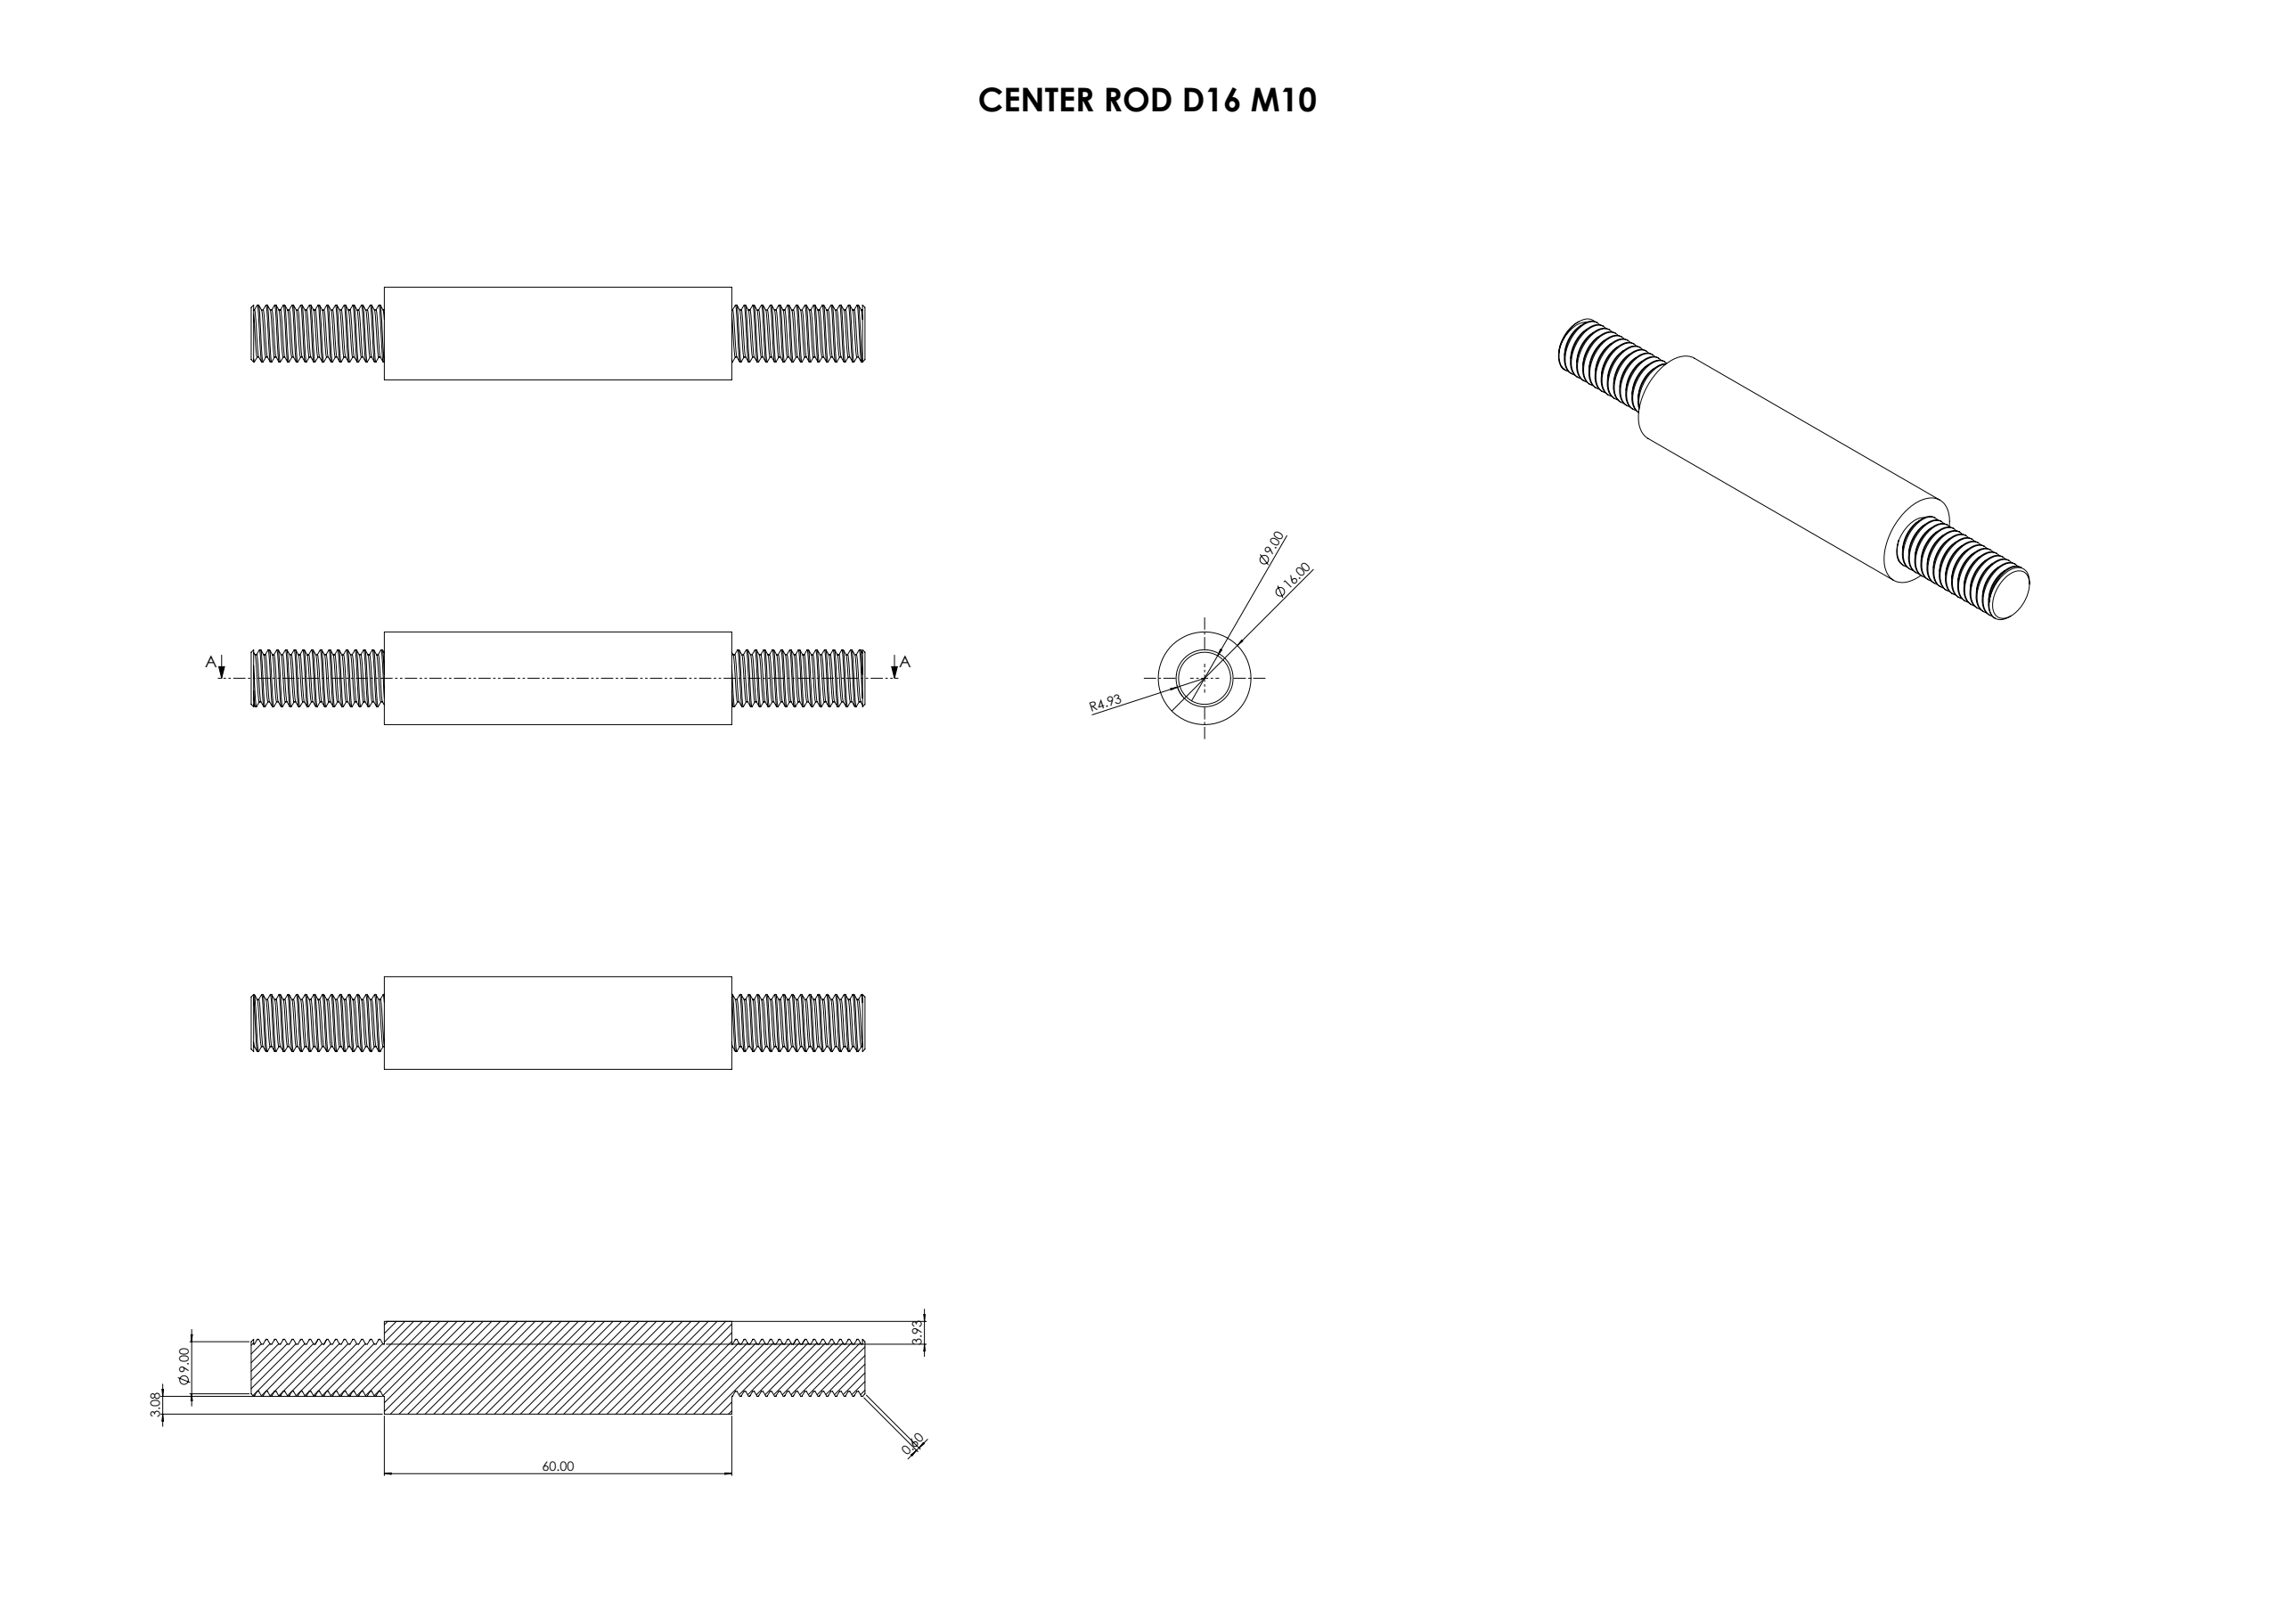
ISO-10303-21;
HEADER;
/* Generated by software containing ST-Developer
 * from STEP Tools, Inc. (www.steptools.com) 
 */

FILE_DESCRIPTION(
/* description */ (''),
/* implementation_level */ '2;1');

FILE_NAME(
/* name */ '08_Center_Rod_D16_M10.step',
/* time_stamp */ '2026-10-26T06:13:19-07:00',
/* author */ (''),
/* organization */ (''),
/* preprocessor_version */ 'ST-DEVELOPER v20.2',
/* originating_system */ 'Autodesk Translation Framework v15.15.0.0',
/* authorisation */ '');

FILE_SCHEMA (('AUTOMOTIVE_DESIGN { 1 0 10303 214 3 1 1 }','TECHNICAL_DATA_PACKAGING'));
ENDSEC;

DATA;
#10=MECHANICAL_DESIGN_GEOMETRIC_PRESENTATION_REPRESENTATION('',(#304),#56639);
#264=SHAPE_REPRESENTATION_RELATIONSHIP('SRR','None',#56752,#284);
#284=ADVANCED_BREP_SHAPE_REPRESENTATION('',(#324),#56626);
#304=STYLED_ITEM('',(#56915),#324);
#324=MANIFOLD_SOLID_BREP('Body1',#16956);
#339=B_SPLINE_SURFACE_WITH_KNOTS('',3,3,((#28895,#28896,#28897,#28898,#28899,
#28900,#28901,#28902,#28903,#28904,#28905,#28906,#28907,#28908,#28909,#28910,
#28911,#28912,#28913,#28914,#28915,#28916,#28917,#28918,#28919,#28920,#28921,
#28922,#28923,#28924,#28925,#28926,#28927,#28928,#28929,#28930,#28931,#28932,
#28933,#28934,#28935,#28936,#28937,#28938,#28939,#28940,#28941,#28942,#28943,
#28944,#28945,#28946,#28947,#28948,#28949,#28950,#28951,#28952,#28953,#28954,
#28955,#28956,#28957,#28958,#28959,#28960,#28961,#28962,#28963,#28964,#28965,
#28966,#28967,#28968,#28969,#28970,#28971,#28972,#28973,#28974,#28975,#28976,
#28977,#28978,#28979,#28980,#28981,#28982,#28983,#28984,#28985,#28986,#28987,
#28988,#28989,#28990,#28991,#28992,#28993,#28994,#28995,#28996,#28997,#28998,
#28999,#29000,#29001,#29002,#29003,#29004,#29005,#29006,#29007,#29008,#29009,
#29010,#29011,#29012,#29013,#29014,#29015,#29016,#29017,#29018,#29019,#29020,
#29021,#29022,#29023,#29024,#29025,#29026,#29027,#29028,#29029,#29030,#29031,
#29032,#29033,#29034,#29035,#29036,#29037,#29038,#29039,#29040,#29041,#29042,
#29043,#29044,#29045,#29046,#29047,#29048,#29049,#29050,#29051,#29052,#29053,
#29054,#29055,#29056,#29057,#29058,#29059,#29060,#29061,#29062,#29063,#29064,
#29065,#29066,#29067,#29068,#29069,#29070,#29071,#29072,#29073,#29074,#29075,
#29076,#29077,#29078,#29079,#29080,#29081,#29082,#29083,#29084,#29085,#29086,
#29087,#29088),(#29089,#29090,#29091,#29092,#29093,#29094,#29095,#29096,
#29097,#29098,#29099,#29100,#29101,#29102,#29103,#29104,#29105,#29106,#29107,
#29108,#29109,#29110,#29111,#29112,#29113,#29114,#29115,#29116,#29117,#29118,
#29119,#29120,#29121,#29122,#29123,#29124,#29125,#29126,#29127,#29128,#29129,
#29130,#29131,#29132,#29133,#29134,#29135,#29136,#29137,#29138,#29139,#29140,
#29141,#29142,#29143,#29144,#29145,#29146,#29147,#29148,#29149,#29150,#29151,
#29152,#29153,#29154,#29155,#29156,#29157,#29158,#29159,#29160,#29161,#29162,
#29163,#29164,#29165,#29166,#29167,#29168,#29169,#29170,#29171,#29172,#29173,
#29174,#29175,#29176,#29177,#29178,#29179,#29180,#29181,#29182,#29183,#29184,
#29185,#29186,#29187,#29188,#29189,#29190,#29191,#29192,#29193,#29194,#29195,
#29196,#29197,#29198,#29199,#29200,#29201,#29202,#29203,#29204,#29205,#29206,
#29207,#29208,#29209,#29210,#29211,#29212,#29213,#29214,#29215,#29216,#29217,
#29218,#29219,#29220,#29221,#29222,#29223,#29224,#29225,#29226,#29227,#29228,
#29229,#29230,#29231,#29232,#29233,#29234,#29235,#29236,#29237,#29238,#29239,
#29240,#29241,#29242,#29243,#29244,#29245,#29246,#29247,#29248,#29249,#29250,
#29251,#29252,#29253,#29254,#29255,#29256,#29257,#29258,#29259,#29260,#29261,
#29262,#29263,#29264,#29265,#29266,#29267,#29268,#29269,#29270,#29271,#29272,
#29273,#29274,#29275,#29276,#29277,#29278,#29279,#29280,#29281,#29282),
(#29283,#29284,#29285,#29286,#29287,#29288,#29289,#29290,#29291,#29292,
#29293,#29294,#29295,#29296,#29297,#29298,#29299,#29300,#29301,#29302,#29303,
#29304,#29305,#29306,#29307,#29308,#29309,#29310,#29311,#29312,#29313,#29314,
#29315,#29316,#29317,#29318,#29319,#29320,#29321,#29322,#29323,#29324,#29325,
#29326,#29327,#29328,#29329,#29330,#29331,#29332,#29333,#29334,#29335,#29336,
#29337,#29338,#29339,#29340,#29341,#29342,#29343,#29344,#29345,#29346,#29347,
#29348,#29349,#29350,#29351,#29352,#29353,#29354,#29355,#29356,#29357,#29358,
#29359,#29360,#29361,#29362,#29363,#29364,#29365,#29366,#29367,#29368,#29369,
#29370,#29371,#29372,#29373,#29374,#29375,#29376,#29377,#29378,#29379,#29380,
#29381,#29382,#29383,#29384,#29385,#29386,#29387,#29388,#29389,#29390,#29391,
#29392,#29393,#29394,#29395,#29396,#29397,#29398,#29399,#29400,#29401,#29402,
#29403,#29404,#29405,#29406,#29407,#29408,#29409,#29410,#29411,#29412,#29413,
#29414,#29415,#29416,#29417,#29418,#29419,#29420,#29421,#29422,#29423,#29424,
#29425,#29426,#29427,#29428,#29429,#29430,#29431,#29432,#29433,#29434,#29435,
#29436,#29437,#29438,#29439,#29440,#29441,#29442,#29443,#29444,#29445,#29446,
#29447,#29448,#29449,#29450,#29451,#29452,#29453,#29454,#29455,#29456,#29457,
#29458,#29459,#29460,#29461,#29462,#29463,#29464,#29465,#29466,#29467,#29468,
#29469,#29470,#29471,#29472,#29473,#29474,#29475,#29476),(#29477,#29478,
#29479,#29480,#29481,#29482,#29483,#29484,#29485,#29486,#29487,#29488,#29489,
#29490,#29491,#29492,#29493,#29494,#29495,#29496,#29497,#29498,#29499,#29500,
#29501,#29502,#29503,#29504,#29505,#29506,#29507,#29508,#29509,#29510,#29511,
#29512,#29513,#29514,#29515,#29516,#29517,#29518,#29519,#29520,#29521,#29522,
#29523,#29524,#29525,#29526,#29527,#29528,#29529,#29530,#29531,#29532,#29533,
#29534,#29535,#29536,#29537,#29538,#29539,#29540,#29541,#29542,#29543,#29544,
#29545,#29546,#29547,#29548,#29549,#29550,#29551,#29552,#29553,#29554,#29555,
#29556,#29557,#29558,#29559,#29560,#29561,#29562,#29563,#29564,#29565,#29566,
#29567,#29568,#29569,#29570,#29571,#29572,#29573,#29574,#29575,#29576,#29577,
#29578,#29579,#29580,#29581,#29582,#29583,#29584,#29585,#29586,#29587,#29588,
#29589,#29590,#29591,#29592,#29593,#29594,#29595,#29596,#29597,#29598,#29599,
#29600,#29601,#29602,#29603,#29604,#29605,#29606,#29607,#29608,#29609,#29610,
#29611,#29612,#29613,#29614,#29615,#29616,#29617,#29618,#29619,#29620,#29621,
#29622,#29623,#29624,#29625,#29626,#29627,#29628,#29629,#29630,#29631,#29632,
#29633,#29634,#29635,#29636,#29637,#29638,#29639,#29640,#29641,#29642,#29643,
#29644,#29645,#29646,#29647,#29648,#29649,#29650,#29651,#29652,#29653,#29654,
#29655,#29656,#29657,#29658,#29659,#29660,#29661,#29662,#29663,#29664,#29665,
#29666,#29667,#29668,#29669,#29670)),.UNSPECIFIED.,.F.,.F.,.F.,(4,4),(4,
1,1,1,1,1,1,1,1,1,1,1,1,1,1,1,1,1,1,1,1,1,1,1,1,1,1,1,1,1,1,1,1,1,1,1,1,
1,1,1,1,1,1,1,1,1,1,1,1,1,1,1,1,1,1,1,1,1,1,1,1,1,1,1,1,1,1,1,1,1,1,1,1,
1,1,1,1,1,1,1,1,1,1,1,1,1,1,1,1,1,1,1,1,1,1,1,1,1,1,1,1,1,1,1,1,1,1,1,1,
1,1,1,1,1,1,1,1,1,1,1,1,1,1,1,1,1,1,1,1,1,1,1,1,1,1,1,1,1,1,1,1,1,1,1,1,
1,1,1,1,1,1,1,1,1,1,1,1,1,1,1,1,1,1,1,1,1,1,1,1,1,1,1,1,1,1,1,1,1,1,1,1,
1,1,1,1,1,1,1,1,1,1,4),(0.,0.0986691610045069),(8.30989595155334,8.80798080180439,
9.30606565205544,9.80415050230649,10.3022353525575,10.8003202028086,11.2984050530596,
11.7964899033107,12.2945747535617,12.7926596038128,13.2907444540638,13.7888293043149,
14.2869141545659,14.784999004817,15.283083855068,15.7811687053191,16.2792535555701,
16.7773384058212,17.2754232560722,17.7735081063233,18.2715929565743,18.7696778068254,
19.2677626570764,19.7658475073275,20.2639323575785,20.7620172078296,21.2601020580806,
21.7581869083317,22.2562717585827,22.7543566088338,23.2524414590848,23.7505263093359,
24.2486111595869,24.746696009838,25.244780860089,25.7428657103401,26.2409505605911,
26.7390354108422,27.2371202610932,27.7352051113443,28.2332899615953,28.7313748118464,
29.2294596620974,29.7275445123485,30.2256293625995,30.7237142128506,31.2217990631016,
31.7198839133527,32.2179687636037,32.7160536138548,33.2141384641058,33.7122233143569,
34.2103081646079,34.708393014859,35.20647786511,35.7045627153611,36.2026475656121,
36.7007324158632,37.1988172661142,37.6969021163653,38.1949869666163,38.6930718168674,
39.1911566671184,39.6892415173695,40.1873263676205,40.6854112178715,41.1834960681226,
41.6815809183737,42.1796657686247,42.6777506188757,43.1758354691268,43.6739203193778,
44.1720051696289,44.67009001988,45.168174870131,45.666259720382,46.1643445706331,
46.6624294208841,47.1605142711352,47.6585991213862,48.1566839716373,48.6547688218883,
49.1528536721394,49.6509385223904,50.1490233726415,50.6471082228925,51.1451930731436,
51.6432779233946,52.1413627736457,52.6394476238967,53.1375324741478,53.6356173243988,
54.1337021746499,54.6317870249009,55.129871875152,56.1260415756541,57.1222112761562,
58.1183809766583,58.6164658269093,59.1145506771604,59.6126355274114,60.1107203776625,
60.6088052279135,61.1068900781646,61.6049749284156,62.1030597786667,62.6011446289177,
63.0992294791688,63.5973143294198,64.0953991796709,64.5934840299219,65.091568880173,
65.589653730424,66.0877385806751,66.5858234309261,67.0839082811772,67.5819931314282,
68.0800779816793,68.5781628319303,69.0762476821814,69.5743325324324,70.0724173826835,
70.5705022329345,71.0685870831856,71.5666719334366,72.0647567836877,72.5628416339387,
73.0609264841898,73.5590113344408,74.0570961846919,74.5551810349429,75.053265885194,
75.551350735445,76.0494355856961,76.5475204359471,77.0456052861982,77.5436901364492,
78.0417749867003,78.5398598369513,79.0379446872024,79.5360295374534,80.0341143877044,
80.5321992379555,81.0302840882066,81.5283689384576,82.0264537887087,82.5245386389597,
83.0226234892107,83.5207083394618,84.0187931897129,84.5168780399639,85.0149628902149,
85.513047740466,86.011132590717,86.5092174409681,87.0073022912191,87.5053871414702,
88.0034719917212,88.5015568419723,88.9996416922233,89.4977265424744,89.9958113927254,
90.4938962429765,90.9919810932275,91.4900659434786,91.9881507937296,92.4862356439807,
92.9843204942317,93.4824053444828,93.9804901947338,94.4785750449849,94.9766598952359,
95.474744745487,95.972829595738,96.4709144459891,96.9689992962401,97.4670841464912,
97.9651689967422,98.4632538469933,98.9613386972443,99.4594235474954,99.9575083977464,
100.455593247997,100.953678098249,101.4517629485,101.949847798751,102.447932649002,
102.946017499253,103.444102349504,103.942187199755,104.440272050006,104.938356900257),
 .UNSPECIFIED.);
#340=B_SPLINE_SURFACE_WITH_KNOTS('',3,3,((#29850,#29851,#29852,#29853,#29854,
#29855,#29856,#29857,#29858,#29859,#29860,#29861,#29862,#29863,#29864,#29865,
#29866,#29867,#29868,#29869,#29870,#29871,#29872,#29873,#29874,#29875,#29876,
#29877,#29878,#29879,#29880,#29881,#29882,#29883,#29884,#29885,#29886,#29887,
#29888,#29889,#29890,#29891,#29892,#29893,#29894,#29895,#29896,#29897,#29898,
#29899,#29900,#29901,#29902,#29903,#29904,#29905,#29906,#29907,#29908,#29909,
#29910,#29911,#29912,#29913,#29914,#29915,#29916,#29917,#29918,#29919,#29920,
#29921,#29922,#29923,#29924,#29925,#29926,#29927,#29928,#29929,#29930,#29931,
#29932,#29933,#29934,#29935,#29936,#29937,#29938,#29939,#29940,#29941,#29942,
#29943,#29944,#29945,#29946,#29947,#29948,#29949,#29950,#29951,#29952,#29953,
#29954,#29955,#29956,#29957,#29958,#29959,#29960,#29961,#29962,#29963,#29964,
#29965,#29966,#29967,#29968,#29969,#29970,#29971,#29972,#29973,#29974,#29975,
#29976,#29977,#29978,#29979,#29980,#29981,#29982,#29983,#29984,#29985,#29986,
#29987,#29988,#29989,#29990,#29991,#29992,#29993,#29994,#29995,#29996,#29997,
#29998,#29999,#30000,#30001,#30002,#30003,#30004,#30005,#30006,#30007,#30008,
#30009,#30010,#30011,#30012,#30013,#30014,#30015,#30016,#30017,#30018,#30019,
#30020,#30021,#30022,#30023,#30024,#30025,#30026,#30027,#30028,#30029,#30030,
#30031,#30032,#30033,#30034,#30035,#30036,#30037,#30038,#30039,#30040,#30041,
#30042,#30043),(#30044,#30045,#30046,#30047,#30048,#30049,#30050,#30051,
#30052,#30053,#30054,#30055,#30056,#30057,#30058,#30059,#30060,#30061,#30062,
#30063,#30064,#30065,#30066,#30067,#30068,#30069,#30070,#30071,#30072,#30073,
#30074,#30075,#30076,#30077,#30078,#30079,#30080,#30081,#30082,#30083,#30084,
#30085,#30086,#30087,#30088,#30089,#30090,#30091,#30092,#30093,#30094,#30095,
#30096,#30097,#30098,#30099,#30100,#30101,#30102,#30103,#30104,#30105,#30106,
#30107,#30108,#30109,#30110,#30111,#30112,#30113,#30114,#30115,#30116,#30117,
#30118,#30119,#30120,#30121,#30122,#30123,#30124,#30125,#30126,#30127,#30128,
#30129,#30130,#30131,#30132,#30133,#30134,#30135,#30136,#30137,#30138,#30139,
#30140,#30141,#30142,#30143,#30144,#30145,#30146,#30147,#30148,#30149,#30150,
#30151,#30152,#30153,#30154,#30155,#30156,#30157,#30158,#30159,#30160,#30161,
#30162,#30163,#30164,#30165,#30166,#30167,#30168,#30169,#30170,#30171,#30172,
#30173,#30174,#30175,#30176,#30177,#30178,#30179,#30180,#30181,#30182,#30183,
#30184,#30185,#30186,#30187,#30188,#30189,#30190,#30191,#30192,#30193,#30194,
#30195,#30196,#30197,#30198,#30199,#30200,#30201,#30202,#30203,#30204,#30205,
#30206,#30207,#30208,#30209,#30210,#30211,#30212,#30213,#30214,#30215,#30216,
#30217,#30218,#30219,#30220,#30221,#30222,#30223,#30224,#30225,#30226,#30227,
#30228,#30229,#30230,#30231,#30232,#30233,#30234,#30235,#30236,#30237),
(#30238,#30239,#30240,#30241,#30242,#30243,#30244,#30245,#30246,#30247,
#30248,#30249,#30250,#30251,#30252,#30253,#30254,#30255,#30256,#30257,#30258,
#30259,#30260,#30261,#30262,#30263,#30264,#30265,#30266,#30267,#30268,#30269,
#30270,#30271,#30272,#30273,#30274,#30275,#30276,#30277,#30278,#30279,#30280,
#30281,#30282,#30283,#30284,#30285,#30286,#30287,#30288,#30289,#30290,#30291,
#30292,#30293,#30294,#30295,#30296,#30297,#30298,#30299,#30300,#30301,#30302,
#30303,#30304,#30305,#30306,#30307,#30308,#30309,#30310,#30311,#30312,#30313,
#30314,#30315,#30316,#30317,#30318,#30319,#30320,#30321,#30322,#30323,#30324,
#30325,#30326,#30327,#30328,#30329,#30330,#30331,#30332,#30333,#30334,#30335,
#30336,#30337,#30338,#30339,#30340,#30341,#30342,#30343,#30344,#30345,#30346,
#30347,#30348,#30349,#30350,#30351,#30352,#30353,#30354,#30355,#30356,#30357,
#30358,#30359,#30360,#30361,#30362,#30363,#30364,#30365,#30366,#30367,#30368,
#30369,#30370,#30371,#30372,#30373,#30374,#30375,#30376,#30377,#30378,#30379,
#30380,#30381,#30382,#30383,#30384,#30385,#30386,#30387,#30388,#30389,#30390,
#30391,#30392,#30393,#30394,#30395,#30396,#30397,#30398,#30399,#30400,#30401,
#30402,#30403,#30404,#30405,#30406,#30407,#30408,#30409,#30410,#30411,#30412,
#30413,#30414,#30415,#30416,#30417,#30418,#30419,#30420,#30421,#30422,#30423,
#30424,#30425,#30426,#30427,#30428,#30429,#30430,#30431),(#30432,#30433,
#30434,#30435,#30436,#30437,#30438,#30439,#30440,#30441,#30442,#30443,#30444,
#30445,#30446,#30447,#30448,#30449,#30450,#30451,#30452,#30453,#30454,#30455,
#30456,#30457,#30458,#30459,#30460,#30461,#30462,#30463,#30464,#30465,#30466,
#30467,#30468,#30469,#30470,#30471,#30472,#30473,#30474,#30475,#30476,#30477,
#30478,#30479,#30480,#30481,#30482,#30483,#30484,#30485,#30486,#30487,#30488,
#30489,#30490,#30491,#30492,#30493,#30494,#30495,#30496,#30497,#30498,#30499,
#30500,#30501,#30502,#30503,#30504,#30505,#30506,#30507,#30508,#30509,#30510,
#30511,#30512,#30513,#30514,#30515,#30516,#30517,#30518,#30519,#30520,#30521,
#30522,#30523,#30524,#30525,#30526,#30527,#30528,#30529,#30530,#30531,#30532,
#30533,#30534,#30535,#30536,#30537,#30538,#30539,#30540,#30541,#30542,#30543,
#30544,#30545,#30546,#30547,#30548,#30549,#30550,#30551,#30552,#30553,#30554,
#30555,#30556,#30557,#30558,#30559,#30560,#30561,#30562,#30563,#30564,#30565,
#30566,#30567,#30568,#30569,#30570,#30571,#30572,#30573,#30574,#30575,#30576,
#30577,#30578,#30579,#30580,#30581,#30582,#30583,#30584,#30585,#30586,#30587,
#30588,#30589,#30590,#30591,#30592,#30593,#30594,#30595,#30596,#30597,#30598,
#30599,#30600,#30601,#30602,#30603,#30604,#30605,#30606,#30607,#30608,#30609,
#30610,#30611,#30612,#30613,#30614,#30615,#30616,#30617,#30618,#30619,#30620,
#30621,#30622,#30623,#30624,#30625)),.UNSPECIFIED.,.F.,.F.,.F.,(4,4),(4,
1,1,1,1,1,1,1,1,1,1,1,1,1,1,1,1,1,1,1,1,1,1,1,1,1,1,1,1,1,1,1,1,1,1,1,1,
1,1,1,1,1,1,1,1,1,1,1,1,1,1,1,1,1,1,1,1,1,1,1,1,1,1,1,1,1,1,1,1,1,1,1,1,
1,1,1,1,1,1,1,1,1,1,1,1,1,1,1,1,1,1,1,1,1,1,1,1,1,1,1,1,1,1,1,1,1,1,1,1,
1,1,1,1,1,1,1,1,1,1,1,1,1,1,1,1,1,1,1,1,1,1,1,1,1,1,1,1,1,1,1,1,1,1,1,1,
1,1,1,1,1,1,1,1,1,1,1,1,1,1,1,1,1,1,1,1,1,1,1,1,1,1,1,1,1,1,1,1,1,1,1,1,
1,1,1,1,1,1,1,1,1,1,4),(0.,0.0986691610045069),(11.6147305479242,12.1128153981753,
12.6109002484263,13.1089850986774,13.6070699489284,14.1051547991795,14.6032396494305,
15.1013244996816,15.5994093499326,16.0974942001837,16.5955790504347,17.0936639006858,
17.5917487509368,18.0898336011878,18.5879184514389,19.0860033016899,19.584088151941,
20.082173002192,20.5802578524431,21.0783427026941,21.5764275529452,22.0745124031962,
22.5725972534473,23.0706821036983,23.5687669539494,24.0668518042004,24.5649366544515,
25.0630215047025,25.5611063549536,26.0591912052046,26.5572760554557,27.0553609057067,
27.5534457559578,28.0515306062088,28.5496154564599,29.0477003067109,29.545785156962,
30.043870007213,30.5419548574641,31.0400397077151,31.5381245579662,32.0362094082172,
32.5342942584683,33.0323791087193,33.5304639589704,34.0285488092214,34.5266336594725,
35.0247185097235,35.5228033599746,36.0208882102256,36.5189730604767,37.0170579107277,
37.5151427609788,38.0132276112298,38.5113124614809,39.0093973117319,39.507482161983,
40.005567012234,40.5036518624851,41.0017367127361,41.4998215629872,41.9979064132382,
42.4959912634893,42.9940761137403,43.4921609639914,43.9902458142424,44.4883306644935,
44.9864155147445,45.4845003649956,45.9825852152466,46.4806700654977,46.9787549157487,
47.4768397659998,47.9749246162508,48.4730094665019,48.9710943167529,49.469179167004,
49.967264017255,50.4653488675061,50.9634337177571,51.4615185680082,51.9596034182592,
52.4576882685103,52.9557731187613,53.4538579690124,53.9519428192634,54.4500276695145,
54.9481125197655,55.4461973700166,55.9442822202676,56.4423670705187,56.9404519207697,
57.4385367710208,57.9366216212718,58.4347064715229,59.430876172025,60.427045872527,
61.4232155730292,61.9213004232802,62.4193852735312,62.9174701237823,63.4155549740333,
63.9136398242844,64.4117246745354,64.9098095247865,65.4078943750375,65.9059792252886,
66.4040640755397,66.9021489257907,67.4002337760417,67.8983186262928,68.3964034765438,
68.8944883267949,69.3925731770459,69.890658027297,70.388742877548,70.8868277277991,
71.3849125780501,71.8829974283012,72.3810822785522,72.8791671288033,73.3772519790543,
73.8753368293054,74.3734216795564,74.8715065298075,75.3695913800585,75.8676762303096,
76.3657610805606,76.8638459308117,77.3619307810627,77.8600156313138,78.3581004815648,
78.8561853318159,79.3542701820669,79.852355032318,80.350439882569,80.8485247328201,
81.3466095830711,81.8446944333222,82.3427792835732,82.8408641338243,83.3389489840753,
83.8370338343264,84.3351186845774,84.8332035348285,85.3312883850795,85.8293732353306,
86.3274580855816,86.8255429358327,87.3236277860837,87.8217126363348,88.3197974865858,
88.8178823368369,89.3159671870879,89.814052037339,90.31213688759,90.8102217378411,
91.3083065880921,91.8063914383432,92.3044762885942,92.8025611388453,93.3006459890963,
93.7987308393474,94.2968156895984,94.7949005398495,95.2929853901005,95.7910702403516,
96.2891550906026,96.7872399408537,97.2853247911047,97.7834096413558,98.2814944916068,
98.7795793418579,99.2776641921089,99.77574904236,100.273833892611,100.771918742862,
101.270003593113,101.768088443364,102.266173293615,102.764258143866,103.262342994117,
103.760427844368,104.258512694619,104.75659754487,105.254682395122,105.752767245373,
106.250852095624,106.748936945875,107.247021796126,107.745106646377,108.243191496628),
 .UNSPECIFIED.);
#341=B_SPLINE_SURFACE_WITH_KNOTS('',3,3,((#30768,#30769,#30770,#30771,#30772,
#30773,#30774,#30775,#30776,#30777,#30778,#30779,#30780,#30781,#30782,#30783,
#30784,#30785,#30786,#30787,#30788,#30789,#30790,#30791,#30792,#30793,#30794,
#30795,#30796,#30797,#30798,#30799,#30800,#30801,#30802,#30803,#30804,#30805,
#30806,#30807,#30808,#30809,#30810,#30811,#30812,#30813,#30814,#30815,#30816,
#30817,#30818,#30819,#30820,#30821,#30822,#30823,#30824,#30825,#30826,#30827,
#30828,#30829,#30830,#30831,#30832,#30833,#30834,#30835,#30836,#30837,#30838,
#30839,#30840,#30841,#30842,#30843,#30844,#30845,#30846,#30847,#30848,#30849,
#30850,#30851,#30852,#30853,#30854,#30855,#30856,#30857,#30858,#30859,#30860,
#30861,#30862,#30863,#30864,#30865,#30866,#30867,#30868,#30869,#30870,#30871,
#30872,#30873,#30874,#30875,#30876,#30877,#30878,#30879,#30880,#30881,#30882,
#30883,#30884,#30885,#30886,#30887,#30888,#30889,#30890,#30891,#30892,#30893,
#30894,#30895,#30896,#30897,#30898,#30899,#30900,#30901,#30902,#30903,#30904,
#30905,#30906,#30907,#30908,#30909,#30910,#30911,#30912,#30913,#30914,#30915,
#30916,#30917,#30918,#30919,#30920,#30921,#30922,#30923,#30924,#30925,#30926,
#30927,#30928,#30929,#30930,#30931,#30932,#30933,#30934,#30935,#30936,#30937,
#30938,#30939,#30940,#30941,#30942,#30943,#30944,#30945,#30946,#30947,#30948,
#30949,#30950,#30951,#30952,#30953,#30954,#30955,#30956,#30957,#30958,#30959,
#30960,#30961),(#30962,#30963,#30964,#30965,#30966,#30967,#30968,#30969,
#30970,#30971,#30972,#30973,#30974,#30975,#30976,#30977,#30978,#30979,#30980,
#30981,#30982,#30983,#30984,#30985,#30986,#30987,#30988,#30989,#30990,#30991,
#30992,#30993,#30994,#30995,#30996,#30997,#30998,#30999,#31000,#31001,#31002,
#31003,#31004,#31005,#31006,#31007,#31008,#31009,#31010,#31011,#31012,#31013,
#31014,#31015,#31016,#31017,#31018,#31019,#31020,#31021,#31022,#31023,#31024,
#31025,#31026,#31027,#31028,#31029,#31030,#31031,#31032,#31033,#31034,#31035,
#31036,#31037,#31038,#31039,#31040,#31041,#31042,#31043,#31044,#31045,#31046,
#31047,#31048,#31049,#31050,#31051,#31052,#31053,#31054,#31055,#31056,#31057,
#31058,#31059,#31060,#31061,#31062,#31063,#31064,#31065,#31066,#31067,#31068,
#31069,#31070,#31071,#31072,#31073,#31074,#31075,#31076,#31077,#31078,#31079,
#31080,#31081,#31082,#31083,#31084,#31085,#31086,#31087,#31088,#31089,#31090,
#31091,#31092,#31093,#31094,#31095,#31096,#31097,#31098,#31099,#31100,#31101,
#31102,#31103,#31104,#31105,#31106,#31107,#31108,#31109,#31110,#31111,#31112,
#31113,#31114,#31115,#31116,#31117,#31118,#31119,#31120,#31121,#31122,#31123,
#31124,#31125,#31126,#31127,#31128,#31129,#31130,#31131,#31132,#31133,#31134,
#31135,#31136,#31137,#31138,#31139,#31140,#31141,#31142,#31143,#31144,#31145,
#31146,#31147,#31148,#31149,#31150,#31151,#31152,#31153,#31154,#31155),
(#31156,#31157,#31158,#31159,#31160,#31161,#31162,#31163,#31164,#31165,
#31166,#31167,#31168,#31169,#31170,#31171,#31172,#31173,#31174,#31175,#31176,
#31177,#31178,#31179,#31180,#31181,#31182,#31183,#31184,#31185,#31186,#31187,
#31188,#31189,#31190,#31191,#31192,#31193,#31194,#31195,#31196,#31197,#31198,
#31199,#31200,#31201,#31202,#31203,#31204,#31205,#31206,#31207,#31208,#31209,
#31210,#31211,#31212,#31213,#31214,#31215,#31216,#31217,#31218,#31219,#31220,
#31221,#31222,#31223,#31224,#31225,#31226,#31227,#31228,#31229,#31230,#31231,
#31232,#31233,#31234,#31235,#31236,#31237,#31238,#31239,#31240,#31241,#31242,
#31243,#31244,#31245,#31246,#31247,#31248,#31249,#31250,#31251,#31252,#31253,
#31254,#31255,#31256,#31257,#31258,#31259,#31260,#31261,#31262,#31263,#31264,
#31265,#31266,#31267,#31268,#31269,#31270,#31271,#31272,#31273,#31274,#31275,
#31276,#31277,#31278,#31279,#31280,#31281,#31282,#31283,#31284,#31285,#31286,
#31287,#31288,#31289,#31290,#31291,#31292,#31293,#31294,#31295,#31296,#31297,
#31298,#31299,#31300,#31301,#31302,#31303,#31304,#31305,#31306,#31307,#31308,
#31309,#31310,#31311,#31312,#31313,#31314,#31315,#31316,#31317,#31318,#31319,
#31320,#31321,#31322,#31323,#31324,#31325,#31326,#31327,#31328,#31329,#31330,
#31331,#31332,#31333,#31334,#31335,#31336,#31337,#31338,#31339,#31340,#31341,
#31342,#31343,#31344,#31345,#31346,#31347,#31348,#31349),(#31350,#31351,
#31352,#31353,#31354,#31355,#31356,#31357,#31358,#31359,#31360,#31361,#31362,
#31363,#31364,#31365,#31366,#31367,#31368,#31369,#31370,#31371,#31372,#31373,
#31374,#31375,#31376,#31377,#31378,#31379,#31380,#31381,#31382,#31383,#31384,
#31385,#31386,#31387,#31388,#31389,#31390,#31391,#31392,#31393,#31394,#31395,
#31396,#31397,#31398,#31399,#31400,#31401,#31402,#31403,#31404,#31405,#31406,
#31407,#31408,#31409,#31410,#31411,#31412,#31413,#31414,#31415,#31416,#31417,
#31418,#31419,#31420,#31421,#31422,#31423,#31424,#31425,#31426,#31427,#31428,
#31429,#31430,#31431,#31432,#31433,#31434,#31435,#31436,#31437,#31438,#31439,
#31440,#31441,#31442,#31443,#31444,#31445,#31446,#31447,#31448,#31449,#31450,
#31451,#31452,#31453,#31454,#31455,#31456,#31457,#31458,#31459,#31460,#31461,
#31462,#31463,#31464,#31465,#31466,#31467,#31468,#31469,#31470,#31471,#31472,
#31473,#31474,#31475,#31476,#31477,#31478,#31479,#31480,#31481,#31482,#31483,
#31484,#31485,#31486,#31487,#31488,#31489,#31490,#31491,#31492,#31493,#31494,
#31495,#31496,#31497,#31498,#31499,#31500,#31501,#31502,#31503,#31504,#31505,
#31506,#31507,#31508,#31509,#31510,#31511,#31512,#31513,#31514,#31515,#31516,
#31517,#31518,#31519,#31520,#31521,#31522,#31523,#31524,#31525,#31526,#31527,
#31528,#31529,#31530,#31531,#31532,#31533,#31534,#31535,#31536,#31537,#31538,
#31539,#31540,#31541,#31542,#31543)),.UNSPECIFIED.,.F.,.F.,.F.,(4,4),(4,
1,1,1,1,1,1,1,1,1,1,1,1,1,1,1,1,1,1,1,1,1,1,1,1,1,1,1,1,1,1,1,1,1,1,1,1,
1,1,1,1,1,1,1,1,1,1,1,1,1,1,1,1,1,1,1,1,1,1,1,1,1,1,1,1,1,1,1,1,1,1,1,1,
1,1,1,1,1,1,1,1,1,1,1,1,1,1,1,1,1,1,1,1,1,1,1,1,1,1,1,1,1,1,1,1,1,1,1,1,
1,1,1,1,1,1,1,1,1,1,1,1,1,1,1,1,1,1,1,1,1,1,1,1,1,1,1,1,1,1,1,1,1,1,1,1,
1,1,1,1,1,1,1,1,1,1,1,1,1,1,1,1,1,1,1,1,1,1,1,1,1,1,1,1,1,1,1,1,1,1,1,1,
1,1,1,1,1,1,1,1,1,1,4),(0.,0.0986691610045069),(8.30989595155336,8.80798080180441,
9.30606565205546,9.80415050230651,10.3022353525576,10.8003202028086,11.2984050530597,
11.7964899033107,12.2945747535618,12.7926596038128,13.2907444540639,13.7888293043149,
14.286914154566,14.784999004817,15.2830838550681,15.7811687053191,16.2792535555702,
16.7773384058212,17.2754232560723,17.7735081063233,18.2715929565744,18.7696778068254,
19.2677626570764,19.7658475073275,20.2639323575785,20.7620172078296,21.2601020580806,
21.7581869083317,22.2562717585827,22.7543566088338,23.2524414590848,23.7505263093359,
24.2486111595869,24.746696009838,25.244780860089,25.7428657103401,26.2409505605911,
26.7390354108422,27.2371202610932,27.7352051113443,28.2332899615953,28.7313748118464,
29.2294596620974,29.7275445123485,30.2256293625995,30.7237142128506,31.2217990631016,
31.7198839133527,32.2179687636037,32.7160536138548,33.2141384641058,33.7122233143569,
34.2103081646079,34.708393014859,35.20647786511,35.7045627153611,36.2026475656121,
36.7007324158632,37.1988172661142,37.6969021163653,38.1949869666163,38.6930718168674,
39.1911566671184,39.6892415173695,40.1873263676205,40.6854112178716,41.1834960681226,
41.6815809183737,42.1796657686247,42.6777506188758,43.1758354691268,43.6739203193779,
44.1720051696289,44.67009001988,45.168174870131,45.6662597203821,46.1643445706331,
46.6624294208842,47.1605142711352,47.6585991213863,48.1566839716373,48.6547688218884,
49.1528536721394,49.6509385223905,50.1490233726415,50.6471082228926,51.1451930731436,
51.6432779233947,52.1413627736457,52.6394476238968,53.1375324741478,53.6356173243989,
54.1337021746499,54.631787024901,55.129871875152,56.1260415756541,57.1222112761562,
58.1183809766583,58.6164658269093,59.1145506771604,59.6126355274115,60.1107203776625,
60.6088052279135,61.1068900781646,61.6049749284156,62.1030597786667,62.6011446289178,
63.0992294791688,63.5973143294198,64.0953991796709,64.5934840299219,65.091568880173,
65.589653730424,66.0877385806751,66.5858234309261,67.0839082811772,67.5819931314282,
68.0800779816793,68.5781628319303,69.0762476821814,69.5743325324324,70.0724173826835,
70.5705022329345,71.0685870831856,71.5666719334366,72.0647567836877,72.5628416339387,
73.0609264841898,73.5590113344408,74.0570961846919,74.5551810349429,75.053265885194,
75.551350735445,76.0494355856961,76.5475204359471,77.0456052861982,77.5436901364492,
78.0417749867003,78.5398598369513,79.0379446872024,79.5360295374534,80.0341143877045,
80.5321992379555,81.0302840882066,81.5283689384576,82.0264537887087,82.5245386389597,
83.0226234892108,83.5207083394618,84.0187931897129,84.5168780399639,85.014962890215,
85.513047740466,86.0111325907171,86.5092174409681,87.0073022912192,87.5053871414702,
88.0034719917213,88.5015568419723,88.9996416922233,89.4977265424744,89.9958113927255,
90.4938962429765,90.9919810932276,91.4900659434786,91.9881507937297,92.4862356439807,
92.9843204942318,93.4824053444828,93.9804901947338,94.4785750449849,94.976659895236,
95.474744745487,95.972829595738,96.4709144459891,96.9689992962401,97.4670841464912,
97.9651689967422,98.4632538469933,98.9613386972443,99.4594235474954,99.9575083977464,
100.455593247997,100.953678098249,101.4517629485,101.949847798751,102.447932649002,
102.946017499253,103.444102349504,103.942187199755,104.440272050006,104.938356900257),
 .UNSPECIFIED.);
#342=B_SPLINE_SURFACE_WITH_KNOTS('',3,3,((#31946,#31947,#31948,#31949,#31950,
#31951,#31952,#31953,#31954,#31955,#31956,#31957,#31958,#31959,#31960,#31961,
#31962,#31963,#31964,#31965,#31966,#31967,#31968,#31969,#31970,#31971,#31972,
#31973,#31974,#31975,#31976,#31977,#31978,#31979,#31980,#31981,#31982,#31983,
#31984,#31985,#31986,#31987,#31988,#31989,#31990,#31991,#31992,#31993,#31994,
#31995,#31996,#31997,#31998,#31999,#32000,#32001,#32002,#32003,#32004,#32005,
#32006,#32007,#32008,#32009,#32010,#32011,#32012,#32013,#32014,#32015,#32016,
#32017,#32018,#32019,#32020,#32021,#32022,#32023,#32024,#32025,#32026,#32027,
#32028,#32029,#32030,#32031,#32032,#32033,#32034,#32035,#32036,#32037,#32038,
#32039,#32040,#32041,#32042,#32043,#32044,#32045,#32046,#32047,#32048,#32049,
#32050,#32051,#32052,#32053,#32054,#32055,#32056,#32057,#32058,#32059,#32060,
#32061,#32062,#32063,#32064,#32065,#32066,#32067,#32068,#32069,#32070,#32071,
#32072,#32073,#32074,#32075,#32076,#32077,#32078,#32079,#32080,#32081,#32082,
#32083,#32084,#32085,#32086,#32087,#32088,#32089,#32090,#32091,#32092,#32093,
#32094,#32095,#32096,#32097,#32098,#32099,#32100,#32101,#32102,#32103,#32104,
#32105,#32106,#32107,#32108,#32109,#32110,#32111,#32112,#32113,#32114,#32115,
#32116,#32117,#32118,#32119,#32120,#32121,#32122,#32123,#32124,#32125,#32126,
#32127,#32128,#32129,#32130,#32131,#32132,#32133,#32134,#32135,#32136,#32137,
#32138,#32139),(#32140,#32141,#32142,#32143,#32144,#32145,#32146,#32147,
#32148,#32149,#32150,#32151,#32152,#32153,#32154,#32155,#32156,#32157,#32158,
#32159,#32160,#32161,#32162,#32163,#32164,#32165,#32166,#32167,#32168,#32169,
#32170,#32171,#32172,#32173,#32174,#32175,#32176,#32177,#32178,#32179,#32180,
#32181,#32182,#32183,#32184,#32185,#32186,#32187,#32188,#32189,#32190,#32191,
#32192,#32193,#32194,#32195,#32196,#32197,#32198,#32199,#32200,#32201,#32202,
#32203,#32204,#32205,#32206,#32207,#32208,#32209,#32210,#32211,#32212,#32213,
#32214,#32215,#32216,#32217,#32218,#32219,#32220,#32221,#32222,#32223,#32224,
#32225,#32226,#32227,#32228,#32229,#32230,#32231,#32232,#32233,#32234,#32235,
#32236,#32237,#32238,#32239,#32240,#32241,#32242,#32243,#32244,#32245,#32246,
#32247,#32248,#32249,#32250,#32251,#32252,#32253,#32254,#32255,#32256,#32257,
#32258,#32259,#32260,#32261,#32262,#32263,#32264,#32265,#32266,#32267,#32268,
#32269,#32270,#32271,#32272,#32273,#32274,#32275,#32276,#32277,#32278,#32279,
#32280,#32281,#32282,#32283,#32284,#32285,#32286,#32287,#32288,#32289,#32290,
#32291,#32292,#32293,#32294,#32295,#32296,#32297,#32298,#32299,#32300,#32301,
#32302,#32303,#32304,#32305,#32306,#32307,#32308,#32309,#32310,#32311,#32312,
#32313,#32314,#32315,#32316,#32317,#32318,#32319,#32320,#32321,#32322,#32323,
#32324,#32325,#32326,#32327,#32328,#32329,#32330,#32331,#32332,#32333),
(#32334,#32335,#32336,#32337,#32338,#32339,#32340,#32341,#32342,#32343,
#32344,#32345,#32346,#32347,#32348,#32349,#32350,#32351,#32352,#32353,#32354,
#32355,#32356,#32357,#32358,#32359,#32360,#32361,#32362,#32363,#32364,#32365,
#32366,#32367,#32368,#32369,#32370,#32371,#32372,#32373,#32374,#32375,#32376,
#32377,#32378,#32379,#32380,#32381,#32382,#32383,#32384,#32385,#32386,#32387,
#32388,#32389,#32390,#32391,#32392,#32393,#32394,#32395,#32396,#32397,#32398,
#32399,#32400,#32401,#32402,#32403,#32404,#32405,#32406,#32407,#32408,#32409,
#32410,#32411,#32412,#32413,#32414,#32415,#32416,#32417,#32418,#32419,#32420,
#32421,#32422,#32423,#32424,#32425,#32426,#32427,#32428,#32429,#32430,#32431,
#32432,#32433,#32434,#32435,#32436,#32437,#32438,#32439,#32440,#32441,#32442,
#32443,#32444,#32445,#32446,#32447,#32448,#32449,#32450,#32451,#32452,#32453,
#32454,#32455,#32456,#32457,#32458,#32459,#32460,#32461,#32462,#32463,#32464,
#32465,#32466,#32467,#32468,#32469,#32470,#32471,#32472,#32473,#32474,#32475,
#32476,#32477,#32478,#32479,#32480,#32481,#32482,#32483,#32484,#32485,#32486,
#32487,#32488,#32489,#32490,#32491,#32492,#32493,#32494,#32495,#32496,#32497,
#32498,#32499,#32500,#32501,#32502,#32503,#32504,#32505,#32506,#32507,#32508,
#32509,#32510,#32511,#32512,#32513,#32514,#32515,#32516,#32517,#32518,#32519,
#32520,#32521,#32522,#32523,#32524,#32525,#32526,#32527),(#32528,#32529,
#32530,#32531,#32532,#32533,#32534,#32535,#32536,#32537,#32538,#32539,#32540,
#32541,#32542,#32543,#32544,#32545,#32546,#32547,#32548,#32549,#32550,#32551,
#32552,#32553,#32554,#32555,#32556,#32557,#32558,#32559,#32560,#32561,#32562,
#32563,#32564,#32565,#32566,#32567,#32568,#32569,#32570,#32571,#32572,#32573,
#32574,#32575,#32576,#32577,#32578,#32579,#32580,#32581,#32582,#32583,#32584,
#32585,#32586,#32587,#32588,#32589,#32590,#32591,#32592,#32593,#32594,#32595,
#32596,#32597,#32598,#32599,#32600,#32601,#32602,#32603,#32604,#32605,#32606,
#32607,#32608,#32609,#32610,#32611,#32612,#32613,#32614,#32615,#32616,#32617,
#32618,#32619,#32620,#32621,#32622,#32623,#32624,#32625,#32626,#32627,#32628,
#32629,#32630,#32631,#32632,#32633,#32634,#32635,#32636,#32637,#32638,#32639,
#32640,#32641,#32642,#32643,#32644,#32645,#32646,#32647,#32648,#32649,#32650,
#32651,#32652,#32653,#32654,#32655,#32656,#32657,#32658,#32659,#32660,#32661,
#32662,#32663,#32664,#32665,#32666,#32667,#32668,#32669,#32670,#32671,#32672,
#32673,#32674,#32675,#32676,#32677,#32678,#32679,#32680,#32681,#32682,#32683,
#32684,#32685,#32686,#32687,#32688,#32689,#32690,#32691,#32692,#32693,#32694,
#32695,#32696,#32697,#32698,#32699,#32700,#32701,#32702,#32703,#32704,#32705,
#32706,#32707,#32708,#32709,#32710,#32711,#32712,#32713,#32714,#32715,#32716,
#32717,#32718,#32719,#32720,#32721)),.UNSPECIFIED.,.F.,.F.,.F.,(4,4),(4,
1,1,1,1,1,1,1,1,1,1,1,1,1,1,1,1,1,1,1,1,1,1,1,1,1,1,1,1,1,1,1,1,1,1,1,1,
1,1,1,1,1,1,1,1,1,1,1,1,1,1,1,1,1,1,1,1,1,1,1,1,1,1,1,1,1,1,1,1,1,1,1,1,
1,1,1,1,1,1,1,1,1,1,1,1,1,1,1,1,1,1,1,1,1,1,1,1,1,1,1,1,1,1,1,1,1,1,1,1,
1,1,1,1,1,1,1,1,1,1,1,1,1,1,1,1,1,1,1,1,1,1,1,1,1,1,1,1,1,1,1,1,1,1,1,1,
1,1,1,1,1,1,1,1,1,1,1,1,1,1,1,1,1,1,1,1,1,1,1,1,1,1,1,1,1,1,1,1,1,1,1,1,
1,1,1,1,1,1,1,1,1,1,4),(0.,0.0986691610045069),(11.6147305479242,12.1128153981753,
12.6109002484263,13.1089850986774,13.6070699489284,14.1051547991795,14.6032396494305,
15.1013244996816,15.5994093499326,16.0974942001837,16.5955790504347,17.0936639006858,
17.5917487509368,18.0898336011879,18.5879184514389,19.08600330169,19.584088151941,
20.0821730021921,20.5802578524431,21.0783427026942,21.5764275529452,22.0745124031963,
22.5725972534473,23.0706821036984,23.5687669539494,24.0668518042005,24.5649366544515,
25.0630215047026,25.5611063549536,26.0591912052047,26.5572760554557,27.0553609057068,
27.5534457559578,28.0515306062089,28.5496154564599,29.047700306711,29.545785156962,
30.0438700072131,30.5419548574641,31.0400397077152,31.5381245579662,32.0362094082173,
32.5342942584683,33.0323791087194,33.5304639589704,34.0285488092214,34.5266336594725,
35.0247185097235,35.5228033599746,36.0208882102256,36.5189730604767,37.0170579107277,
37.5151427609788,38.0132276112299,38.5113124614809,39.0093973117319,39.507482161983,
40.005567012234,40.5036518624851,41.0017367127361,41.4998215629872,41.9979064132382,
42.4959912634893,42.9940761137403,43.4921609639914,43.9902458142424,44.4883306644935,
44.9864155147445,45.4845003649956,45.9825852152466,46.4806700654977,46.9787549157487,
47.4768397659998,47.9749246162508,48.4730094665019,48.9710943167529,49.469179167004,
49.967264017255,50.4653488675061,50.9634337177571,51.4615185680082,51.9596034182592,
52.4576882685103,52.9557731187613,53.4538579690124,53.9519428192634,54.4500276695145,
54.9481125197655,55.4461973700166,55.9442822202676,56.4423670705187,56.9404519207697,
57.4385367710208,57.9366216212718,58.4347064715229,59.430876172025,60.4270458725271,
61.4232155730292,61.9213004232802,62.4193852735313,62.9174701237823,63.4155549740334,
63.9136398242844,64.4117246745355,64.9098095247865,65.4078943750376,65.9059792252886,
66.4040640755397,66.9021489257907,67.4002337760418,67.8983186262928,68.3964034765439,
68.8944883267949,69.392573177046,69.890658027297,70.3887428775481,70.8868277277991,
71.3849125780502,71.8829974283012,72.3810822785523,72.8791671288033,73.3772519790544,
73.8753368293054,74.3734216795565,74.8715065298075,75.3695913800586,75.8676762303096,
76.3657610805606,76.8638459308117,77.3619307810628,77.8600156313138,78.3581004815648,
78.8561853318159,79.3542701820669,79.852355032318,80.350439882569,80.8485247328201,
81.3466095830711,81.8446944333222,82.3427792835733,82.8408641338243,83.3389489840753,
83.8370338343264,84.3351186845774,84.8332035348285,85.3312883850795,85.8293732353306,
86.3274580855816,86.8255429358327,87.3236277860837,87.8217126363348,88.3197974865858,
88.8178823368369,89.3159671870879,89.814052037339,90.31213688759,90.8102217378411,
91.3083065880921,91.8063914383432,92.3044762885942,92.8025611388453,93.3006459890963,
93.7987308393474,94.2968156895984,94.7949005398495,95.2929853901005,95.7910702403516,
96.2891550906026,96.7872399408537,97.2853247911047,97.7834096413558,98.2814944916068,
98.7795793418579,99.2776641921089,99.77574904236,100.273833892611,100.771918742862,
101.270003593113,101.768088443364,102.266173293615,102.764258143866,103.262342994117,
103.760427844368,104.258512694619,104.75659754487,105.254682395122,105.752767245373,
106.250852095624,106.748936945875,107.247021796126,107.745106646377,108.243191496628),
 .UNSPECIFIED.);
#510=FACE_BOUND('',#3171,.T.);
#511=FACE_BOUND('',#3174,.T.);
#595=CONICAL_SURFACE('',#17763,4.75,0.78539816339745);
#596=CONICAL_SURFACE('',#17771,4.75,0.78539816339745);
#926=CIRCLE('',#17686,4.925);
#927=CIRCLE('',#17702,4.0705);
#928=CIRCLE('',#17718,4.925);
#929=CIRCLE('',#17734,4.0705);
#930=CIRCLE('',#17750,4.925);
#931=CIRCLE('',#17751,4.925);
#932=CIRCLE('',#17753,4.0705);
#933=CIRCLE('',#17755,4.925);
#934=CIRCLE('',#17757,4.925);
#935=CIRCLE('',#17758,4.925);
#936=CIRCLE('',#17759,4.0705);
#937=CIRCLE('',#17762,4.5);
#938=CIRCLE('',#17765,4.925);
#939=CIRCLE('',#17767,8.);
#940=CIRCLE('',#17769,8.);
#941=CIRCLE('',#17772,4.5);
#1321=CYLINDRICAL_SURFACE('',#17685,4.925);
#1322=CYLINDRICAL_SURFACE('',#17687,4.925);
#1323=CYLINDRICAL_SURFACE('',#17688,4.925);
#1324=CYLINDRICAL_SURFACE('',#17689,4.925);
#1325=CYLINDRICAL_SURFACE('',#17690,4.925);
#1326=CYLINDRICAL_SURFACE('',#17691,4.925);
#1327=CYLINDRICAL_SURFACE('',#17692,4.925);
#1328=CYLINDRICAL_SURFACE('',#17693,4.925);
#1329=CYLINDRICAL_SURFACE('',#17694,4.925);
#1330=CYLINDRICAL_SURFACE('',#17695,4.925);
#1331=CYLINDRICAL_SURFACE('',#17696,4.925);
#1332=CYLINDRICAL_SURFACE('',#17697,4.925);
#1333=CYLINDRICAL_SURFACE('',#17698,4.925);
#1334=CYLINDRICAL_SURFACE('',#17699,4.925);
#1335=CYLINDRICAL_SURFACE('',#17700,4.925);
#1336=CYLINDRICAL_SURFACE('',#17701,4.0705);
#1337=CYLINDRICAL_SURFACE('',#17703,4.0705);
#1338=CYLINDRICAL_SURFACE('',#17704,4.0705);
#1339=CYLINDRICAL_SURFACE('',#17705,4.0705);
#1340=CYLINDRICAL_SURFACE('',#17706,4.0705);
#1341=CYLINDRICAL_SURFACE('',#17707,4.0705);
#1342=CYLINDRICAL_SURFACE('',#17708,4.0705);
#1343=CYLINDRICAL_SURFACE('',#17709,4.0705);
#1344=CYLINDRICAL_SURFACE('',#17710,4.0705);
#1345=CYLINDRICAL_SURFACE('',#17711,4.0705);
#1346=CYLINDRICAL_SURFACE('',#17712,4.0705);
#1347=CYLINDRICAL_SURFACE('',#17713,4.0705);
#1348=CYLINDRICAL_SURFACE('',#17714,4.0705);
#1349=CYLINDRICAL_SURFACE('',#17715,4.0705);
#1350=CYLINDRICAL_SURFACE('',#17716,4.0705);
#1351=CYLINDRICAL_SURFACE('',#17717,4.925);
#1352=CYLINDRICAL_SURFACE('',#17719,4.925);
#1353=CYLINDRICAL_SURFACE('',#17720,4.925);
#1354=CYLINDRICAL_SURFACE('',#17721,4.925);
#1355=CYLINDRICAL_SURFACE('',#17722,4.925);
#1356=CYLINDRICAL_SURFACE('',#17723,4.925);
#1357=CYLINDRICAL_SURFACE('',#17724,4.925);
#1358=CYLINDRICAL_SURFACE('',#17725,4.925);
#1359=CYLINDRICAL_SURFACE('',#17726,4.925);
#1360=CYLINDRICAL_SURFACE('',#17727,4.925);
#1361=CYLINDRICAL_SURFACE('',#17728,4.925);
#1362=CYLINDRICAL_SURFACE('',#17729,4.925);
#1363=CYLINDRICAL_SURFACE('',#17730,4.925);
#1364=CYLINDRICAL_SURFACE('',#17731,4.925);
#1365=CYLINDRICAL_SURFACE('',#17732,4.925);
#1366=CYLINDRICAL_SURFACE('',#17733,4.0705);
#1367=CYLINDRICAL_SURFACE('',#17735,4.0705);
#1368=CYLINDRICAL_SURFACE('',#17736,4.0705);
#1369=CYLINDRICAL_SURFACE('',#17737,4.0705);
#1370=CYLINDRICAL_SURFACE('',#17738,4.0705);
#1371=CYLINDRICAL_SURFACE('',#17739,4.0705);
#1372=CYLINDRICAL_SURFACE('',#17740,4.0705);
#1373=CYLINDRICAL_SURFACE('',#17741,4.0705);
#1374=CYLINDRICAL_SURFACE('',#17742,4.0705);
#1375=CYLINDRICAL_SURFACE('',#17743,4.0705);
#1376=CYLINDRICAL_SURFACE('',#17744,4.0705);
#1377=CYLINDRICAL_SURFACE('',#17745,4.0705);
#1378=CYLINDRICAL_SURFACE('',#17746,4.0705);
#1379=CYLINDRICAL_SURFACE('',#17747,4.0705);
#1380=CYLINDRICAL_SURFACE('',#17748,4.0705);
#1381=CYLINDRICAL_SURFACE('',#17752,4.0705);
#1382=CYLINDRICAL_SURFACE('',#17754,4.925);
#1383=CYLINDRICAL_SURFACE('',#17760,4.0705);
#1384=CYLINDRICAL_SURFACE('',#17764,4.925);
#1385=CYLINDRICAL_SURFACE('',#17768,8.);
#2029=FACE_OUTER_BOUND('',#3098,.T.);
#2030=FACE_OUTER_BOUND('',#3099,.T.);
#2031=FACE_OUTER_BOUND('',#3100,.T.);
#2032=FACE_OUTER_BOUND('',#3101,.T.);
#2033=FACE_OUTER_BOUND('',#3102,.T.);
#2034=FACE_OUTER_BOUND('',#3103,.T.);
#2035=FACE_OUTER_BOUND('',#3104,.T.);
#2036=FACE_OUTER_BOUND('',#3105,.T.);
#2037=FACE_OUTER_BOUND('',#3106,.T.);
#2038=FACE_OUTER_BOUND('',#3107,.T.);
#2039=FACE_OUTER_BOUND('',#3108,.T.);
#2040=FACE_OUTER_BOUND('',#3109,.T.);
#2041=FACE_OUTER_BOUND('',#3110,.T.);
#2042=FACE_OUTER_BOUND('',#3111,.T.);
#2043=FACE_OUTER_BOUND('',#3112,.T.);
#2044=FACE_OUTER_BOUND('',#3113,.T.);
#2045=FACE_OUTER_BOUND('',#3114,.T.);
#2046=FACE_OUTER_BOUND('',#3115,.T.);
#2047=FACE_OUTER_BOUND('',#3116,.T.);
#2048=FACE_OUTER_BOUND('',#3117,.T.);
#2049=FACE_OUTER_BOUND('',#3118,.T.);
#2050=FACE_OUTER_BOUND('',#3119,.T.);
#2051=FACE_OUTER_BOUND('',#3120,.T.);
#2052=FACE_OUTER_BOUND('',#3121,.T.);
#2053=FACE_OUTER_BOUND('',#3122,.T.);
#2054=FACE_OUTER_BOUND('',#3123,.T.);
#2055=FACE_OUTER_BOUND('',#3124,.T.);
#2056=FACE_OUTER_BOUND('',#3125,.T.);
#2057=FACE_OUTER_BOUND('',#3126,.T.);
#2058=FACE_OUTER_BOUND('',#3127,.T.);
#2059=FACE_OUTER_BOUND('',#3128,.T.);
#2060=FACE_OUTER_BOUND('',#3129,.T.);
#2061=FACE_OUTER_BOUND('',#3130,.T.);
#2062=FACE_OUTER_BOUND('',#3131,.T.);
#2063=FACE_OUTER_BOUND('',#3132,.T.);
#2064=FACE_OUTER_BOUND('',#3133,.T.);
#2065=FACE_OUTER_BOUND('',#3134,.T.);
#2066=FACE_OUTER_BOUND('',#3135,.T.);
#2067=FACE_OUTER_BOUND('',#3136,.T.);
#2068=FACE_OUTER_BOUND('',#3137,.T.);
#2069=FACE_OUTER_BOUND('',#3138,.T.);
#2070=FACE_OUTER_BOUND('',#3139,.T.);
#2071=FACE_OUTER_BOUND('',#3140,.T.);
#2072=FACE_OUTER_BOUND('',#3141,.T.);
#2073=FACE_OUTER_BOUND('',#3142,.T.);
#2074=FACE_OUTER_BOUND('',#3143,.T.);
#2075=FACE_OUTER_BOUND('',#3144,.T.);
#2076=FACE_OUTER_BOUND('',#3145,.T.);
#2077=FACE_OUTER_BOUND('',#3146,.T.);
#2078=FACE_OUTER_BOUND('',#3147,.T.);
#2079=FACE_OUTER_BOUND('',#3148,.T.);
#2080=FACE_OUTER_BOUND('',#3149,.T.);
#2081=FACE_OUTER_BOUND('',#3150,.T.);
#2082=FACE_OUTER_BOUND('',#3151,.T.);
#2083=FACE_OUTER_BOUND('',#3152,.T.);
#2084=FACE_OUTER_BOUND('',#3153,.T.);
#2085=FACE_OUTER_BOUND('',#3154,.T.);
#2086=FACE_OUTER_BOUND('',#3155,.T.);
#2087=FACE_OUTER_BOUND('',#3156,.T.);
#2088=FACE_OUTER_BOUND('',#3157,.T.);
#2089=FACE_OUTER_BOUND('',#3158,.T.);
#2090=FACE_OUTER_BOUND('',#3159,.T.);
#2091=FACE_OUTER_BOUND('',#3160,.T.);
#2092=FACE_OUTER_BOUND('',#3161,.T.);
#2093=FACE_OUTER_BOUND('',#3162,.T.);
#2094=FACE_OUTER_BOUND('',#3163,.T.);
#2095=FACE_OUTER_BOUND('',#3164,.T.);
#2096=FACE_OUTER_BOUND('',#3165,.T.);
#2097=FACE_OUTER_BOUND('',#3166,.T.);
#2098=FACE_OUTER_BOUND('',#3167,.T.);
#2099=FACE_OUTER_BOUND('',#3168,.T.);
#2100=FACE_OUTER_BOUND('',#3169,.T.);
#2101=FACE_OUTER_BOUND('',#3170,.T.);
#2102=FACE_OUTER_BOUND('',#3172,.T.);
#2103=FACE_OUTER_BOUND('',#3173,.T.);
#2104=FACE_OUTER_BOUND('',#3175,.T.);
#2105=FACE_OUTER_BOUND('',#3176,.T.);
#3098=EDGE_LOOP('',(#11848,#11849,#11850,#11851));
#3099=EDGE_LOOP('',(#11852,#11853,#11854,#11855));
#3100=EDGE_LOOP('',(#11856,#11857,#11858,#11859));
#3101=EDGE_LOOP('',(#11860,#11861,#11862,#11863));
#3102=EDGE_LOOP('',(#11864,#11865,#11866,#11867));
#3103=EDGE_LOOP('',(#11868,#11869,#11870,#11871));
#3104=EDGE_LOOP('',(#11872,#11873,#11874,#11875));
#3105=EDGE_LOOP('',(#11876,#11877,#11878,#11879));
#3106=EDGE_LOOP('',(#11880,#11881,#11882,#11883));
#3107=EDGE_LOOP('',(#11884,#11885,#11886,#11887));
#3108=EDGE_LOOP('',(#11888,#11889,#11890,#11891));
#3109=EDGE_LOOP('',(#11892,#11893,#11894,#11895));
#3110=EDGE_LOOP('',(#11896,#11897,#11898,#11899));
#3111=EDGE_LOOP('',(#11900,#11901,#11902,#11903));
#3112=EDGE_LOOP('',(#11904,#11905,#11906,#11907));
#3113=EDGE_LOOP('',(#11908,#11909,#11910,#11911));
#3114=EDGE_LOOP('',(#11912,#11913,#11914,#11915));
#3115=EDGE_LOOP('',(#11916,#11917,#11918,#11919));
#3116=EDGE_LOOP('',(#11920,#11921,#11922,#11923));
#3117=EDGE_LOOP('',(#11924,#11925,#11926,#11927));
#3118=EDGE_LOOP('',(#11928,#11929,#11930,#11931));
#3119=EDGE_LOOP('',(#11932,#11933,#11934,#11935));
#3120=EDGE_LOOP('',(#11936,#11937,#11938,#11939));
#3121=EDGE_LOOP('',(#11940,#11941,#11942,#11943));
#3122=EDGE_LOOP('',(#11944,#11945,#11946,#11947));
#3123=EDGE_LOOP('',(#11948,#11949,#11950,#11951));
#3124=EDGE_LOOP('',(#11952,#11953,#11954,#11955));
#3125=EDGE_LOOP('',(#11956,#11957,#11958,#11959));
#3126=EDGE_LOOP('',(#11960,#11961,#11962,#11963));
#3127=EDGE_LOOP('',(#11964,#11965,#11966,#11967));
#3128=EDGE_LOOP('',(#11968,#11969,#11970,#11971));
#3129=EDGE_LOOP('',(#11972,#11973,#11974,#11975));
#3130=EDGE_LOOP('',(#11976,#11977,#11978,#11979));
#3131=EDGE_LOOP('',(#11980,#11981,#11982,#11983));
#3132=EDGE_LOOP('',(#11984,#11985,#11986,#11987));
#3133=EDGE_LOOP('',(#11988,#11989,#11990,#11991));
#3134=EDGE_LOOP('',(#11992,#11993,#11994,#11995));
#3135=EDGE_LOOP('',(#11996,#11997,#11998,#11999));
#3136=EDGE_LOOP('',(#12000,#12001,#12002,#12003));
#3137=EDGE_LOOP('',(#12004,#12005,#12006,#12007));
#3138=EDGE_LOOP('',(#12008,#12009,#12010,#12011));
#3139=EDGE_LOOP('',(#12012,#12013,#12014,#12015));
#3140=EDGE_LOOP('',(#12016,#12017,#12018,#12019));
#3141=EDGE_LOOP('',(#12020,#12021,#12022,#12023));
#3142=EDGE_LOOP('',(#12024,#12025,#12026,#12027));
#3143=EDGE_LOOP('',(#12028,#12029,#12030,#12031));
#3144=EDGE_LOOP('',(#12032,#12033,#12034,#12035));
#3145=EDGE_LOOP('',(#12036,#12037,#12038,#12039));
#3146=EDGE_LOOP('',(#12040,#12041,#12042,#12043));
#3147=EDGE_LOOP('',(#12044,#12045,#12046,#12047));
#3148=EDGE_LOOP('',(#12048,#12049,#12050,#12051));
#3149=EDGE_LOOP('',(#12052,#12053,#12054,#12055));
#3150=EDGE_LOOP('',(#12056,#12057,#12058,#12059));
#3151=EDGE_LOOP('',(#12060,#12061,#12062,#12063));
#3152=EDGE_LOOP('',(#12064,#12065,#12066,#12067));
#3153=EDGE_LOOP('',(#12068,#12069,#12070,#12071));
#3154=EDGE_LOOP('',(#12072,#12073,#12074,#12075));
#3155=EDGE_LOOP('',(#12076,#12077,#12078,#12079));
#3156=EDGE_LOOP('',(#12080,#12081,#12082,#12083));
#3157=EDGE_LOOP('',(#12084,#12085,#12086,#12087));
#3158=EDGE_LOOP('',(#12088,#12089,#12090,#12091,#12092));
#3159=EDGE_LOOP('',(#12093,#12094,#12095,#12096,#12097,#12098,#12099,#12100,
#12101,#12102,#12103,#12104,#12105,#12106,#12107,#12108,#12109,#12110,#12111,
#12112,#12113,#12114,#12115,#12116,#12117,#12118,#12119,#12120,#12121,#12122,
#12123,#12124,#12125,#12126));
#3160=EDGE_LOOP('',(#12127,#12128,#12129,#12130));
#3161=EDGE_LOOP('',(#12131,#12132,#12133,#12134,#12135,#12136,#12137,#12138,
#12139,#12140,#12141,#12142,#12143,#12144,#12145,#12146,#12147,#12148,#12149,
#12150,#12151,#12152,#12153,#12154,#12155,#12156,#12157,#12158,#12159,#12160,
#12161,#12162,#12163,#12164));
#3162=EDGE_LOOP('',(#12165,#12166,#12167,#12168));
#3163=EDGE_LOOP('',(#12169,#12170,#12171,#12172,#12173,#12174,#12175,#12176,
#12177,#12178,#12179,#12180,#12181,#12182,#12183,#12184,#12185,#12186,#12187,
#12188,#12189,#12190,#12191,#12192,#12193,#12194,#12195,#12196,#12197,#12198,
#12199,#12200,#12201,#12202));
#3164=EDGE_LOOP('',(#12203,#12204,#12205,#12206,#12207));
#3165=EDGE_LOOP('',(#12208,#12209,#12210,#12211));
#3166=EDGE_LOOP('',(#12212,#12213,#12214,#12215,#12216,#12217,#12218,#12219,
#12220,#12221,#12222,#12223,#12224,#12225,#12226,#12227,#12228,#12229,#12230,
#12231,#12232,#12233,#12234,#12235,#12236,#12237,#12238,#12239,#12240,#12241,
#12242,#12243,#12244,#12245));
#3167=EDGE_LOOP('',(#12246));
#3168=EDGE_LOOP('',(#12247,#12248,#12249,#12250,#12251,#12252));
#3169=EDGE_LOOP('',(#12253,#12254,#12255,#12256));
#3170=EDGE_LOOP('',(#12257));
#3171=EDGE_LOOP('',(#12258,#12259,#12260,#12261));
#3172=EDGE_LOOP('',(#12262,#12263,#12264,#12265));
#3173=EDGE_LOOP('',(#12266));
#3174=EDGE_LOOP('',(#12267,#12268,#12269,#12270));
#3175=EDGE_LOOP('',(#12271,#12272,#12273,#12274,#12275,#12276));
#3176=EDGE_LOOP('',(#12277));
#4103=LINE('',#25125,#5057);
#4104=LINE('',#25158,#5058);
#4105=LINE('',#25242,#5059);
#4106=LINE('',#25332,#5060);
#4107=LINE('',#25422,#5061);
#4108=LINE('',#25506,#5062);
#4109=LINE('',#25596,#5063);
#4110=LINE('',#25680,#5064);
#4111=LINE('',#25767,#5065);
#4112=LINE('',#25842,#5066);
#4113=LINE('',#25926,#5067);
#4114=LINE('',#26016,#5068);
#4115=LINE('',#26100,#5069);
#4116=LINE('',#26187,#5070);
#4117=LINE('',#26277,#5071);
#4118=LINE('',#26361,#5072);
#4119=LINE('',#26383,#5073);
#4120=LINE('',#26420,#5074);
#4121=LINE('',#26457,#5075);
#4122=LINE('',#26495,#5076);
#4123=LINE('',#26532,#5077);
#4124=LINE('',#26569,#5078);
#4125=LINE('',#26606,#5079);
#4126=LINE('',#26641,#5080);
#4127=LINE('',#26675,#5081);
#4128=LINE('',#26712,#5082);
#4129=LINE('',#26749,#5083);
#4130=LINE('',#26786,#5084);
#4131=LINE('',#26823,#5085);
#4132=LINE('',#26861,#5086);
#4133=LINE('',#26898,#5087);
#4134=LINE('',#26931,#5088);
#4135=LINE('',#27015,#5089);
#4136=LINE('',#27105,#5090);
#4137=LINE('',#27195,#5091);
#4138=LINE('',#27279,#5092);
#4139=LINE('',#27369,#5093);
#4140=LINE('',#27453,#5094);
#4141=LINE('',#27540,#5095);
#4142=LINE('',#27615,#5096);
#4143=LINE('',#27699,#5097);
#4144=LINE('',#27789,#5098);
#4145=LINE('',#27873,#5099);
#4146=LINE('',#27960,#5100);
#4147=LINE('',#28050,#5101);
#4148=LINE('',#28134,#5102);
#4149=LINE('',#28156,#5103);
#4150=LINE('',#28193,#5104);
#4151=LINE('',#28230,#5105);
#4152=LINE('',#28268,#5106);
#4153=LINE('',#28305,#5107);
#4154=LINE('',#28342,#5108);
#4155=LINE('',#28379,#5109);
#4156=LINE('',#28414,#5110);
#4157=LINE('',#28448,#5111);
#4158=LINE('',#28485,#5112);
#4159=LINE('',#28522,#5113);
#4160=LINE('',#28559,#5114);
#4161=LINE('',#28596,#5115);
#4162=LINE('',#28634,#5116);
#4163=LINE('',#32870,#5117);
#4164=LINE('',#32879,#5118);
#4165=LINE('',#32884,#5119);
#5057=VECTOR('',#19983,5.);
#5058=VECTOR('',#19988,5.);
#5059=VECTOR('',#19991,5.);
#5060=VECTOR('',#19994,5.);
#5061=VECTOR('',#19997,5.);
#5062=VECTOR('',#20000,5.);
#5063=VECTOR('',#20003,5.);
#5064=VECTOR('',#20006,5.);
#5065=VECTOR('',#20009,5.);
#5066=VECTOR('',#20012,5.);
#5067=VECTOR('',#20015,5.);
#5068=VECTOR('',#20018,5.);
#5069=VECTOR('',#20021,5.);
#5070=VECTOR('',#20024,5.);
#5071=VECTOR('',#20027,5.);
#5072=VECTOR('',#20030,4.0705);
#5073=VECTOR('',#20035,4.0705);
#5074=VECTOR('',#20038,4.0705);
#5075=VECTOR('',#20041,4.0705);
#5076=VECTOR('',#20044,4.0705);
#5077=VECTOR('',#20047,4.0705);
#5078=VECTOR('',#20050,4.0705);
#5079=VECTOR('',#20053,4.0705);
#5080=VECTOR('',#20056,4.0705);
#5081=VECTOR('',#20059,4.0705);
#5082=VECTOR('',#20062,4.0705);
#5083=VECTOR('',#20065,4.0705);
#5084=VECTOR('',#20068,4.0705);
#5085=VECTOR('',#20071,4.0705);
#5086=VECTOR('',#20074,4.0705);
#5087=VECTOR('',#20077,5.);
#5088=VECTOR('',#20082,5.);
#5089=VECTOR('',#20085,5.);
#5090=VECTOR('',#20088,5.);
#5091=VECTOR('',#20091,5.);
#5092=VECTOR('',#20094,5.);
#5093=VECTOR('',#20097,5.);
#5094=VECTOR('',#20100,5.);
#5095=VECTOR('',#20103,5.);
#5096=VECTOR('',#20106,5.);
#5097=VECTOR('',#20109,5.);
#5098=VECTOR('',#20112,5.);
#5099=VECTOR('',#20115,5.);
#5100=VECTOR('',#20118,5.);
#5101=VECTOR('',#20121,5.);
#5102=VECTOR('',#20124,4.0705);
#5103=VECTOR('',#20129,4.0705);
#5104=VECTOR('',#20132,4.0705);
#5105=VECTOR('',#20135,4.0705);
#5106=VECTOR('',#20138,4.0705);
#5107=VECTOR('',#20141,4.0705);
#5108=VECTOR('',#20144,4.0705);
#5109=VECTOR('',#20147,4.0705);
#5110=VECTOR('',#20150,4.0705);
#5111=VECTOR('',#20153,4.0705);
#5112=VECTOR('',#20156,4.0705);
#5113=VECTOR('',#20159,4.0705);
#5114=VECTOR('',#20162,4.0705);
#5115=VECTOR('',#20165,4.0705);
#5116=VECTOR('',#20168,4.0705);
#5117=VECTOR('',#20199,4.75);
#5118=VECTOR('',#20212,8.);
#5119=VECTOR('',#20219,4.75);
#5881=B_SPLINE_CURVE_WITH_KNOTS('',3,(#25127,#25128,#25129,#25130,#25131,
#25132,#25133,#25134,#25135,#25136,#25137,#25138,#25139,#25140,#25141,#25142),
 .UNSPECIFIED.,.F.,.F.,(4,3,3,3,3,4),(-4.09323272002468,-3.98467880200839,
-3.48659395175734,-2.9885091015063,-2.49042425125525,-2.06652207565085),
 .UNSPECIFIED.);
#5882=B_SPLINE_CURVE_WITH_KNOTS('',3,(#25145,#25146,#25147,#25148,#25149,
#25150,#25151,#25152,#25153,#25154),.UNSPECIFIED.,.F.,.F.,(4,3,3,4),(0.,
0.498084850251037,0.996169700502089,1.11488200921589),.UNSPECIFIED.);
#5883=B_SPLINE_CURVE_WITH_KNOTS('',3,(#25159,#25160,#25161,#25162,#25163,
#25164,#25165,#25166,#25167,#25168,#25169,#25170,#25171,#25172,#25173,#25174,
#25175,#25176,#25177,#25178,#25179,#25180,#25181,#25182,#25183,#25184,#25185,
#25186,#25187,#25188,#25189,#25190,#25191,#25192,#25193,#25194,#25195,#25196,
#25197,#25198),.UNSPECIFIED.,.F.,.F.,(4,3,3,3,3,3,3,3,3,3,3,3,3,4),(-10.3764180272042,
-9.96169700502099,-9.46361215476994,-8.96552730451889,-8.46744245426784,
-7.96935760401679,-7.47127275376574,-6.97318790351469,-6.47510305326364,
-5.9770182030126,-5.47893335276154,-4.9808485025105,-4.48276365225944,-4.09323272002468),
 .UNSPECIFIED.);
#5884=B_SPLINE_CURVE_WITH_KNOTS('',3,(#25199,#25200,#25201,#25202,#25203,
#25204,#25205,#25206,#25207,#25208,#25209,#25210,#25211,#25212,#25213,#25214,
#25215,#25216,#25217,#25218,#25219,#25220,#25221,#25222,#25223,#25224,#25225,
#25226,#25227,#25228,#25229,#25230,#25231,#25232,#25233,#25234,#25235,#25236,
#25237,#25238),.UNSPECIFIED.,.F.,.F.,(4,3,3,3,3,3,3,3,3,3,3,3,3,4),(1.11488200921589,
1.49425455075314,1.99233940100419,2.49042425125524,2.98850910150629,3.48659395175734,
3.98467880200839,4.48276365225944,4.98084850251049,5.47893335276154,5.97701820301259,
6.47510305326364,6.97318790351469,7.39806731639545),.UNSPECIFIED.);
#5885=B_SPLINE_CURVE_WITH_KNOTS('',3,(#25243,#25244,#25245,#25246,#25247,
#25248,#25249,#25250,#25251,#25252,#25253,#25254,#25255,#25256,#25257,#25258,
#25259,#25260,#25261,#25262,#25263,#25264,#25265,#25266,#25267,#25268,#25269,
#25270,#25271,#25272,#25273,#25274,#25275,#25276,#25277,#25278,#25279,#25280,
#25281,#25282,#25283,#25284,#25285),.UNSPECIFIED.,.F.,.F.,(4,3,3,3,3,3,
3,3,3,3,3,3,3,3,4),(-16.6596033343838,-16.4368000582846,-15.9387152080336,
-15.4406303577825,-14.9425455075315,-14.4444606572804,-13.9463758070294,
-13.4482909567783,-12.9502061065273,-12.4521212562762,-11.9540364060252,
-11.4559515557741,-10.9578667055231,-10.459781855272,-10.3764180272042),
 .UNSPECIFIED.);
#5886=B_SPLINE_CURVE_WITH_KNOTS('',3,(#25286,#25287,#25288,#25289,#25290,
#25291,#25292,#25293,#25294,#25295,#25296,#25297,#25298,#25299,#25300,#25301,
#25302,#25303,#25304,#25305,#25306,#25307,#25308,#25309,#25310,#25311,#25312,
#25313,#25314,#25315,#25316,#25317,#25318,#25319,#25320,#25321,#25322,#25323,
#25324,#25325,#25326,#25327,#25328),.UNSPECIFIED.,.F.,.F.,(4,3,3,3,3,3,
3,3,3,3,3,3,3,3,4),(7.39806731639545,7.47127275376574,7.96935760401679,
8.46744245426784,8.96552730451889,9.46361215476994,9.96169700502099,10.459781855272,
10.9578667055231,11.4559515557741,11.9540364060252,12.4521212562762,12.9502061065273,
13.4482909567783,13.681252623575),.UNSPECIFIED.);
#5887=B_SPLINE_CURVE_WITH_KNOTS('',3,(#25333,#25334,#25335,#25336,#25337,
#25338,#25339,#25340,#25341,#25342,#25343,#25344,#25345,#25346,#25347,#25348,
#25349,#25350,#25351,#25352,#25353,#25354,#25355,#25356,#25357,#25358,#25359,
#25360,#25361,#25362,#25363,#25364,#25365,#25366,#25367,#25368,#25369,#25370,
#25371,#25372,#25373,#25374,#25375),.UNSPECIFIED.,.F.,.F.,(4,3,3,3,3,3,
3,3,3,3,3,3,3,3,4),(-22.9427886415634,-22.9119031115483,-22.4138182612972,
-21.9157334110462,-21.4176485607951,-20.9195637105441,-20.421478860293,
-19.923394010042,-19.4253091597909,-18.9272243095399,-18.4291394592888,
-17.9310546090378,-17.4329697587867,-16.9348849085357,-16.6596033343838),
 .UNSPECIFIED.);
#5888=B_SPLINE_CURVE_WITH_KNOTS('',3,(#25376,#25377,#25378,#25379,#25380,
#25381,#25382,#25383,#25384,#25385,#25386,#25387,#25388,#25389,#25390,#25391,
#25392,#25393,#25394,#25395,#25396,#25397,#25398,#25399,#25400,#25401,#25402,
#25403,#25404,#25405,#25406,#25407,#25408,#25409,#25410,#25411,#25412,#25413,
#25414,#25415,#25416,#25417,#25418),.UNSPECIFIED.,.F.,.F.,(4,3,3,3,3,3,
3,3,3,3,3,3,3,3,4),(13.681252623575,13.9463758070294,14.4444606572804,14.9425455075315,
15.4406303577825,15.9387152080336,16.4368000582846,16.9348849085357,17.4329697587867,
17.9310546090378,18.4291394592888,18.9272243095399,19.4253091597909,19.923394010042,
19.9644379307546),.UNSPECIFIED.);
#5889=B_SPLINE_CURVE_WITH_KNOTS('',3,(#25423,#25424,#25425,#25426,#25427,
#25428,#25429,#25430,#25431,#25432,#25433,#25434,#25435,#25436,#25437,#25438,
#25439,#25440,#25441,#25442,#25443,#25444,#25445,#25446,#25447,#25448,#25449,
#25450,#25451,#25452,#25453,#25454,#25455,#25456,#25457,#25458,#25459,#25460,
#25461,#25462),.UNSPECIFIED.,.F.,.F.,(4,3,3,3,3,3,3,3,3,3,3,3,3,4),(-29.225973948743,
-28.8889213145609,-28.3908364643098,-27.8927516140588,-27.3946667638077,
-26.8965819135567,-26.3984970633056,-25.9004122130546,-25.4023273628035,
-24.9042425125525,-24.4061576623014,-23.9080728120504,-23.4099879617993,
-22.9427886415634),.UNSPECIFIED.);
#5890=B_SPLINE_CURVE_WITH_KNOTS('',3,(#25463,#25464,#25465,#25466,#25467,
#25468,#25469,#25470,#25471,#25472,#25473,#25474,#25475,#25476,#25477,#25478,
#25479,#25480,#25481,#25482,#25483,#25484,#25485,#25486,#25487,#25488,#25489,
#25490,#25491,#25492,#25493,#25494,#25495,#25496,#25497,#25498,#25499,#25500,
#25501,#25502),.UNSPECIFIED.,.F.,.F.,(4,3,3,3,3,3,3,3,3,3,3,3,3,4),(19.9644379307546,
20.421478860293,20.9195637105441,21.4176485607951,21.9157334110462,22.4138182612972,
22.9119031115483,23.4099879617993,23.9080728120504,24.4061576623014,24.9042425125525,
25.4023273628035,25.9004122130546,26.2476232379342),.UNSPECIFIED.);
#5891=B_SPLINE_CURVE_WITH_KNOTS('',3,(#25507,#25508,#25509,#25510,#25511,
#25512,#25513,#25514,#25515,#25516,#25517,#25518,#25519,#25520,#25521,#25522,
#25523,#25524,#25525,#25526,#25527,#25528,#25529,#25530,#25531,#25532,#25533,
#25534,#25535,#25536,#25537,#25538,#25539,#25540,#25541,#25542,#25543,#25544,
#25545,#25546,#25547,#25548,#25549),.UNSPECIFIED.,.F.,.F.,(4,3,3,3,3,3,
3,3,3,3,3,3,3,3,4),(-35.5091592559226,-35.3640243678245,-34.8659395175735,
-34.3678546673224,-33.8697698170714,-33.3716849668203,-32.8736001165693,
-32.3755152663182,-31.8774304160672,-31.3793455658161,-30.8812607155651,
-30.383175865314,-29.885091015063,-29.3870061648119,-29.225973948743),
 .UNSPECIFIED.);
#5892=B_SPLINE_CURVE_WITH_KNOTS('',3,(#25550,#25551,#25552,#25553,#25554,
#25555,#25556,#25557,#25558,#25559,#25560,#25561,#25562,#25563,#25564,#25565,
#25566,#25567,#25568,#25569,#25570,#25571,#25572,#25573,#25574,#25575,#25576,
#25577,#25578,#25579,#25580,#25581,#25582,#25583,#25584,#25585,#25586,#25587,
#25588,#25589,#25590,#25591,#25592),.UNSPECIFIED.,.F.,.F.,(4,3,3,3,3,3,
3,3,3,3,3,3,3,3,4),(26.2476232379342,26.3984970633056,26.8965819135567,
27.3946667638077,27.8927516140588,28.3908364643098,28.8889213145609,29.3870061648119,
29.885091015063,30.383175865314,30.8812607155651,31.3793455658161,31.8774304160672,
32.3755152663182,32.5308085451138),.UNSPECIFIED.);
#5893=B_SPLINE_CURVE_WITH_KNOTS('',3,(#25597,#25598,#25599,#25600,#25601,
#25602,#25603,#25604,#25605,#25606,#25607,#25608,#25609,#25610,#25611,#25612,
#25613,#25614,#25615,#25616,#25617,#25618,#25619,#25620,#25621,#25622,#25623,
#25624,#25625,#25626,#25627,#25628,#25629,#25630,#25631,#25632,#25633,#25634,
#25635,#25636),.UNSPECIFIED.,.F.,.F.,(4,3,3,3,3,3,3,3,3,3,3,3,3,4),(-41.7923445631022,
-41.3410425708371,-40.842957720586,-40.344872870335,-39.846788020084,-39.3487031698329,
-38.8506183195819,-38.3525334693308,-37.8544486190798,-37.3563637688287,
-36.8582789185777,-36.3601940683266,-35.8621092180756,-35.5091592559226),
 .UNSPECIFIED.);
#5894=B_SPLINE_CURVE_WITH_KNOTS('',3,(#25637,#25638,#25639,#25640,#25641,
#25642,#25643,#25644,#25645,#25646,#25647,#25648,#25649,#25650,#25651,#25652,
#25653,#25654,#25655,#25656,#25657,#25658,#25659,#25660,#25661,#25662,#25663,
#25664,#25665,#25666,#25667,#25668,#25669,#25670,#25671,#25672,#25673,#25674,
#25675,#25676),.UNSPECIFIED.,.F.,.F.,(4,3,3,3,3,3,3,3,3,3,3,3,3,4),(32.5308085451138,
32.8736001165693,33.3716849668203,33.8697698170714,34.3678546673224,34.8659395175735,
35.3640243678245,35.8621092180756,36.3601940683266,36.8582789185776,37.3563637688287,
37.8544486190798,38.3525334693308,38.8139938522934),.UNSPECIFIED.);
#5895=B_SPLINE_CURVE_WITH_KNOTS('',3,(#25681,#25682,#25683,#25684,#25685,
#25686,#25687,#25688,#25689,#25690,#25691,#25692,#25693,#25694,#25695,#25696,
#25697,#25698,#25699,#25700,#25701,#25702,#25703,#25704,#25705,#25706,#25707,
#25708,#25709,#25710,#25711,#25712,#25713,#25714,#25715,#25716,#25717,#25718,
#25719,#25720),.UNSPECIFIED.,.F.,.F.,(4,3,3,3,3,3,3,3,3,3,3,3,3,4),(-48.0755298702818,
-47.8161456241007,-46.8199759235986,-46.3218910733476,-45.8238062230966,
-45.3257213728455,-44.8276365225944,-44.3295516723434,-43.8314668220923,
-43.3333819718413,-42.8352971215903,-42.3372122713392,-41.8391274210882,
-41.7923445631022),.UNSPECIFIED.);
#5896=B_SPLINE_CURVE_WITH_KNOTS('',3,(#25721,#25722,#25723,#25724,#25725,
#25726,#25727,#25728,#25729,#25730,#25731,#25732,#25733,#25734,#25735,#25736,
#25737,#25738,#25739,#25740,#25741,#25742,#25743,#25744,#25745,#25746,#25747,
#25748,#25749,#25750,#25751,#25752,#25753,#25754,#25755,#25756,#25757,#25758,
#25759,#25760,#25761,#25762,#25763),.UNSPECIFIED.,.F.,.F.,(4,3,3,3,3,3,
3,3,3,3,3,3,3,3,4),(38.8139938522934,38.8506183195818,39.3487031698329,
39.846788020084,40.344872870335,40.842957720586,41.3410425708371,41.8391274210882,
42.3372122713392,42.8352971215903,43.3333819718413,43.8314668220924,44.3295516723434,
44.8276365225945,45.097179159473),.UNSPECIFIED.);
#5897=B_SPLINE_CURVE_WITH_KNOTS('',3,(#25768,#25769,#25770,#25771,#25772,
#25773,#25774,#25775,#25776,#25777,#25778,#25779,#25780,#25781,#25782,#25783,
#25784,#25785,#25786,#25787,#25788,#25789,#25790,#25791,#25792,#25793,#25794,
#25795,#25796,#25797,#25798,#25799,#25800,#25801,#25802,#25803,#25804),
 .UNSPECIFIED.,.F.,.F.,(4,3,3,3,3,3,3,3,3,3,3,3,4),(-54.3587151774614,-54.2912486773644,
-53.7931638271134,-53.2950789768623,-52.7969941266112,-52.2989092763602,
-51.8008244261091,-51.3027395758581,-50.8046547256071,-50.306569875356,
-49.8084850251049,-48.8123153246028,-48.0755298702818),.UNSPECIFIED.);
#5898=B_SPLINE_CURVE_WITH_KNOTS('',3,(#25805,#25806,#25807,#25808,#25809,
#25810,#25811,#25812,#25813,#25814,#25815,#25816,#25817,#25818,#25819,#25820,
#25821,#25822,#25823,#25824,#25825,#25826,#25827,#25828,#25829,#25830,#25831,
#25832,#25833,#25834,#25835,#25836,#25837,#25838),.UNSPECIFIED.,.F.,.F.,
(4,3,3,3,3,3,3,3,3,3,3,4),(45.097179159473,45.3257213728455,45.8238062230965,
46.3218910733476,46.8199759235986,47.8161456241007,48.8123153246028,49.8084850251049,
50.306569875356,50.8046547256071,51.3027395758581,51.3803644666526),
 .UNSPECIFIED.);
#5899=B_SPLINE_CURVE_WITH_KNOTS('',3,(#25843,#25844,#25845,#25846,#25847,
#25848,#25849,#25850,#25851,#25852,#25853,#25854,#25855,#25856,#25857,#25858,
#25859,#25860,#25861,#25862,#25863,#25864,#25865,#25866,#25867,#25868,#25869,
#25870,#25871,#25872,#25873,#25874,#25875,#25876,#25877,#25878,#25879,#25880,
#25881,#25882),.UNSPECIFIED.,.F.,.F.,(4,3,3,3,3,3,3,3,3,3,3,3,3,4),(-60.641900484641,
-60.268266880377,-59.7701820301259,-59.2720971798749,-58.7740123296238,
-58.2759274793728,-57.7778426291217,-57.2797577788707,-56.7816729286196,
-56.2835880783686,-55.7855032281175,-55.2874183778665,-54.7893335276154,
-54.3587151774614),.UNSPECIFIED.);
#5900=B_SPLINE_CURVE_WITH_KNOTS('',3,(#25883,#25884,#25885,#25886,#25887,
#25888,#25889,#25890,#25891,#25892,#25893,#25894,#25895,#25896,#25897,#25898,
#25899,#25900,#25901,#25902,#25903,#25904,#25905,#25906,#25907,#25908,#25909,
#25910,#25911,#25912,#25913,#25914,#25915,#25916,#25917,#25918,#25919,#25920,
#25921,#25922),.UNSPECIFIED.,.F.,.F.,(4,3,3,3,3,3,3,3,3,3,3,3,3,4),(51.3803644666526,
51.8008244261091,52.2989092763602,52.7969941266112,53.2950789768623,53.7931638271133,
54.2912486773644,54.7893335276154,55.2874183778665,55.7855032281175,56.2835880783686,
56.7816729286196,57.2797577788707,57.6635497738322),.UNSPECIFIED.);
#5901=B_SPLINE_CURVE_WITH_KNOTS('',3,(#25927,#25928,#25929,#25930,#25931,
#25932,#25933,#25934,#25935,#25936,#25937,#25938,#25939,#25940,#25941,#25942,
#25943,#25944,#25945,#25946,#25947,#25948,#25949,#25950,#25951,#25952,#25953,
#25954,#25955,#25956,#25957,#25958,#25959,#25960,#25961,#25962,#25963,#25964,
#25965,#25966,#25967,#25968,#25969),.UNSPECIFIED.,.F.,.F.,(4,3,3,3,3,3,
3,3,3,3,3,3,3,3,4),(-66.9250857918206,-66.7433699336406,-66.2452850833896,
-65.7472002331385,-65.2491153828875,-64.7510305326364,-64.2529456823854,
-63.7548608321343,-63.2567759818833,-62.7586911316322,-62.2606062813812,
-61.7625214311301,-61.2644365808791,-60.766351730628,-60.641900484641),
 .UNSPECIFIED.);
#5902=B_SPLINE_CURVE_WITH_KNOTS('',3,(#25970,#25971,#25972,#25973,#25974,
#25975,#25976,#25977,#25978,#25979,#25980,#25981,#25982,#25983,#25984,#25985,
#25986,#25987,#25988,#25989,#25990,#25991,#25992,#25993,#25994,#25995,#25996,
#25997,#25998,#25999,#26000,#26001,#26002,#26003,#26004,#26005,#26006,#26007,
#26008,#26009,#26010,#26011,#26012),.UNSPECIFIED.,.F.,.F.,(4,3,3,3,3,3,
3,3,3,3,3,3,3,3,4),(57.6635497738322,57.7778426291217,58.2759274793728,
58.7740123296238,59.2720971798749,59.7701820301259,60.268266880377,60.766351730628,
61.2644365808791,61.7625214311301,62.2606062813812,62.7586911316322,63.2567759818833,
63.7548608321343,63.9467350810118),.UNSPECIFIED.);
#5903=B_SPLINE_CURVE_WITH_KNOTS('',3,(#26017,#26018,#26019,#26020,#26021,
#26022,#26023,#26024,#26025,#26026,#26027,#26028,#26029,#26030,#26031,#26032,
#26033,#26034,#26035,#26036,#26037,#26038,#26039,#26040,#26041,#26042,#26043,
#26044,#26045,#26046,#26047,#26048,#26049,#26050,#26051,#26052,#26053,#26054,
#26055,#26056),.UNSPECIFIED.,.F.,.F.,(4,3,3,3,3,3,3,3,3,3,3,3,3,4),(-73.2082710990001,
-72.7203881366532,-72.2223032864022,-71.7242184361511,-71.2261335859001,
-70.728048735649,-70.229963885398,-69.7318790351469,-69.2337941848959,-68.7357093346448,
-68.2376244843938,-67.7395396341427,-67.2414547838917,-66.9250857918206),
 .UNSPECIFIED.);
#5904=B_SPLINE_CURVE_WITH_KNOTS('',3,(#26057,#26058,#26059,#26060,#26061,
#26062,#26063,#26064,#26065,#26066,#26067,#26068,#26069,#26070,#26071,#26072,
#26073,#26074,#26075,#26076,#26077,#26078,#26079,#26080,#26081,#26082,#26083,
#26084,#26085,#26086,#26087,#26088,#26089,#26090,#26091,#26092,#26093,#26094,
#26095,#26096),.UNSPECIFIED.,.F.,.F.,(4,3,3,3,3,3,3,3,3,3,3,3,3,4),(63.9467350810118,
64.2529456823854,64.7510305326364,65.2491153828875,65.7472002331385,66.2452850833896,
66.7433699336406,67.2414547838917,67.7395396341427,68.2376244843938,68.7357093346448,
69.2337941848959,69.7318790351469,70.2299203881914),.UNSPECIFIED.);
#5905=B_SPLINE_CURVE_WITH_KNOTS('',3,(#26101,#26102,#26103,#26104,#26105,
#26106,#26107,#26108,#26109,#26110,#26111,#26112,#26113,#26114,#26115,#26116,
#26117,#26118,#26119,#26120,#26121,#26122,#26123,#26124,#26125,#26126,#26127,
#26128,#26129,#26130,#26131,#26132,#26133,#26134,#26135,#26136,#26137,#26138,
#26139,#26140,#26141,#26142,#26143),.UNSPECIFIED.,.F.,.F.,(4,3,3,3,3,3,
3,3,3,3,3,3,3,3,4),(-79.4914564061798,-79.1954911899169,-78.6974063396658,
-78.1993214894147,-77.7012366391637,-77.2031517889127,-76.7050669386616,
-76.2069820884106,-75.7088972381595,-75.2108123879085,-74.7127275376574,
-74.2146426874064,-73.7165578371553,-73.2184729869043,-73.2082710990001),
 .UNSPECIFIED.);
#5906=B_SPLINE_CURVE_WITH_KNOTS('',3,(#26144,#26145,#26146,#26147,#26148,
#26149,#26150,#26151,#26152,#26153,#26154,#26155,#26156,#26157,#26158,#26159,
#26160,#26161,#26162,#26163,#26164,#26165,#26166,#26167,#26168,#26169,#26170,
#26171,#26172,#26173,#26174,#26175,#26176,#26177,#26178,#26179,#26180,#26181,
#26182,#26183),.UNSPECIFIED.,.F.,.F.,(4,3,3,3,3,3,3,3,3,3,3,3,3,4),(70.2299203881914,
70.728048735649,71.2261335859,71.7242184361511,72.2223032864022,72.7203881366532,
73.2184729869043,73.7165578371553,74.2146426874063,74.7127275376574,75.2108123879084,
75.7088972381595,76.2069820884106,76.513105695371),.UNSPECIFIED.);
#5907=B_SPLINE_CURVE_WITH_KNOTS('',3,(#26188,#26189,#26190,#26191,#26192,
#26193,#26194,#26195,#26196,#26197,#26198,#26199,#26200,#26201,#26202,#26203,
#26204,#26205,#26206,#26207,#26208,#26209,#26210,#26211,#26212,#26213,#26214,
#26215,#26216,#26217,#26218,#26219,#26220,#26221,#26222,#26223,#26224,#26225,
#26226,#26227,#26228,#26229,#26230),.UNSPECIFIED.,.F.,.F.,(4,3,3,3,3,3,
3,3,3,3,3,3,3,3,4),(-85.7746417133593,-85.6705942431805,-85.1725093929295,
-84.6744245426784,-84.1763396924274,-83.6782548421763,-83.1801699919253,
-82.6820851416742,-82.1840002914231,-81.6859154411721,-81.1878305909211,
-80.68974574067,-80.191660890419,-79.6935760401679,-79.4914564061798),
 .UNSPECIFIED.);
#5908=B_SPLINE_CURVE_WITH_KNOTS('',3,(#26231,#26232,#26233,#26234,#26235,
#26236,#26237,#26238,#26239,#26240,#26241,#26242,#26243,#26244,#26245,#26246,
#26247,#26248,#26249,#26250,#26251,#26252,#26253,#26254,#26255,#26256,#26257,
#26258,#26259,#26260,#26261,#26262,#26263,#26264,#26265,#26266,#26267,#26268,
#26269,#26270,#26271,#26272,#26273),.UNSPECIFIED.,.F.,.F.,(4,3,3,3,3,3,
3,3,3,3,3,3,3,3,4),(76.513105695371,76.7050669386616,77.2031517889126,77.7012366391637,
78.1993214894148,78.6974063396658,79.1954911899169,79.6935760401679,80.1916608904189,
80.68974574067,81.187830590921,81.6859154411721,82.1840002914232,82.6820851416742,
82.7962910025505),.UNSPECIFIED.);
#5909=B_SPLINE_CURVE_WITH_KNOTS('',3,(#26278,#26279,#26280,#26281,#26282,
#26283,#26284,#26285,#26286,#26287,#26288,#26289,#26290,#26291,#26292,#26293,
#26294,#26295,#26296,#26297,#26298,#26299,#26300,#26301,#26302,#26303,#26304,
#26305,#26306,#26307,#26308,#26309,#26310,#26311,#26312,#26313,#26314,#26315,
#26316,#26317),.UNSPECIFIED.,.F.,.F.,(4,3,3,3,3,3,3,3,3,3,3,3,3,4),(-92.0578270205389,
-91.6476124461931,-91.1495275959421,-90.651442745691,-90.15335789544,-89.6552730451889,
-89.1571881949379,-88.6591033446868,-88.1610184944358,-87.6629336441847,
-87.1648487939337,-86.6667639436826,-86.1686790934316,-85.7746417133593),
 .UNSPECIFIED.);
#5910=B_SPLINE_CURVE_WITH_KNOTS('',3,(#26318,#26319,#26320,#26321,#26322,
#26323,#26324,#26325,#26326,#26327,#26328,#26329,#26330,#26331,#26332,#26333,
#26334,#26335,#26336,#26337,#26338,#26339,#26340,#26341,#26342,#26343,#26344,
#26345,#26346,#26347,#26348,#26349,#26350,#26351,#26352,#26353,#26354,#26355,
#26356,#26357),.UNSPECIFIED.,.F.,.F.,(4,3,3,3,3,3,3,3,3,3,3,3,3,4),(82.7962910025505,
83.1801699919253,83.6782548421763,84.1763396924274,84.6744245426784,85.1725093929295,
85.6705942431805,86.1686790934315,86.6667639436826,87.1648487939336,87.6629336441847,
88.1610184944358,88.6591033446868,89.0794763097301),.UNSPECIFIED.);
#5911=B_SPLINE_CURVE_WITH_KNOTS('',3,(#26363,#26364,#26365,#26366,#26367,
#26368,#26369,#26370,#26371),.UNSPECIFIED.,.F.,.F.,(4,1,1,1,1,1,4),(103.672557568463,
103.760427844368,104.258512694619,104.75659754487,105.254682395122,105.752767245373,
106.176669420977),.UNSPECIFIED.);
#5912=B_SPLINE_CURVE_WITH_KNOTS('',3,(#26374,#26375,#26376,#26377,#26378,
#26379),.UNSPECIFIED.,.F.,.F.,(4,1,1,4),(103.672557568463,103.942187199755,
104.440272050006,104.938356900257),.UNSPECIFIED.);
#5913=B_SPLINE_CURVE_WITH_KNOTS('',3,(#26384,#26385,#26386,#26387,#26388,
#26389,#26390,#26391,#26392,#26393,#26394,#26395,#26396,#26397,#26398,#26399),
 .UNSPECIFIED.,.F.,.F.,(4,1,1,1,1,1,1,1,1,1,1,1,1,4),(97.3893722612836,
97.7834096413558,98.2814944916068,98.7795793418579,99.2776641921089,99.77574904236,
100.273833892611,100.771918742862,101.270003593113,101.768088443364,102.266173293615,
102.764258143866,103.262342994117,103.672557568463),.UNSPECIFIED.);
#5914=B_SPLINE_CURVE_WITH_KNOTS('',3,(#26400,#26401,#26402,#26403,#26404,
#26405,#26406,#26407,#26408,#26409,#26410,#26411,#26412,#26413,#26414,#26415,
#26416),.UNSPECIFIED.,.F.,.F.,(4,1,1,1,1,1,1,1,1,1,1,1,1,1,4),(97.3893722612836,
97.4670841464912,97.9651689967422,98.4632538469933,98.9613386972443,99.4594235474954,
99.9575083977464,100.455593247997,100.953678098249,101.4517629485,101.949847798751,
102.447932649002,102.946017499253,103.444102349504,103.672557568463),
 .UNSPECIFIED.);
#5915=B_SPLINE_CURVE_WITH_KNOTS('',3,(#26421,#26422,#26423,#26424,#26425,
#26426,#26427,#26428,#26429,#26430,#26431,#26432,#26433,#26434,#26435,#26436,
#26437),.UNSPECIFIED.,.F.,.F.,(4,1,1,1,1,1,1,1,1,1,1,1,1,1,4),(91.106186954104,
91.3083065880921,91.8063914383432,92.3044762885942,92.8025611388453,93.3006459890963,
93.7987308393474,94.2968156895984,94.7949005398495,95.2929853901005,95.7910702403516,
96.2891550906026,96.7872399408537,97.2853247911047,97.3893722612836),
 .UNSPECIFIED.);
#5916=B_SPLINE_CURVE_WITH_KNOTS('',3,(#26438,#26439,#26440,#26441,#26442,
#26443,#26444,#26445,#26446,#26447,#26448,#26449,#26450,#26451,#26452,#26453),
 .UNSPECIFIED.,.F.,.F.,(4,1,1,1,1,1,1,1,1,1,1,1,1,4),(91.106186954104,91.4900659434786,
91.9881507937297,92.4862356439807,92.9843204942318,93.4824053444828,93.9804901947338,
94.4785750449849,94.976659895236,95.474744745487,95.972829595738,96.4709144459891,
96.9689992962401,97.3893722612836),.UNSPECIFIED.);
#5917=B_SPLINE_CURVE_WITH_KNOTS('',3,(#26458,#26459,#26460,#26461,#26462,
#26463,#26464,#26465,#26466,#26467,#26468,#26469,#26470,#26471,#26472,#26473,
#26474),.UNSPECIFIED.,.F.,.F.,(4,1,1,1,1,1,1,1,1,1,1,1,1,1,4),(84.8230016469244,
84.8332035348285,85.3312883850795,85.8293732353306,86.3274580855816,86.8255429358327,
87.3236277860837,87.8217126363348,88.3197974865858,88.8178823368369,89.3159671870879,
89.814052037339,90.31213688759,90.8102217378411,91.106186954104),
 .UNSPECIFIED.);
#5918=B_SPLINE_CURVE_WITH_KNOTS('',3,(#26475,#26476,#26477,#26478,#26479,
#26480,#26481,#26482,#26483,#26484,#26485,#26486,#26487,#26488,#26489,#26490,
#26491),.UNSPECIFIED.,.F.,.F.,(4,1,1,1,1,1,1,1,1,1,1,1,1,1,4),(84.8230016469244,
85.014962890215,85.513047740466,86.0111325907171,86.5092174409681,87.0073022912192,
87.5053871414702,88.0034719917213,88.5015568419723,88.9996416922233,89.4977265424744,
89.9958113927255,90.4938962429765,90.9919810932276,91.106186954104),
 .UNSPECIFIED.);
#5919=B_SPLINE_CURVE_WITH_KNOTS('',3,(#26496,#26497,#26498,#26499,#26500,
#26501,#26502,#26503,#26504,#26505,#26506,#26507,#26508,#26509,#26510,#26511),
 .UNSPECIFIED.,.F.,.F.,(4,1,1,1,1,1,1,1,1,1,1,1,1,4),(78.5398163397448,
78.8561853318159,79.3542701820669,79.852355032318,80.350439882569,80.8485247328201,
81.3466095830711,81.8446944333222,82.3427792835733,82.8408641338243,83.3389489840753,
83.8370338343264,84.3351186845774,84.8230016469244),.UNSPECIFIED.);
#5920=B_SPLINE_CURVE_WITH_KNOTS('',3,(#26512,#26513,#26514,#26515,#26516,
#26517,#26518,#26519,#26520,#26521,#26522,#26523,#26524,#26525,#26526,#26527,
#26528),.UNSPECIFIED.,.F.,.F.,(4,1,1,1,1,1,1,1,1,1,1,1,1,1,4),(78.5398163397448,
78.5398598369513,79.0379446872024,79.5360295374534,80.0341143877045,80.5321992379555,
81.0302840882066,81.5283689384576,82.0264537887087,82.5245386389597,83.0226234892108,
83.5207083394618,84.0187931897129,84.5168780399639,84.8230016469244),
 .UNSPECIFIED.);
#5921=B_SPLINE_CURVE_WITH_KNOTS('',3,(#26533,#26534,#26535,#26536,#26537,
#26538,#26539,#26540,#26541,#26542,#26543,#26544,#26545,#26546,#26547,#26548,
#26549),.UNSPECIFIED.,.F.,.F.,(4,1,1,1,1,1,1,1,1,1,1,1,1,1,4),(72.2566310325652,
72.3810822785523,72.8791671288033,73.3772519790544,73.8753368293054,74.3734216795565,
74.8715065298075,75.3695913800586,75.8676762303096,76.3657610805606,76.8638459308117,
77.3619307810628,77.8600156313138,78.3581004815648,78.5398163397448),
 .UNSPECIFIED.);
#5922=B_SPLINE_CURVE_WITH_KNOTS('',3,(#26550,#26551,#26552,#26553,#26554,
#26555,#26556,#26557,#26558,#26559,#26560,#26561,#26562,#26563,#26564,#26565),
 .UNSPECIFIED.,.F.,.F.,(4,1,1,1,1,1,1,1,1,1,1,1,1,4),(72.2566310325652,
72.5628416339387,73.0609264841898,73.5590113344408,74.0570961846919,74.5551810349429,
75.053265885194,75.551350735445,76.0494355856961,76.5475204359471,77.0456052861982,
77.5436901364492,78.0417749867003,78.5398163397448),.UNSPECIFIED.);
#5923=B_SPLINE_CURVE_WITH_KNOTS('',3,(#26570,#26571,#26572,#26573,#26574,
#26575,#26576,#26577,#26578,#26579,#26580,#26581,#26582,#26583,#26584,#26585),
 .UNSPECIFIED.,.F.,.F.,(4,1,1,1,1,1,1,1,1,1,1,1,1,4),(65.9734457253856,
66.4040640755397,66.9021489257907,67.4002337760418,67.8983186262928,68.3964034765439,
68.8944883267949,69.392573177046,69.890658027297,70.3887428775481,70.8868277277991,
71.3849125780502,71.8829974283012,72.2566310325652),.UNSPECIFIED.);
#5924=B_SPLINE_CURVE_WITH_KNOTS('',3,(#26586,#26587,#26588,#26589,#26590,
#26591,#26592,#26593,#26594,#26595,#26596,#26597,#26598,#26599,#26600,#26601,
#26602),.UNSPECIFIED.,.F.,.F.,(4,1,1,1,1,1,1,1,1,1,1,1,1,1,4),(65.9734457253856,
66.0877385806751,66.5858234309261,67.0839082811772,67.5819931314282,68.0800779816793,
68.5781628319303,69.0762476821814,69.5743325324324,70.0724173826835,70.5705022329345,
71.0685870831856,71.5666719334366,72.0647567836877,72.2566310325652),
 .UNSPECIFIED.);
#5925=B_SPLINE_CURVE_WITH_KNOTS('',3,(#26607,#26608,#26609,#26610,#26611,
#26612,#26613,#26614,#26615,#26616,#26617,#26618,#26619,#26620,#26621),
 .UNSPECIFIED.,.F.,.F.,(4,1,1,1,1,1,1,1,1,1,1,1,4),(59.6902604182061,60.4270458725271,
61.4232155730292,61.9213004232802,62.4193852735313,62.9174701237823,63.4155549740334,
63.9136398242844,64.4117246745355,64.9098095247865,65.4078943750376,65.9059792252886,
65.9734457253856),.UNSPECIFIED.);
#5926=B_SPLINE_CURVE_WITH_KNOTS('',3,(#26622,#26623,#26624,#26625,#26626,
#26627,#26628,#26629,#26630,#26631,#26632,#26633,#26634,#26635,#26636,#26637),
 .UNSPECIFIED.,.F.,.F.,(4,1,1,1,1,1,1,1,1,1,1,1,1,4),(59.690260418206,60.1107203776625,
60.6088052279135,61.1068900781646,61.6049749284156,62.1030597786667,62.6011446289178,
63.0992294791688,63.5973143294198,64.0953991796709,64.5934840299219,65.091568880173,
65.589653730424,65.9734457253856),.UNSPECIFIED.);
#5927=B_SPLINE_CURVE_WITH_KNOTS('',3,(#26642,#26643,#26644,#26645,#26646,
#26647,#26648,#26649,#26650,#26651,#26652,#26653,#26654,#26655,#26656,#26657),
 .UNSPECIFIED.,.F.,.F.,(4,1,1,1,1,1,1,1,1,1,1,1,1,4),(53.4070751110264,
53.4538579690124,53.9519428192634,54.4500276695145,54.9481125197655,55.4461973700166,
55.9442822202676,56.4423670705187,56.9404519207697,57.4385367710208,57.9366216212718,
58.4347064715229,59.430876172025,59.6902604182061),.UNSPECIFIED.);
#5928=B_SPLINE_CURVE_WITH_KNOTS('',3,(#26658,#26659,#26660,#26661,#26662,
#26663,#26664,#26665,#26666,#26667,#26668,#26669,#26670,#26671),
 .UNSPECIFIED.,.F.,.F.,(4,1,1,1,1,1,1,1,1,1,1,4),(53.4070751110264,53.6356173243989,
54.1337021746499,54.631787024901,55.129871875152,56.1260415756541,57.1222112761562,
58.1183809766583,58.6164658269093,59.1145506771604,59.6126355274115,59.690260418206),
 .UNSPECIFIED.);
#5929=B_SPLINE_CURVE_WITH_KNOTS('',3,(#26676,#26677,#26678,#26679,#26680,
#26681,#26682,#26683,#26684,#26685,#26686,#26687,#26688,#26689,#26690,#26691),
 .UNSPECIFIED.,.F.,.F.,(4,1,1,1,1,1,1,1,1,1,1,1,1,4),(47.1238898038469,
47.4768397659998,47.9749246162508,48.4730094665019,48.9710943167529,49.469179167004,
49.967264017255,50.4653488675061,50.9634337177571,51.4615185680082,51.9596034182592,
52.4576882685103,52.9557731187613,53.4070751110264),.UNSPECIFIED.);
#5930=B_SPLINE_CURVE_WITH_KNOTS('',3,(#26692,#26693,#26694,#26695,#26696,
#26697,#26698,#26699,#26700,#26701,#26702,#26703,#26704,#26705,#26706,#26707,
#26708),.UNSPECIFIED.,.F.,.F.,(4,1,1,1,1,1,1,1,1,1,1,1,1,1,4),(47.1238898038469,
47.1605142711352,47.6585991213863,48.1566839716373,48.6547688218884,49.1528536721394,
49.6509385223905,50.1490233726415,50.6471082228926,51.1451930731436,51.6432779233947,
52.1413627736457,52.6394476238968,53.1375324741478,53.4070751110264),
 .UNSPECIFIED.);
#5931=B_SPLINE_CURVE_WITH_KNOTS('',3,(#26713,#26714,#26715,#26716,#26717,
#26718,#26719,#26720,#26721,#26722,#26723,#26724,#26725,#26726,#26727,#26728,
#26729),.UNSPECIFIED.,.F.,.F.,(4,1,1,1,1,1,1,1,1,1,1,1,1,1,4),(40.8407044966673,
41.0017367127361,41.4998215629872,41.9979064132382,42.4959912634893,42.9940761137403,
43.4921609639914,43.9902458142424,44.4883306644935,44.9864155147445,45.4845003649956,
45.9825852152466,46.4806700654977,46.9787549157487,47.1238898038469),
 .UNSPECIFIED.);
#5932=B_SPLINE_CURVE_WITH_KNOTS('',3,(#26730,#26731,#26732,#26733,#26734,
#26735,#26736,#26737,#26738,#26739,#26740,#26741,#26742,#26743,#26744,#26745),
 .UNSPECIFIED.,.F.,.F.,(4,1,1,1,1,1,1,1,1,1,1,1,1,4),(40.8407044966673,
41.1834960681226,41.6815809183737,42.1796657686247,42.6777506188758,43.1758354691268,
43.6739203193779,44.1720051696289,44.67009001988,45.168174870131,45.6662597203821,
46.1643445706331,46.6624294208842,47.1238898038469),.UNSPECIFIED.);
#5933=B_SPLINE_CURVE_WITH_KNOTS('',3,(#26750,#26751,#26752,#26753,#26754,
#26755,#26756,#26757,#26758,#26759,#26760,#26761,#26762,#26763,#26764,#26765),
 .UNSPECIFIED.,.F.,.F.,(4,1,1,1,1,1,1,1,1,1,1,1,1,4),(34.5575191894876,
35.0247185097235,35.5228033599746,36.0208882102256,36.5189730604767,37.0170579107277,
37.5151427609788,38.0132276112299,38.5113124614809,39.0093973117319,39.507482161983,
40.005567012234,40.5036518624851,40.8407044966673),.UNSPECIFIED.);
#5934=B_SPLINE_CURVE_WITH_KNOTS('',3,(#26766,#26767,#26768,#26769,#26770,
#26771,#26772,#26773,#26774,#26775,#26776,#26777,#26778,#26779,#26780,#26781,
#26782),.UNSPECIFIED.,.F.,.F.,(4,1,1,1,1,1,1,1,1,1,1,1,1,1,4),(34.5575191894876,
34.708393014859,35.20647786511,35.7045627153611,36.2026475656121,36.7007324158632,
37.1988172661142,37.6969021163653,38.1949869666163,38.6930718168674,39.1911566671184,
39.6892415173695,40.1873263676205,40.6854112178716,40.8407044966673),
 .UNSPECIFIED.);
#5935=B_SPLINE_CURVE_WITH_KNOTS('',3,(#26787,#26788,#26789,#26790,#26791,
#26792,#26793,#26794,#26795,#26796,#26797,#26798,#26799,#26800,#26801,#26802,
#26803),.UNSPECIFIED.,.F.,.F.,(4,1,1,1,1,1,1,1,1,1,1,1,1,1,4),(28.2743338823081,
28.5496154564599,29.047700306711,29.545785156962,30.0438700072131,30.5419548574641,
31.0400397077152,31.5381245579662,32.0362094082173,32.5342942584683,33.0323791087194,
33.5304639589704,34.0285488092214,34.5266336594725,34.5575191894876),
 .UNSPECIFIED.);
#5936=B_SPLINE_CURVE_WITH_KNOTS('',3,(#26804,#26805,#26806,#26807,#26808,
#26809,#26810,#26811,#26812,#26813,#26814,#26815,#26816,#26817,#26818,#26819),
 .UNSPECIFIED.,.F.,.F.,(4,1,1,1,1,1,1,1,1,1,1,1,1,4),(28.274333882308,28.7313748118464,
29.2294596620974,29.7275445123485,30.2256293625995,30.7237142128506,31.2217990631016,
31.7198839133527,32.2179687636037,32.7160536138548,33.2141384641058,33.7122233143569,
34.2103081646079,34.5575191894876),.UNSPECIFIED.);
#5937=B_SPLINE_CURVE_WITH_KNOTS('',3,(#26824,#26825,#26826,#26827,#26828,
#26829,#26830,#26831,#26832,#26833,#26834,#26835,#26836,#26837,#26838,#26839,
#26840),.UNSPECIFIED.,.F.,.F.,(4,1,1,1,1,1,1,1,1,1,1,1,1,1,4),(21.9911485751285,
22.0745124031963,22.5725972534473,23.0706821036984,23.5687669539494,24.0668518042005,
24.5649366544515,25.0630215047026,25.5611063549536,26.0591912052047,26.5572760554557,
27.0553609057068,27.5534457559578,28.0515306062089,28.2743338823081),
 .UNSPECIFIED.);
#5938=B_SPLINE_CURVE_WITH_KNOTS('',3,(#26841,#26842,#26843,#26844,#26845,
#26846,#26847,#26848,#26849,#26850,#26851,#26852,#26853,#26854,#26855,#26856,
#26857),.UNSPECIFIED.,.F.,.F.,(4,1,1,1,1,1,1,1,1,1,1,1,1,1,4),(21.9911485751285,
22.2562717585827,22.7543566088338,23.2524414590848,23.7505263093359,24.2486111595869,
24.746696009838,25.244780860089,25.7428657103401,26.2409505605911,26.7390354108422,
27.2371202610932,27.7352051113443,28.2332899615953,28.274333882308),
 .UNSPECIFIED.);
#5939=B_SPLINE_CURVE_WITH_KNOTS('',3,(#26862,#26863,#26864,#26865,#26866,
#26867,#26868,#26869,#26870,#26871,#26872,#26873,#26874,#26875,#26876,#26877),
 .UNSPECIFIED.,.F.,.F.,(4,1,1,1,1,1,1,1,1,1,1,1,1,4),(15.7079632679489,
16.0974942001837,16.5955790504347,17.0936639006858,17.5917487509368,18.0898336011879,
18.5879184514389,19.08600330169,19.584088151941,20.0821730021921,20.5802578524431,
21.0783427026942,21.5764275529452,21.9911485751285),.UNSPECIFIED.);
#5940=B_SPLINE_CURVE_WITH_KNOTS('',3,(#26878,#26879,#26880,#26881,#26882,
#26883,#26884,#26885,#26886,#26887,#26888,#26889,#26890,#26891,#26892,#26893,
#26894),.UNSPECIFIED.,.F.,.F.,(4,1,1,1,1,1,1,1,1,1,1,1,1,1,4),(15.7079632679489,
15.7811687053191,16.2792535555702,16.7773384058212,17.2754232560723,17.7735081063233,
18.2715929565744,18.7696778068254,19.2677626570764,19.7658475073275,20.2639323575785,
20.7620172078296,21.2601020580806,21.7581869083317,21.9911485751285),
 .UNSPECIFIED.);
#5941=B_SPLINE_CURVE_WITH_KNOTS('',3,(#26900,#26901,#26902,#26903,#26904,
#26905,#26906,#26907,#26908,#26909,#26910,#26911,#26912,#26913,#26914,#26915),
 .UNSPECIFIED.,.F.,.F.,(4,3,3,3,3,4),(-4.09323272002468,-3.9846788020084,
-3.48659395175735,-2.9885091015063,-2.49042425125525,-2.06652207565086),
 .UNSPECIFIED.);
#5942=B_SPLINE_CURVE_WITH_KNOTS('',3,(#26918,#26919,#26920,#26921,#26922,
#26923,#26924,#26925,#26926,#26927),.UNSPECIFIED.,.F.,.F.,(4,3,3,4),(0.,
0.498084850251037,0.996169700502091,1.11488200921589),.UNSPECIFIED.);
#5943=B_SPLINE_CURVE_WITH_KNOTS('',3,(#26932,#26933,#26934,#26935,#26936,
#26937,#26938,#26939,#26940,#26941,#26942,#26943,#26944,#26945,#26946,#26947,
#26948,#26949,#26950,#26951,#26952,#26953,#26954,#26955,#26956,#26957,#26958,
#26959,#26960,#26961,#26962,#26963,#26964,#26965,#26966,#26967,#26968,#26969,
#26970,#26971),.UNSPECIFIED.,.F.,.F.,(4,3,3,3,3,3,3,3,3,3,3,3,3,4),(-10.3764180272043,
-9.96169700502099,-9.46361215476994,-8.96552730451889,-8.46744245426784,
-7.96935760401679,-7.47127275376574,-6.97318790351469,-6.47510305326364,
-5.97701820301259,-5.47893335276154,-4.98084850251049,-4.48276365225945,
-4.09323272002468),.UNSPECIFIED.);
#5944=B_SPLINE_CURVE_WITH_KNOTS('',3,(#26972,#26973,#26974,#26975,#26976,
#26977,#26978,#26979,#26980,#26981,#26982,#26983,#26984,#26985,#26986,#26987,
#26988,#26989,#26990,#26991,#26992,#26993,#26994,#26995,#26996,#26997,#26998,
#26999,#27000,#27001,#27002,#27003,#27004,#27005,#27006,#27007,#27008,#27009,
#27010,#27011),.UNSPECIFIED.,.F.,.F.,(4,3,3,3,3,3,3,3,3,3,3,3,3,4),(1.11488200921589,
1.49425455075314,1.99233940100419,2.49042425125524,2.98850910150629,3.48659395175734,
3.98467880200839,4.48276365225944,4.98084850251049,5.47893335276154,5.97701820301259,
6.47510305326364,6.97318790351469,7.39806731639547),.UNSPECIFIED.);
#5945=B_SPLINE_CURVE_WITH_KNOTS('',3,(#27016,#27017,#27018,#27019,#27020,
#27021,#27022,#27023,#27024,#27025,#27026,#27027,#27028,#27029,#27030,#27031,
#27032,#27033,#27034,#27035,#27036,#27037,#27038,#27039,#27040,#27041,#27042,
#27043,#27044,#27045,#27046,#27047,#27048,#27049,#27050,#27051,#27052,#27053,
#27054,#27055,#27056,#27057,#27058),.UNSPECIFIED.,.F.,.F.,(4,3,3,3,3,3,
3,3,3,3,3,3,3,3,4),(-16.6596033343839,-16.4368000582846,-15.9387152080336,
-15.4406303577825,-14.9425455075315,-14.4444606572804,-13.9463758070294,
-13.4482909567783,-12.9502061065273,-12.4521212562762,-11.9540364060252,
-11.4559515557741,-10.9578667055231,-10.459781855272,-10.3764180272043),
 .UNSPECIFIED.);
#5946=B_SPLINE_CURVE_WITH_KNOTS('',3,(#27059,#27060,#27061,#27062,#27063,
#27064,#27065,#27066,#27067,#27068,#27069,#27070,#27071,#27072,#27073,#27074,
#27075,#27076,#27077,#27078,#27079,#27080,#27081,#27082,#27083,#27084,#27085,
#27086,#27087,#27088,#27089,#27090,#27091,#27092,#27093,#27094,#27095,#27096,
#27097,#27098,#27099,#27100,#27101),.UNSPECIFIED.,.F.,.F.,(4,3,3,3,3,3,
3,3,3,3,3,3,3,3,4),(7.39806731639547,7.47127275376574,7.96935760401679,
8.46744245426784,8.96552730451889,9.46361215476994,9.96169700502099,10.459781855272,
10.9578667055231,11.4559515557741,11.9540364060252,12.4521212562762,12.9502061065273,
13.4482909567783,13.681252623575),.UNSPECIFIED.);
#5947=B_SPLINE_CURVE_WITH_KNOTS('',3,(#27106,#27107,#27108,#27109,#27110,
#27111,#27112,#27113,#27114,#27115,#27116,#27117,#27118,#27119,#27120,#27121,
#27122,#27123,#27124,#27125,#27126,#27127,#27128,#27129,#27130,#27131,#27132,
#27133,#27134,#27135,#27136,#27137,#27138,#27139,#27140,#27141,#27142,#27143,
#27144,#27145,#27146,#27147,#27148),.UNSPECIFIED.,.F.,.F.,(4,3,3,3,3,3,
3,3,3,3,3,3,3,3,4),(-22.9427886415634,-22.9119031115483,-22.4138182612972,
-21.9157334110462,-21.4176485607951,-20.9195637105441,-20.421478860293,
-19.923394010042,-19.4253091597909,-18.9272243095399,-18.4291394592888,
-17.9310546090378,-17.4329697587867,-16.9348849085357,-16.6596033343839),
 .UNSPECIFIED.);
#5948=B_SPLINE_CURVE_WITH_KNOTS('',3,(#27149,#27150,#27151,#27152,#27153,
#27154,#27155,#27156,#27157,#27158,#27159,#27160,#27161,#27162,#27163,#27164,
#27165,#27166,#27167,#27168,#27169,#27170,#27171,#27172,#27173,#27174,#27175,
#27176,#27177,#27178,#27179,#27180,#27181,#27182,#27183,#27184,#27185,#27186,
#27187,#27188,#27189,#27190,#27191),.UNSPECIFIED.,.F.,.F.,(4,3,3,3,3,3,
3,3,3,3,3,3,3,3,4),(13.681252623575,13.9463758070294,14.4444606572804,14.9425455075315,
15.4406303577825,15.9387152080336,16.4368000582846,16.9348849085357,17.4329697587867,
17.9310546090378,18.4291394592888,18.9272243095399,19.4253091597909,19.923394010042,
19.9644379307546),.UNSPECIFIED.);
#5949=B_SPLINE_CURVE_WITH_KNOTS('',3,(#27196,#27197,#27198,#27199,#27200,
#27201,#27202,#27203,#27204,#27205,#27206,#27207,#27208,#27209,#27210,#27211,
#27212,#27213,#27214,#27215,#27216,#27217,#27218,#27219,#27220,#27221,#27222,
#27223,#27224,#27225,#27226,#27227,#27228,#27229,#27230,#27231,#27232,#27233,
#27234,#27235),.UNSPECIFIED.,.F.,.F.,(4,3,3,3,3,3,3,3,3,3,3,3,3,4),(-29.225973948743,
-28.8889213145609,-28.3908364643098,-27.8927516140588,-27.3946667638077,
-26.8965819135567,-26.3984970633056,-25.9004122130546,-25.4023273628035,
-24.9042425125525,-24.4061576623014,-23.9080728120504,-23.4099879617993,
-22.9427886415634),.UNSPECIFIED.);
#5950=B_SPLINE_CURVE_WITH_KNOTS('',3,(#27236,#27237,#27238,#27239,#27240,
#27241,#27242,#27243,#27244,#27245,#27246,#27247,#27248,#27249,#27250,#27251,
#27252,#27253,#27254,#27255,#27256,#27257,#27258,#27259,#27260,#27261,#27262,
#27263,#27264,#27265,#27266,#27267,#27268,#27269,#27270,#27271,#27272,#27273,
#27274,#27275),.UNSPECIFIED.,.F.,.F.,(4,3,3,3,3,3,3,3,3,3,3,3,3,4),(19.9644379307546,
20.421478860293,20.9195637105441,21.4176485607951,21.9157334110462,22.4138182612972,
22.9119031115483,23.4099879617993,23.9080728120504,24.4061576623014,24.9042425125525,
25.4023273628035,25.9004122130546,26.2476232379342),.UNSPECIFIED.);
#5951=B_SPLINE_CURVE_WITH_KNOTS('',3,(#27280,#27281,#27282,#27283,#27284,
#27285,#27286,#27287,#27288,#27289,#27290,#27291,#27292,#27293,#27294,#27295,
#27296,#27297,#27298,#27299,#27300,#27301,#27302,#27303,#27304,#27305,#27306,
#27307,#27308,#27309,#27310,#27311,#27312,#27313,#27314,#27315,#27316,#27317,
#27318,#27319,#27320,#27321,#27322),.UNSPECIFIED.,.F.,.F.,(4,3,3,3,3,3,
3,3,3,3,3,3,3,3,4),(-35.5091592559226,-35.3640243678245,-34.8659395175735,
-34.3678546673224,-33.8697698170714,-33.3716849668203,-32.8736001165693,
-32.3755152663182,-31.8774304160672,-31.3793455658161,-30.8812607155651,
-30.383175865314,-29.885091015063,-29.3870061648119,-29.225973948743),
 .UNSPECIFIED.);
#5952=B_SPLINE_CURVE_WITH_KNOTS('',3,(#27323,#27324,#27325,#27326,#27327,
#27328,#27329,#27330,#27331,#27332,#27333,#27334,#27335,#27336,#27337,#27338,
#27339,#27340,#27341,#27342,#27343,#27344,#27345,#27346,#27347,#27348,#27349,
#27350,#27351,#27352,#27353,#27354,#27355,#27356,#27357,#27358,#27359,#27360,
#27361,#27362,#27363,#27364,#27365),.UNSPECIFIED.,.F.,.F.,(4,3,3,3,3,3,
3,3,3,3,3,3,3,3,4),(26.2476232379342,26.3984970633056,26.8965819135567,
27.3946667638077,27.8927516140588,28.3908364643098,28.8889213145609,29.3870061648119,
29.885091015063,30.383175865314,30.8812607155651,31.3793455658161,31.8774304160672,
32.3755152663182,32.5308085451138),.UNSPECIFIED.);
#5953=B_SPLINE_CURVE_WITH_KNOTS('',3,(#27370,#27371,#27372,#27373,#27374,
#27375,#27376,#27377,#27378,#27379,#27380,#27381,#27382,#27383,#27384,#27385,
#27386,#27387,#27388,#27389,#27390,#27391,#27392,#27393,#27394,#27395,#27396,
#27397,#27398,#27399,#27400,#27401,#27402,#27403,#27404,#27405,#27406,#27407,
#27408,#27409),.UNSPECIFIED.,.F.,.F.,(4,3,3,3,3,3,3,3,3,3,3,3,3,4),(-41.7923445631022,
-41.3410425708371,-40.842957720586,-40.344872870335,-39.846788020084,-39.3487031698329,
-38.8506183195819,-38.3525334693308,-37.8544486190798,-37.3563637688287,
-36.8582789185777,-36.3601940683266,-35.8621092180756,-35.5091592559226),
 .UNSPECIFIED.);
#5954=B_SPLINE_CURVE_WITH_KNOTS('',3,(#27410,#27411,#27412,#27413,#27414,
#27415,#27416,#27417,#27418,#27419,#27420,#27421,#27422,#27423,#27424,#27425,
#27426,#27427,#27428,#27429,#27430,#27431,#27432,#27433,#27434,#27435,#27436,
#27437,#27438,#27439,#27440,#27441,#27442,#27443,#27444,#27445,#27446,#27447,
#27448,#27449),.UNSPECIFIED.,.F.,.F.,(4,3,3,3,3,3,3,3,3,3,3,3,3,4),(32.5308085451138,
32.8736001165693,33.3716849668203,33.8697698170714,34.3678546673224,34.8659395175735,
35.3640243678245,35.8621092180756,36.3601940683266,36.8582789185777,37.3563637688287,
37.8544486190798,38.3525334693308,38.8139938522934),.UNSPECIFIED.);
#5955=B_SPLINE_CURVE_WITH_KNOTS('',3,(#27454,#27455,#27456,#27457,#27458,
#27459,#27460,#27461,#27462,#27463,#27464,#27465,#27466,#27467,#27468,#27469,
#27470,#27471,#27472,#27473,#27474,#27475,#27476,#27477,#27478,#27479,#27480,
#27481,#27482,#27483,#27484,#27485,#27486,#27487,#27488,#27489,#27490,#27491,
#27492,#27493),.UNSPECIFIED.,.F.,.F.,(4,3,3,3,3,3,3,3,3,3,3,3,3,4),(-48.0755298702818,
-47.8161456241007,-46.8199759235987,-46.3218910733476,-45.8238062230965,
-45.3257213728455,-44.8276365225945,-44.3295516723434,-43.8314668220924,
-43.3333819718413,-42.8352971215903,-42.3372122713392,-41.8391274210882,
-41.7923445631022),.UNSPECIFIED.);
#5956=B_SPLINE_CURVE_WITH_KNOTS('',3,(#27494,#27495,#27496,#27497,#27498,
#27499,#27500,#27501,#27502,#27503,#27504,#27505,#27506,#27507,#27508,#27509,
#27510,#27511,#27512,#27513,#27514,#27515,#27516,#27517,#27518,#27519,#27520,
#27521,#27522,#27523,#27524,#27525,#27526,#27527,#27528,#27529,#27530,#27531,
#27532,#27533,#27534,#27535,#27536),.UNSPECIFIED.,.F.,.F.,(4,3,3,3,3,3,
3,3,3,3,3,3,3,3,4),(38.8139938522934,38.8506183195819,39.3487031698329,
39.846788020084,40.344872870335,40.842957720586,41.3410425708371,41.8391274210882,
42.3372122713392,42.8352971215903,43.3333819718413,43.8314668220923,44.3295516723434,
44.8276365225945,45.097179159473),.UNSPECIFIED.);
#5957=B_SPLINE_CURVE_WITH_KNOTS('',3,(#27541,#27542,#27543,#27544,#27545,
#27546,#27547,#27548,#27549,#27550,#27551,#27552,#27553,#27554,#27555,#27556,
#27557,#27558,#27559,#27560,#27561,#27562,#27563,#27564,#27565,#27566,#27567,
#27568,#27569,#27570,#27571,#27572,#27573,#27574,#27575,#27576,#27577),
 .UNSPECIFIED.,.F.,.F.,(4,3,3,3,3,3,3,3,3,3,3,3,4),(-54.3587151774614,-54.2912486773644,
-53.7931638271133,-53.2950789768623,-52.7969941266112,-52.2989092763602,
-51.8008244261091,-51.3027395758581,-50.804654725607,-50.306569875356,-49.808485025105,
-48.8123153246028,-48.0755298702818),.UNSPECIFIED.);
#5958=B_SPLINE_CURVE_WITH_KNOTS('',3,(#27578,#27579,#27580,#27581,#27582,
#27583,#27584,#27585,#27586,#27587,#27588,#27589,#27590,#27591,#27592,#27593,
#27594,#27595,#27596,#27597,#27598,#27599,#27600,#27601,#27602,#27603,#27604,
#27605,#27606,#27607,#27608,#27609,#27610,#27611),.UNSPECIFIED.,.F.,.F.,
(4,3,3,3,3,3,3,3,3,3,3,4),(45.097179159473,45.3257213728455,45.8238062230965,
46.3218910733476,46.8199759235987,47.8161456241007,48.8123153246028,49.808485025105,
50.306569875356,50.8046547256071,51.3027395758581,51.3803644666526),
 .UNSPECIFIED.);
#5959=B_SPLINE_CURVE_WITH_KNOTS('',3,(#27616,#27617,#27618,#27619,#27620,
#27621,#27622,#27623,#27624,#27625,#27626,#27627,#27628,#27629,#27630,#27631,
#27632,#27633,#27634,#27635,#27636,#27637,#27638,#27639,#27640,#27641,#27642,
#27643,#27644,#27645,#27646,#27647,#27648,#27649,#27650,#27651,#27652,#27653,
#27654,#27655),.UNSPECIFIED.,.F.,.F.,(4,3,3,3,3,3,3,3,3,3,3,3,3,4),(-60.641900484641,
-60.268266880377,-59.7701820301259,-59.2720971798749,-58.7740123296238,
-58.2759274793728,-57.7778426291217,-57.2797577788707,-56.7816729286196,
-56.2835880783686,-55.7855032281175,-55.2874183778665,-54.7893335276154,
-54.3587151774614),.UNSPECIFIED.);
#5960=B_SPLINE_CURVE_WITH_KNOTS('',3,(#27656,#27657,#27658,#27659,#27660,
#27661,#27662,#27663,#27664,#27665,#27666,#27667,#27668,#27669,#27670,#27671,
#27672,#27673,#27674,#27675,#27676,#27677,#27678,#27679,#27680,#27681,#27682,
#27683,#27684,#27685,#27686,#27687,#27688,#27689,#27690,#27691,#27692,#27693,
#27694,#27695),.UNSPECIFIED.,.F.,.F.,(4,3,3,3,3,3,3,3,3,3,3,3,3,4),(51.3803644666526,
51.8008244261092,52.2989092763602,52.7969941266112,53.2950789768623,53.7931638271133,
54.2912486773644,54.7893335276154,55.2874183778665,55.7855032281175,56.2835880783686,
56.7816729286196,57.2797577788707,57.6635497738322),.UNSPECIFIED.);
#5961=B_SPLINE_CURVE_WITH_KNOTS('',3,(#27700,#27701,#27702,#27703,#27704,
#27705,#27706,#27707,#27708,#27709,#27710,#27711,#27712,#27713,#27714,#27715,
#27716,#27717,#27718,#27719,#27720,#27721,#27722,#27723,#27724,#27725,#27726,
#27727,#27728,#27729,#27730,#27731,#27732,#27733,#27734,#27735,#27736,#27737,
#27738,#27739,#27740,#27741,#27742),.UNSPECIFIED.,.F.,.F.,(4,3,3,3,3,3,
3,3,3,3,3,3,3,3,4),(-66.9250857918206,-66.7433699336406,-66.2452850833896,
-65.7472002331385,-65.2491153828875,-64.7510305326364,-64.2529456823854,
-63.7548608321343,-63.2567759818833,-62.7586911316322,-62.2606062813812,
-61.7625214311301,-61.2644365808791,-60.766351730628,-60.641900484641),
 .UNSPECIFIED.);
#5962=B_SPLINE_CURVE_WITH_KNOTS('',3,(#27743,#27744,#27745,#27746,#27747,
#27748,#27749,#27750,#27751,#27752,#27753,#27754,#27755,#27756,#27757,#27758,
#27759,#27760,#27761,#27762,#27763,#27764,#27765,#27766,#27767,#27768,#27769,
#27770,#27771,#27772,#27773,#27774,#27775,#27776,#27777,#27778,#27779,#27780,
#27781,#27782,#27783,#27784,#27785),.UNSPECIFIED.,.F.,.F.,(4,3,3,3,3,3,
3,3,3,3,3,3,3,3,4),(57.6635497738322,57.7778426291217,58.2759274793728,
58.7740123296238,59.2720971798749,59.7701820301259,60.268266880377,60.766351730628,
61.2644365808791,61.7625214311301,62.2606062813812,62.7586911316322,63.2567759818833,
63.7548608321343,63.9467350810118),.UNSPECIFIED.);
#5963=B_SPLINE_CURVE_WITH_KNOTS('',3,(#27790,#27791,#27792,#27793,#27794,
#27795,#27796,#27797,#27798,#27799,#27800,#27801,#27802,#27803,#27804,#27805,
#27806,#27807,#27808,#27809,#27810,#27811,#27812,#27813,#27814,#27815,#27816,
#27817,#27818,#27819,#27820,#27821,#27822,#27823,#27824,#27825,#27826,#27827,
#27828,#27829),.UNSPECIFIED.,.F.,.F.,(4,3,3,3,3,3,3,3,3,3,3,3,3,4),(-73.2082710990002,
-72.7203881366532,-72.2223032864022,-71.7242184361511,-71.2261335859001,
-70.728048735649,-70.229963885398,-69.7318790351469,-69.2337941848959,-68.7357093346448,
-68.2376244843938,-67.7395396341427,-67.2414547838917,-66.9250857918206),
 .UNSPECIFIED.);
#5964=B_SPLINE_CURVE_WITH_KNOTS('',3,(#27830,#27831,#27832,#27833,#27834,
#27835,#27836,#27837,#27838,#27839,#27840,#27841,#27842,#27843,#27844,#27845,
#27846,#27847,#27848,#27849,#27850,#27851,#27852,#27853,#27854,#27855,#27856,
#27857,#27858,#27859,#27860,#27861,#27862,#27863,#27864,#27865,#27866,#27867,
#27868,#27869),.UNSPECIFIED.,.F.,.F.,(4,3,3,3,3,3,3,3,3,3,3,3,3,4),(63.9467350810118,
64.2529456823854,64.7510305326364,65.2491153828875,65.7472002331385,66.2452850833896,
66.7433699336406,67.2414547838917,67.7395396341427,68.2376244843938,68.7357093346448,
69.2337941848959,69.7318790351469,70.2299203881914),.UNSPECIFIED.);
#5965=B_SPLINE_CURVE_WITH_KNOTS('',3,(#27874,#27875,#27876,#27877,#27878,
#27879,#27880,#27881,#27882,#27883,#27884,#27885,#27886,#27887,#27888,#27889,
#27890,#27891,#27892,#27893,#27894,#27895,#27896,#27897,#27898,#27899,#27900,
#27901,#27902,#27903,#27904,#27905,#27906,#27907,#27908,#27909,#27910,#27911,
#27912,#27913,#27914,#27915,#27916),.UNSPECIFIED.,.F.,.F.,(4,3,3,3,3,3,
3,3,3,3,3,3,3,3,4),(-79.4914564061798,-79.1954911899169,-78.6974063396658,
-78.1993214894148,-77.7012366391637,-77.2031517889127,-76.7050669386616,
-76.2069820884106,-75.7088972381595,-75.2108123879085,-74.7127275376574,
-74.2146426874064,-73.7165578371553,-73.2184729869043,-73.2082710990002),
 .UNSPECIFIED.);
#5966=B_SPLINE_CURVE_WITH_KNOTS('',3,(#27917,#27918,#27919,#27920,#27921,
#27922,#27923,#27924,#27925,#27926,#27927,#27928,#27929,#27930,#27931,#27932,
#27933,#27934,#27935,#27936,#27937,#27938,#27939,#27940,#27941,#27942,#27943,
#27944,#27945,#27946,#27947,#27948,#27949,#27950,#27951,#27952,#27953,#27954,
#27955,#27956),.UNSPECIFIED.,.F.,.F.,(4,3,3,3,3,3,3,3,3,3,3,3,3,4),(70.2299203881914,
70.728048735649,71.2261335859001,71.7242184361511,72.2223032864022,72.7203881366532,
73.2184729869043,73.7165578371553,74.2146426874064,74.7127275376574,75.2108123879085,
75.7088972381595,76.2069820884106,76.513105695371),.UNSPECIFIED.);
#5967=B_SPLINE_CURVE_WITH_KNOTS('',3,(#27961,#27962,#27963,#27964,#27965,
#27966,#27967,#27968,#27969,#27970,#27971,#27972,#27973,#27974,#27975,#27976,
#27977,#27978,#27979,#27980,#27981,#27982,#27983,#27984,#27985,#27986,#27987,
#27988,#27989,#27990,#27991,#27992,#27993,#27994,#27995,#27996,#27997,#27998,
#27999,#28000,#28001,#28002,#28003),.UNSPECIFIED.,.F.,.F.,(4,3,3,3,3,3,
3,3,3,3,3,3,3,3,4),(-85.7746417133593,-85.6705942431805,-85.1725093929295,
-84.6744245426784,-84.1763396924274,-83.6782548421763,-83.1801699919253,
-82.6820851416742,-82.1840002914232,-81.6859154411721,-81.1878305909211,
-80.68974574067,-80.191660890419,-79.6935760401679,-79.4914564061798),
 .UNSPECIFIED.);
#5968=B_SPLINE_CURVE_WITH_KNOTS('',3,(#28004,#28005,#28006,#28007,#28008,
#28009,#28010,#28011,#28012,#28013,#28014,#28015,#28016,#28017,#28018,#28019,
#28020,#28021,#28022,#28023,#28024,#28025,#28026,#28027,#28028,#28029,#28030,
#28031,#28032,#28033,#28034,#28035,#28036,#28037,#28038,#28039,#28040,#28041,
#28042,#28043,#28044,#28045,#28046),.UNSPECIFIED.,.F.,.F.,(4,3,3,3,3,3,
3,3,3,3,3,3,3,3,4),(76.513105695371,76.7050669386616,77.2031517889126,77.7012366391637,
78.1993214894147,78.6974063396658,79.1954911899169,79.6935760401679,80.1916608904189,
80.68974574067,81.1878305909211,81.6859154411721,82.1840002914231,82.6820851416742,
82.7962910025506),.UNSPECIFIED.);
#5969=B_SPLINE_CURVE_WITH_KNOTS('',3,(#28051,#28052,#28053,#28054,#28055,
#28056,#28057,#28058,#28059,#28060,#28061,#28062,#28063,#28064,#28065,#28066,
#28067,#28068,#28069,#28070,#28071,#28072,#28073,#28074,#28075,#28076,#28077,
#28078,#28079,#28080,#28081,#28082,#28083,#28084,#28085,#28086,#28087,#28088,
#28089,#28090),.UNSPECIFIED.,.F.,.F.,(4,3,3,3,3,3,3,3,3,3,3,3,3,4),(-92.057827020539,
-91.6476124461931,-91.1495275959421,-90.651442745691,-90.15335789544,-89.6552730451889,
-89.1571881949379,-88.6591033446868,-88.1610184944358,-87.6629336441847,
-87.1648487939337,-86.6667639436826,-86.1686790934316,-85.7746417133593),
 .UNSPECIFIED.);
#5970=B_SPLINE_CURVE_WITH_KNOTS('',3,(#28091,#28092,#28093,#28094,#28095,
#28096,#28097,#28098,#28099,#28100,#28101,#28102,#28103,#28104,#28105,#28106,
#28107,#28108,#28109,#28110,#28111,#28112,#28113,#28114,#28115,#28116,#28117,
#28118,#28119,#28120,#28121,#28122,#28123,#28124,#28125,#28126,#28127,#28128,
#28129,#28130),.UNSPECIFIED.,.F.,.F.,(4,3,3,3,3,3,3,3,3,3,3,3,3,4),(82.7962910025506,
83.1801699919252,83.6782548421763,84.1763396924274,84.6744245426784,85.1725093929295,
85.6705942431805,86.1686790934316,86.6667639436826,87.1648487939337,87.6629336441847,
88.1610184944358,88.6591033446868,89.0794763097302),.UNSPECIFIED.);
#5971=B_SPLINE_CURVE_WITH_KNOTS('',3,(#28136,#28137,#28138,#28139,#28140,
#28141,#28142,#28143,#28144),.UNSPECIFIED.,.F.,.F.,(4,1,1,1,1,1,4),(103.672557568463,
103.760427844368,104.258512694619,104.75659754487,105.254682395122,105.752767245373,
106.176669420977),.UNSPECIFIED.);
#5972=B_SPLINE_CURVE_WITH_KNOTS('',3,(#28147,#28148,#28149,#28150,#28151,
#28152),.UNSPECIFIED.,.F.,.F.,(4,1,1,4),(103.672557568463,103.942187199755,
104.440272050006,104.938356900257),.UNSPECIFIED.);
#5973=B_SPLINE_CURVE_WITH_KNOTS('',3,(#28157,#28158,#28159,#28160,#28161,
#28162,#28163,#28164,#28165,#28166,#28167,#28168,#28169,#28170,#28171,#28172),
 .UNSPECIFIED.,.F.,.F.,(4,1,1,1,1,1,1,1,1,1,1,1,1,4),(97.3893722612836,
97.7834096413558,98.2814944916068,98.7795793418579,99.2776641921089,99.77574904236,
100.273833892611,100.771918742862,101.270003593113,101.768088443364,102.266173293615,
102.764258143866,103.262342994117,103.672557568463),.UNSPECIFIED.);
#5974=B_SPLINE_CURVE_WITH_KNOTS('',3,(#28173,#28174,#28175,#28176,#28177,
#28178,#28179,#28180,#28181,#28182,#28183,#28184,#28185,#28186,#28187,#28188,
#28189),.UNSPECIFIED.,.F.,.F.,(4,1,1,1,1,1,1,1,1,1,1,1,1,1,4),(97.3893722612835,
97.4670841464912,97.9651689967422,98.4632538469933,98.9613386972443,99.4594235474954,
99.9575083977464,100.455593247997,100.953678098249,101.4517629485,101.949847798751,
102.447932649002,102.946017499253,103.444102349504,103.672557568463),
 .UNSPECIFIED.);
#5975=B_SPLINE_CURVE_WITH_KNOTS('',3,(#28194,#28195,#28196,#28197,#28198,
#28199,#28200,#28201,#28202,#28203,#28204,#28205,#28206,#28207,#28208,#28209,
#28210),.UNSPECIFIED.,.F.,.F.,(4,1,1,1,1,1,1,1,1,1,1,1,1,1,4),(91.106186954104,
91.3083065880921,91.8063914383432,92.3044762885942,92.8025611388453,93.3006459890963,
93.7987308393474,94.2968156895984,94.7949005398495,95.2929853901005,95.7910702403516,
96.2891550906026,96.7872399408537,97.2853247911047,97.3893722612836),
 .UNSPECIFIED.);
#5976=B_SPLINE_CURVE_WITH_KNOTS('',3,(#28211,#28212,#28213,#28214,#28215,
#28216,#28217,#28218,#28219,#28220,#28221,#28222,#28223,#28224,#28225,#28226),
 .UNSPECIFIED.,.F.,.F.,(4,1,1,1,1,1,1,1,1,1,1,1,1,4),(91.106186954104,91.4900659434786,
91.9881507937296,92.4862356439807,92.9843204942317,93.4824053444828,93.9804901947338,
94.4785750449849,94.9766598952359,95.474744745487,95.972829595738,96.4709144459891,
96.9689992962401,97.3893722612835),.UNSPECIFIED.);
#5977=B_SPLINE_CURVE_WITH_KNOTS('',3,(#28231,#28232,#28233,#28234,#28235,
#28236,#28237,#28238,#28239,#28240,#28241,#28242,#28243,#28244,#28245,#28246,
#28247),.UNSPECIFIED.,.F.,.F.,(4,1,1,1,1,1,1,1,1,1,1,1,1,1,4),(84.8230016469244,
84.8332035348285,85.3312883850795,85.8293732353306,86.3274580855816,86.8255429358327,
87.3236277860837,87.8217126363348,88.3197974865858,88.8178823368369,89.3159671870879,
89.814052037339,90.31213688759,90.8102217378411,91.106186954104),
 .UNSPECIFIED.);
#5978=B_SPLINE_CURVE_WITH_KNOTS('',3,(#28248,#28249,#28250,#28251,#28252,
#28253,#28254,#28255,#28256,#28257,#28258,#28259,#28260,#28261,#28262,#28263,
#28264),.UNSPECIFIED.,.F.,.F.,(4,1,1,1,1,1,1,1,1,1,1,1,1,1,4),(84.8230016469244,
85.0149628902149,85.513047740466,86.011132590717,86.5092174409681,87.0073022912191,
87.5053871414702,88.0034719917212,88.5015568419723,88.9996416922233,89.4977265424744,
89.9958113927254,90.4938962429765,90.9919810932275,91.106186954104),
 .UNSPECIFIED.);
#5979=B_SPLINE_CURVE_WITH_KNOTS('',3,(#28269,#28270,#28271,#28272,#28273,
#28274,#28275,#28276,#28277,#28278,#28279,#28280,#28281,#28282,#28283,#28284),
 .UNSPECIFIED.,.F.,.F.,(4,1,1,1,1,1,1,1,1,1,1,1,1,4),(78.5398163397448,
78.8561853318159,79.3542701820669,79.852355032318,80.350439882569,80.8485247328201,
81.3466095830711,81.8446944333222,82.3427792835732,82.8408641338243,83.3389489840753,
83.8370338343264,84.3351186845774,84.8230016469244),.UNSPECIFIED.);
#5980=B_SPLINE_CURVE_WITH_KNOTS('',3,(#28285,#28286,#28287,#28288,#28289,
#28290,#28291,#28292,#28293,#28294,#28295,#28296,#28297,#28298,#28299,#28300,
#28301),.UNSPECIFIED.,.F.,.F.,(4,1,1,1,1,1,1,1,1,1,1,1,1,1,4),(78.5398163397448,
78.5398598369513,79.0379446872024,79.5360295374534,80.0341143877044,80.5321992379555,
81.0302840882066,81.5283689384576,82.0264537887087,82.5245386389597,83.0226234892107,
83.5207083394618,84.0187931897129,84.5168780399639,84.8230016469244),
 .UNSPECIFIED.);
#5981=B_SPLINE_CURVE_WITH_KNOTS('',3,(#28306,#28307,#28308,#28309,#28310,
#28311,#28312,#28313,#28314,#28315,#28316,#28317,#28318,#28319,#28320,#28321,
#28322),.UNSPECIFIED.,.F.,.F.,(4,1,1,1,1,1,1,1,1,1,1,1,1,1,4),(72.2566310325652,
72.3810822785522,72.8791671288033,73.3772519790543,73.8753368293054,74.3734216795564,
74.8715065298075,75.3695913800585,75.8676762303096,76.3657610805606,76.8638459308117,
77.3619307810627,77.8600156313138,78.3581004815648,78.5398163397448),
 .UNSPECIFIED.);
#5982=B_SPLINE_CURVE_WITH_KNOTS('',3,(#28323,#28324,#28325,#28326,#28327,
#28328,#28329,#28330,#28331,#28332,#28333,#28334,#28335,#28336,#28337,#28338),
 .UNSPECIFIED.,.F.,.F.,(4,1,1,1,1,1,1,1,1,1,1,1,1,4),(72.2566310325652,
72.5628416339387,73.0609264841898,73.5590113344408,74.0570961846919,74.5551810349429,
75.053265885194,75.551350735445,76.0494355856961,76.5475204359471,77.0456052861982,
77.5436901364492,78.0417749867003,78.5398163397448),.UNSPECIFIED.);
#5983=B_SPLINE_CURVE_WITH_KNOTS('',3,(#28343,#28344,#28345,#28346,#28347,
#28348,#28349,#28350,#28351,#28352,#28353,#28354,#28355,#28356,#28357,#28358),
 .UNSPECIFIED.,.F.,.F.,(4,1,1,1,1,1,1,1,1,1,1,1,1,4),(65.9734457253856,
66.4040640755397,66.9021489257907,67.4002337760417,67.8983186262928,68.3964034765438,
68.8944883267949,69.3925731770459,69.890658027297,70.388742877548,70.8868277277991,
71.3849125780501,71.8829974283012,72.2566310325652),.UNSPECIFIED.);
#5984=B_SPLINE_CURVE_WITH_KNOTS('',3,(#28359,#28360,#28361,#28362,#28363,
#28364,#28365,#28366,#28367,#28368,#28369,#28370,#28371,#28372,#28373,#28374,
#28375),.UNSPECIFIED.,.F.,.F.,(4,1,1,1,1,1,1,1,1,1,1,1,1,1,4),(65.9734457253856,
66.0877385806751,66.5858234309261,67.0839082811772,67.5819931314282,68.0800779816793,
68.5781628319303,69.0762476821814,69.5743325324324,70.0724173826835,70.5705022329345,
71.0685870831856,71.5666719334366,72.0647567836877,72.2566310325652),
 .UNSPECIFIED.);
#5985=B_SPLINE_CURVE_WITH_KNOTS('',3,(#28380,#28381,#28382,#28383,#28384,
#28385,#28386,#28387,#28388,#28389,#28390,#28391,#28392,#28393,#28394),
 .UNSPECIFIED.,.F.,.F.,(4,1,1,1,1,1,1,1,1,1,1,1,4),(59.690260418206,60.427045872527,
61.4232155730292,61.9213004232802,62.4193852735312,62.9174701237823,63.4155549740333,
63.9136398242844,64.4117246745354,64.9098095247865,65.4078943750375,65.9059792252886,
65.9734457253856),.UNSPECIFIED.);
#5986=B_SPLINE_CURVE_WITH_KNOTS('',3,(#28395,#28396,#28397,#28398,#28399,
#28400,#28401,#28402,#28403,#28404,#28405,#28406,#28407,#28408,#28409,#28410),
 .UNSPECIFIED.,.F.,.F.,(4,1,1,1,1,1,1,1,1,1,1,1,1,4),(59.690260418206,60.1107203776625,
60.6088052279135,61.1068900781646,61.6049749284156,62.1030597786667,62.6011446289177,
63.0992294791688,63.5973143294198,64.0953991796709,64.5934840299219,65.091568880173,
65.589653730424,65.9734457253856),.UNSPECIFIED.);
#5987=B_SPLINE_CURVE_WITH_KNOTS('',3,(#28415,#28416,#28417,#28418,#28419,
#28420,#28421,#28422,#28423,#28424,#28425,#28426,#28427,#28428,#28429,#28430),
 .UNSPECIFIED.,.F.,.F.,(4,1,1,1,1,1,1,1,1,1,1,1,1,4),(53.4070751110264,
53.4538579690124,53.9519428192634,54.4500276695145,54.9481125197655,55.4461973700166,
55.9442822202676,56.4423670705187,56.9404519207697,57.4385367710208,57.9366216212718,
58.4347064715229,59.430876172025,59.690260418206),.UNSPECIFIED.);
#5988=B_SPLINE_CURVE_WITH_KNOTS('',3,(#28431,#28432,#28433,#28434,#28435,
#28436,#28437,#28438,#28439,#28440,#28441,#28442,#28443,#28444),
 .UNSPECIFIED.,.F.,.F.,(4,1,1,1,1,1,1,1,1,1,1,4),(53.4070751110264,53.6356173243988,
54.1337021746499,54.6317870249009,55.129871875152,56.1260415756541,57.1222112761562,
58.1183809766583,58.6164658269093,59.1145506771604,59.6126355274114,59.690260418206),
 .UNSPECIFIED.);
#5989=B_SPLINE_CURVE_WITH_KNOTS('',3,(#28449,#28450,#28451,#28452,#28453,
#28454,#28455,#28456,#28457,#28458,#28459,#28460,#28461,#28462,#28463,#28464),
 .UNSPECIFIED.,.F.,.F.,(4,1,1,1,1,1,1,1,1,1,1,1,1,4),(47.1238898038469,
47.4768397659998,47.9749246162508,48.4730094665019,48.9710943167529,49.469179167004,
49.967264017255,50.4653488675061,50.9634337177571,51.4615185680082,51.9596034182592,
52.4576882685103,52.9557731187613,53.4070751110264),.UNSPECIFIED.);
#5990=B_SPLINE_CURVE_WITH_KNOTS('',3,(#28465,#28466,#28467,#28468,#28469,
#28470,#28471,#28472,#28473,#28474,#28475,#28476,#28477,#28478,#28479,#28480,
#28481),.UNSPECIFIED.,.F.,.F.,(4,1,1,1,1,1,1,1,1,1,1,1,1,1,4),(47.1238898038468,
47.1605142711352,47.6585991213862,48.1566839716373,48.6547688218883,49.1528536721394,
49.6509385223904,50.1490233726415,50.6471082228925,51.1451930731436,51.6432779233946,
52.1413627736457,52.6394476238967,53.1375324741478,53.4070751110264),
 .UNSPECIFIED.);
#5991=B_SPLINE_CURVE_WITH_KNOTS('',3,(#28486,#28487,#28488,#28489,#28490,
#28491,#28492,#28493,#28494,#28495,#28496,#28497,#28498,#28499,#28500,#28501,
#28502),.UNSPECIFIED.,.F.,.F.,(4,1,1,1,1,1,1,1,1,1,1,1,1,1,4),(40.8407044966673,
41.0017367127361,41.4998215629872,41.9979064132382,42.4959912634893,42.9940761137403,
43.4921609639914,43.9902458142424,44.4883306644935,44.9864155147445,45.4845003649956,
45.9825852152466,46.4806700654977,46.9787549157487,47.1238898038469),
 .UNSPECIFIED.);
#5992=B_SPLINE_CURVE_WITH_KNOTS('',3,(#28503,#28504,#28505,#28506,#28507,
#28508,#28509,#28510,#28511,#28512,#28513,#28514,#28515,#28516,#28517,#28518),
 .UNSPECIFIED.,.F.,.F.,(4,1,1,1,1,1,1,1,1,1,1,1,1,4),(40.8407044966672,
41.1834960681226,41.6815809183737,42.1796657686247,42.6777506188757,43.1758354691268,
43.6739203193778,44.1720051696289,44.67009001988,45.168174870131,45.666259720382,
46.1643445706331,46.6624294208841,47.1238898038468),.UNSPECIFIED.);
#5993=B_SPLINE_CURVE_WITH_KNOTS('',3,(#28523,#28524,#28525,#28526,#28527,
#28528,#28529,#28530,#28531,#28532,#28533,#28534,#28535,#28536,#28537,#28538),
 .UNSPECIFIED.,.F.,.F.,(4,1,1,1,1,1,1,1,1,1,1,1,1,4),(34.5575191894877,
35.0247185097235,35.5228033599746,36.0208882102256,36.5189730604767,37.0170579107277,
37.5151427609788,38.0132276112298,38.5113124614809,39.0093973117319,39.507482161983,
40.005567012234,40.5036518624851,40.8407044966673),.UNSPECIFIED.);
#5994=B_SPLINE_CURVE_WITH_KNOTS('',3,(#28539,#28540,#28541,#28542,#28543,
#28544,#28545,#28546,#28547,#28548,#28549,#28550,#28551,#28552,#28553,#28554,
#28555),.UNSPECIFIED.,.F.,.F.,(4,1,1,1,1,1,1,1,1,1,1,1,1,1,4),(34.5575191894876,
34.708393014859,35.20647786511,35.7045627153611,36.2026475656121,36.7007324158632,
37.1988172661142,37.6969021163653,38.1949869666163,38.6930718168674,39.1911566671184,
39.6892415173695,40.1873263676205,40.6854112178715,40.8407044966672),
 .UNSPECIFIED.);
#5995=B_SPLINE_CURVE_WITH_KNOTS('',3,(#28560,#28561,#28562,#28563,#28564,
#28565,#28566,#28567,#28568,#28569,#28570,#28571,#28572,#28573,#28574,#28575,
#28576),.UNSPECIFIED.,.F.,.F.,(4,1,1,1,1,1,1,1,1,1,1,1,1,1,4),(28.2743338823081,
28.5496154564599,29.0477003067109,29.545785156962,30.043870007213,30.5419548574641,
31.0400397077151,31.5381245579662,32.0362094082172,32.5342942584683,33.0323791087193,
33.5304639589704,34.0285488092214,34.5266336594725,34.5575191894877),
 .UNSPECIFIED.);
#5996=B_SPLINE_CURVE_WITH_KNOTS('',3,(#28577,#28578,#28579,#28580,#28581,
#28582,#28583,#28584,#28585,#28586,#28587,#28588,#28589,#28590,#28591,#28592),
 .UNSPECIFIED.,.F.,.F.,(4,1,1,1,1,1,1,1,1,1,1,1,1,4),(28.2743338823081,
28.7313748118464,29.2294596620974,29.7275445123485,30.2256293625995,30.7237142128506,
31.2217990631016,31.7198839133527,32.2179687636037,32.7160536138548,33.2141384641058,
33.7122233143569,34.2103081646079,34.5575191894876),.UNSPECIFIED.);
#5997=B_SPLINE_CURVE_WITH_KNOTS('',3,(#28597,#28598,#28599,#28600,#28601,
#28602,#28603,#28604,#28605,#28606,#28607,#28608,#28609,#28610,#28611,#28612,
#28613),.UNSPECIFIED.,.F.,.F.,(4,1,1,1,1,1,1,1,1,1,1,1,1,1,4),(21.9911485751285,
22.0745124031962,22.5725972534473,23.0706821036983,23.5687669539494,24.0668518042004,
24.5649366544515,25.0630215047025,25.5611063549536,26.0591912052046,26.5572760554557,
27.0553609057067,27.5534457559578,28.0515306062088,28.2743338823081),
 .UNSPECIFIED.);
#5998=B_SPLINE_CURVE_WITH_KNOTS('',3,(#28614,#28615,#28616,#28617,#28618,
#28619,#28620,#28621,#28622,#28623,#28624,#28625,#28626,#28627,#28628,#28629,
#28630),.UNSPECIFIED.,.F.,.F.,(4,1,1,1,1,1,1,1,1,1,1,1,1,1,4),(21.9911485751285,
22.2562717585827,22.7543566088338,23.2524414590848,23.7505263093359,24.2486111595869,
24.746696009838,25.244780860089,25.7428657103401,26.2409505605911,26.7390354108422,
27.2371202610932,27.7352051113443,28.2332899615953,28.2743338823081),
 .UNSPECIFIED.);
#5999=B_SPLINE_CURVE_WITH_KNOTS('',3,(#28635,#28636,#28637,#28638,#28639,
#28640,#28641,#28642,#28643,#28644,#28645,#28646,#28647,#28648,#28649,#28650),
 .UNSPECIFIED.,.F.,.F.,(4,1,1,1,1,1,1,1,1,1,1,1,1,4),(15.7079632679489,
16.0974942001837,16.5955790504347,17.0936639006858,17.5917487509368,18.0898336011878,
18.5879184514389,19.0860033016899,19.584088151941,20.082173002192,20.5802578524431,
21.0783427026941,21.5764275529452,21.9911485751285),.UNSPECIFIED.);
#6000=B_SPLINE_CURVE_WITH_KNOTS('',3,(#28651,#28652,#28653,#28654,#28655,
#28656,#28657,#28658,#28659,#28660,#28661,#28662,#28663,#28664,#28665,#28666,
#28667),.UNSPECIFIED.,.F.,.F.,(4,1,1,1,1,1,1,1,1,1,1,1,1,1,4),(15.7079632679489,
15.7811687053191,16.2792535555701,16.7773384058212,17.2754232560722,17.7735081063233,
18.2715929565743,18.7696778068254,19.2677626570764,19.7658475073275,20.2639323575785,
20.7620172078296,21.2601020580806,21.7581869083317,21.9911485751285),
 .UNSPECIFIED.);
#6001=B_SPLINE_CURVE_WITH_KNOTS('',3,(#28670,#28671,#28672,#28673,#28674,
#28675,#28676,#28677,#28678,#28679,#28680,#28681,#28682,#28683,#28684,#28685,
#28686,#28687,#28688,#28689,#28690,#28691,#28692,#28693,#28694,#28695,#28696,
#28697,#28698,#28699,#28700,#28701,#28702,#28703,#28704,#28705,#28706,#28707,
#28708,#28709,#28710,#28711,#28712,#28713,#28714,#28715,#28716,#28717,#28718,
#28719,#28720,#28721,#28722,#28723,#28724,#28725,#28726,#28727,#28728,#28729,
#28730,#28731,#28732,#28733,#28734,#28735,#28736,#28737,#28738,#28739,#28740,
#28741,#28742,#28743,#28744,#28745,#28746,#28747,#28748,#28749,#28750,#28751,
#28752,#28753,#28754,#28755,#28756,#28757,#28758,#28759,#28760,#28761,#28762,
#28763,#28764,#28765,#28766,#28767,#28768,#28769,#28770,#28771,#28772,#28773,
#28774,#28775,#28776,#28777,#28778,#28779,#28780,#28781),.UNSPECIFIED.,
 .F.,.F.,(4,3,3,3,3,3,3,3,3,3,3,3,3,3,3,3,3,3,3,3,3,3,3,3,3,3,3,3,3,3,3,
3,3,3,3,3,3,4),(-0.937740963081762,-0.907140654471692,-0.869270994512239,
-0.847580464190145,-0.836481370332155,-0.829351939903567,-0.823129304558617,
-0.784196549339193,-0.745021726803261,-0.731277450917006,-0.71832202012087,
-0.712280445222016,-0.695746751935488,-0.656667790671875,-0.616960744636697,
-0.581187597295744,-0.55435773679003,-0.548462240506954,-0.542574359443091,
-0.501604130349,-0.473868155272887,-0.433137517704096,-0.392064137358273,
-0.380617560497555,-0.373704777408693,-0.367641533845849,-0.325920769696254,
-0.283682092026838,-0.241892561201202,-0.211655991051052,-0.198277640892043,
-0.190678095127374,-0.184988742540942,-0.142742067998012,-0.0995960223031999,
-0.0562915317555258,-0.0133559795731416,0.),.UNSPECIFIED.);
#6002=B_SPLINE_CURVE_WITH_KNOTS('',3,(#28786,#28787,#28788,#28789,#28790,
#28791,#28792,#28793,#28794,#28795,#28796,#28797,#28798,#28799,#28800,#28801,
#28802,#28803,#28804,#28805,#28806,#28807,#28808,#28809,#28810,#28811,#28812,
#28813,#28814,#28815,#28816,#28817,#28818,#28819,#28820,#28821,#28822,#28823,
#28824,#28825,#28826,#28827,#28828,#28829,#28830,#28831,#28832,#28833,#28834,
#28835,#28836,#28837,#28838,#28839,#28840,#28841,#28842,#28843,#28844,#28845,
#28846,#28847,#28848,#28849,#28850,#28851,#28852,#28853,#28854,#28855,#28856,
#28857,#28858,#28859,#28860,#28861,#28862,#28863,#28864,#28865,#28866,#28867,
#28868,#28869,#28870,#28871,#28872,#28873,#28874,#28875,#28876,#28877,#28878,
#28879,#28880,#28881,#28882,#28883,#28884,#28885,#28886,#28887,#28888,#28889,
#28890,#28891,#28892,#28893,#28894),.UNSPECIFIED.,.F.,.F.,(4,3,3,3,3,3,
3,3,3,3,3,3,3,3,3,3,3,3,3,3,3,3,3,3,3,3,3,3,3,3,3,3,3,3,3,3,4),(-0.933975894023124,
-0.897518245917797,-0.85418730917007,-0.828760118608177,-0.810932623488333,
-0.801688081435698,-0.75915821677069,-0.716968557512012,-0.68769245742961,
-0.681621420340466,-0.675695062647656,-0.658416357347208,-0.61685703941993,
-0.575176630920201,-0.534137469845906,-0.507834227956848,-0.502068244191955,
-0.496724770966358,-0.456296287597963,-0.428924502289673,-0.388319492614483,
-0.348042200526848,-0.337185447634125,-0.330206209215421,-0.324918360767453,
-0.285434308044378,-0.246386225108482,-0.209399208416579,-0.183224307364507,
-0.169375884861305,-0.161952755019649,-0.156778294147562,-0.117583720610671,
-0.0792968209528158,-0.0396484104764079,-0.00263560956954647,0.),
 .UNSPECIFIED.);
#6003=B_SPLINE_CURVE_WITH_KNOTS('',3,(#29671,#29672,#29673,#29674,#29675,
#29676,#29677,#29678,#29679,#29680,#29681,#29682,#29683,#29684,#29685,#29686,
#29687,#29688,#29689,#29690,#29691,#29692,#29693,#29694,#29695,#29696,#29697,
#29698,#29699,#29700,#29701,#29702,#29703,#29704,#29705,#29706,#29707),
 .UNSPECIFIED.,.F.,.F.,(4,3,3,3,3,3,3,3,3,3,3,3,4),(89.0794763097302,89.1571881949378,
89.6552730451889,90.1533578954399,90.651442745691,91.149527595942,91.6476124461931,
92.1456972964441,92.6437821466952,93.1418669969462,93.6399518471973,94.1380366974483,
94.5619388730527),.UNSPECIFIED.);
#6004=B_SPLINE_CURVE_WITH_KNOTS('',3,(#29709,#29710,#29711,#29712,#29713,
#29714,#29715,#29716,#29717,#29718,#29719,#29720,#29721,#29722,#29723,#29724,
#29725,#29726,#29727,#29728,#29729,#29730,#29731,#29732,#29733,#29734,#29735,
#29736,#29737,#29738,#29739,#29740,#29741,#29742,#29743,#29744,#29745,#29746,
#29747,#29748,#29749,#29750,#29751,#29752,#29753,#29754,#29755,#29756,#29757,
#29758,#29759,#29760,#29761,#29762,#29763,#29764,#29765,#29766,#29767,#29768,
#29769,#29770,#29771,#29772,#29773,#29774,#29775,#29776,#29777,#29778,#29779,
#29780,#29781,#29782,#29783,#29784,#29785,#29786,#29787,#29788,#29789,#29790,
#29791,#29792,#29793,#29794,#29795,#29796,#29797,#29798,#29799,#29800,#29801,
#29802,#29803,#29804,#29805,#29806,#29807,#29808,#29809,#29810,#29811,#29812,
#29813,#29814,#29815,#29816,#29817,#29818,#29819,#29820),.UNSPECIFIED.,
 .F.,.F.,(4,3,3,3,3,3,3,3,3,3,3,3,3,3,3,3,3,3,3,3,3,3,3,3,3,3,3,3,3,3,3,
3,3,3,3,3,3,4),(-0.937740963081777,-0.907140654471705,-0.869270990721146,
-0.847580460872939,-0.836481370719858,-0.829351942923115,-0.823129305042622,
-0.784196547851699,-0.745021725430866,-0.731277450252294,-0.718322019189878,
-0.71228044507783,-0.695746751935491,-0.656667795916307,-0.616960751834722,
-0.581187602694266,-0.554357740838925,-0.548462261493557,-0.542574361216013,
-0.501604132790064,-0.4738681552729,-0.43313752173811,-0.392064143224716,
-0.380617571602666,-0.373704828437967,-0.367641520509243,-0.325920760345294,
-0.283682082032713,-0.241892561201202,-0.211655991051052,-0.19827764062779,
-0.190678095304841,-0.184988742699727,-0.142742050577153,-0.0995959952880378,
-0.0562915047899489,-0.0133559696020479,0.),.UNSPECIFIED.);
#6005=B_SPLINE_CURVE_WITH_KNOTS('',3,(#29821,#29822,#29823,#29824,#29825,
#29826,#29827,#29828,#29829,#29830,#29831,#29832,#29833,#29834),
 .UNSPECIFIED.,.F.,.F.,(4,1,1,1,1,1,1,1,1,1,1,4),(10.3764180272042,10.8003202028086,
11.2984050530596,11.7964899033107,12.2945747535617,12.7926596038128,13.2907444540638,
13.7888293043149,14.2869141545659,14.784999004817,15.283083855068,15.7079632679489),
 .UNSPECIFIED.);
#6006=B_SPLINE_CURVE_WITH_KNOTS('',3,(#29838,#29839,#29840,#29841,#29842,
#29843,#29844,#29845,#29846,#29847,#29848,#29849),.UNSPECIFIED.,.F.,.F.,
(4,1,1,1,1,1,1,1,1,4),(11.6147305479242,12.1128153981753,12.6109002484263,
13.1089850986774,13.6070699489284,14.1051547991795,14.6032396494305,15.1013244996816,
15.5994093499326,15.7079632679489),.UNSPECIFIED.);
#6007=B_SPLINE_CURVE_WITH_KNOTS('',3,(#30626,#30627,#30628,#30629,#30630,
#30631,#30632,#30633,#30634,#30635,#30636,#30637,#30638,#30639,#30640,#30641,
#30642,#30643,#30644,#30645,#30646,#30647,#30648,#30649,#30650,#30651,#30652,
#30653,#30654,#30655,#30656,#30657,#30658,#30659,#30660,#30661,#30662,#30663,
#30664,#30665,#30666,#30667,#30668,#30669,#30670,#30671,#30672,#30673,#30674,
#30675,#30676,#30677,#30678,#30679,#30680,#30681,#30682,#30683,#30684,#30685,
#30686,#30687,#30688,#30689,#30690,#30691,#30692,#30693,#30694,#30695,#30696,
#30697,#30698,#30699,#30700,#30701,#30702,#30703,#30704,#30705,#30706,#30707,
#30708,#30709,#30710,#30711,#30712,#30713,#30714,#30715,#30716,#30717,#30718,
#30719,#30720,#30721,#30722,#30723,#30724,#30725,#30726,#30727,#30728,#30729,
#30730,#30731,#30732,#30733,#30734),.UNSPECIFIED.,.F.,.F.,(4,3,3,3,3,3,
3,3,3,3,3,3,3,3,3,3,3,3,3,3,3,3,3,3,3,3,3,3,3,3,3,3,3,3,3,3,4),(-0.93397589402311,
-0.897518245917774,-0.854187309108942,-0.828760118100427,-0.810932622175928,
-0.80168808147928,-0.759158216888781,-0.71696855880315,-0.68769245807517,
-0.681621420864493,-0.67569506273405,-0.65841635734719,-0.616857039876412,
-0.575176628785756,-0.534137456961281,-0.50783421829338,-0.502068149909085,
-0.496724747629148,-0.456296258740099,-0.428924502289679,-0.388319496329734,
-0.348042218766811,-0.337185483602948,-0.330206404188209,-0.324918477526632,
-0.285434428793379,-0.246386363191161,-0.209399208416591,-0.183224307364517,
-0.169375887565707,-0.161952767222463,-0.156778312515109,-0.117583734386332,
-0.0792968228051709,-0.0396484114025855,-0.00263558281026646,0.),
 .UNSPECIFIED.);
#6008=B_SPLINE_CURVE_WITH_KNOTS('',3,(#30735,#30736,#30737,#30738,#30739,
#30740,#30741,#30742,#30743,#30744,#30745,#30746,#30747,#30748,#30749,#30750,
#30751,#30752,#30753,#30754,#30755,#30756,#30757,#30758,#30759,#30760,#30761,
#30762,#30763,#30764,#30765),.UNSPECIFIED.,.F.,.F.,(4,3,3,3,3,3,3,3,3,3,
4),(-96.6284609487036,-96.1303760984525,-95.6322912482015,-95.1342063979505,
-94.6361215476994,-94.1380366974484,-93.6399518471973,-93.1418669969463,
-92.6437821466952,-92.1456972964442,-92.057827020539),.UNSPECIFIED.);
#6009=B_SPLINE_CURVE_WITH_KNOTS('',3,(#31545,#31546,#31547,#31548,#31549,
#31550,#31551,#31552,#31553,#31554,#31555,#31556,#31557,#31558,#31559,#31560,
#31561,#31562,#31563,#31564,#31565,#31566,#31567,#31568,#31569,#31570,#31571,
#31572,#31573,#31574,#31575,#31576,#31577,#31578,#31579,#31580,#31581,#31582,
#31583,#31584,#31585,#31586,#31587,#31588,#31589,#31590,#31591,#31592,#31593,
#31594,#31595,#31596,#31597,#31598,#31599,#31600,#31601,#31602,#31603,#31604,
#31605,#31606,#31607,#31608,#31609,#31610,#31611,#31612,#31613,#31614,#31615,
#31616,#31617,#31618,#31619,#31620,#31621,#31622,#31623,#31624,#31625,#31626,
#31627,#31628,#31629,#31630,#31631,#31632,#31633,#31634,#31635,#31636,#31637,
#31638,#31639,#31640,#31641,#31642,#31643,#31644,#31645,#31646,#31647,#31648,
#31649,#31650,#31651,#31652,#31653),.UNSPECIFIED.,.F.,.F.,(4,3,3,3,3,3,
3,3,3,3,3,3,3,3,3,3,3,3,3,3,3,3,3,3,3,3,3,3,3,3,3,3,3,3,3,3,4),(-0.933975894023072,
-0.897518245917738,-0.854187309124176,-0.828760118193598,-0.810932622421368,
-0.801688081392097,-0.759158216787806,-0.71696855847361,-0.68769245791039,
-0.681621420681061,-0.675695062695478,-0.65841635734717,-0.616857039787599,
-0.57517662920082,-0.534137459479038,-0.507834220181699,-0.50206816750527,
-0.496724751985825,-0.456296264177866,-0.428924502289679,-0.388319495603713,
-0.348042215202905,-0.337185476574032,-0.330206366049313,-0.324918454649377,
-0.285434405134626,-0.246386336138671,-0.209399208416599,-0.183224307364524,
-0.16937588703651,-0.161952764832493,-0.156778308884714,-0.117583731663536,
-0.07929682241449,-0.039648411207245,-0.00263558803031834,0.),
 .UNSPECIFIED.);
#6010=B_SPLINE_CURVE_WITH_KNOTS('',3,(#31654,#31655,#31656,#31657,#31658,
#31659,#31660,#31661,#31662,#31663,#31664,#31665,#31666,#31667,#31668,#31669,
#31670,#31671,#31672,#31673,#31674,#31675,#31676,#31677,#31678,#31679,#31680,
#31681,#31682,#31683,#31684,#31685,#31686,#31687,#31688,#31689,#31690),
 .UNSPECIFIED.,.F.,.F.,(4,3,3,3,3,3,3,3,3,3,3,3,4),(89.0794763097301,89.1571881949378,
89.6552730451889,90.1533578954399,90.651442745691,91.149527595942,91.6476124461931,
92.1456972964441,92.6437821466952,93.1418669969462,93.6399518471973,94.1380366974483,
94.5619388730527),.UNSPECIFIED.);
#6011=B_SPLINE_CURVE_WITH_KNOTS('',3,(#31692,#31693,#31694,#31695,#31696,
#31697,#31698,#31699,#31700,#31701,#31702,#31703,#31704,#31705,#31706,#31707,
#31708,#31709,#31710,#31711,#31712,#31713,#31714,#31715,#31716,#31717,#31718,
#31719,#31720,#31721,#31722,#31723,#31724,#31725,#31726,#31727,#31728,#31729,
#31730,#31731,#31732,#31733,#31734,#31735,#31736,#31737,#31738,#31739,#31740,
#31741,#31742,#31743,#31744,#31745,#31746,#31747,#31748,#31749,#31750,#31751,
#31752,#31753,#31754,#31755,#31756,#31757,#31758,#31759,#31760,#31761,#31762,
#31763,#31764,#31765,#31766,#31767,#31768,#31769,#31770,#31771,#31772,#31773,
#31774,#31775,#31776,#31777,#31778,#31779,#31780,#31781,#31782,#31783,#31784,
#31785,#31786,#31787,#31788,#31789,#31790,#31791,#31792,#31793,#31794,#31795,
#31796,#31797,#31798,#31799,#31800,#31801,#31802,#31803),.UNSPECIFIED.,
 .F.,.F.,(4,3,3,3,3,3,3,3,3,3,3,3,3,3,3,3,3,3,3,3,3,3,3,3,3,3,3,3,3,3,3,
3,3,3,3,3,3,4),(-0.937740963081779,-0.907140654471699,-0.869270993771617,
-0.847580463542101,-0.836481370403699,-0.829351940484709,-0.823129304651435,
-0.784196549047682,-0.745021726528349,-0.731277450780518,-0.718322019931952,
-0.71228044519251,-0.695746751935487,-0.656667791699655,-0.616960746051451,
-0.581187598356812,-0.554357737585833,-0.548462244751326,-0.542574359801447,
-0.501604130842675,-0.473868155272894,-0.43313751849459,-0.392064138499691,
-0.380617562658136,-0.373704787334874,-0.367641531325938,-0.325920767956713,
-0.283682090161745,-0.241892561201193,-0.211655991051044,-0.198277640840565,
-0.190678095160864,-0.184988742533586,-0.142742064539499,-0.0995960169687047,
-0.0562915264308693,-0.0133559775752571,0.),.UNSPECIFIED.);
#6012=B_SPLINE_CURVE_WITH_KNOTS('',3,(#31804,#31805,#31806,#31807,#31808,
#31809,#31810,#31811,#31812,#31813,#31814,#31815,#31816,#31817),
 .UNSPECIFIED.,.F.,.F.,(4,1,1,1,1,1,1,1,1,1,1,4),(10.3764180272042,10.8003202028086,
11.2984050530597,11.7964899033107,12.2945747535618,12.7926596038128,13.2907444540639,
13.7888293043149,14.286914154566,14.784999004817,15.2830838550681,15.7079632679489),
 .UNSPECIFIED.);
#6013=B_SPLINE_CURVE_WITH_KNOTS('',3,(#31823,#31824,#31825,#31826,#31827,
#31828,#31829,#31830,#31831,#31832,#31833,#31834,#31835,#31836,#31837,#31838,
#31839,#31840,#31841,#31842,#31843,#31844,#31845,#31846,#31847,#31848,#31849,
#31850,#31851,#31852,#31853,#31854,#31855,#31856,#31857,#31858,#31859,#31860,
#31861,#31862,#31863,#31864,#31865,#31866,#31867,#31868,#31869,#31870,#31871,
#31872,#31873,#31874,#31875,#31876,#31877,#31878,#31879,#31880,#31881,#31882,
#31883,#31884,#31885,#31886,#31887,#31888,#31889,#31890,#31891,#31892,#31893,
#31894,#31895,#31896,#31897,#31898,#31899,#31900,#31901,#31902,#31903,#31904,
#31905,#31906,#31907,#31908,#31909,#31910,#31911,#31912,#31913,#31914,#31915,
#31916,#31917,#31918,#31919,#31920,#31921,#31922,#31923,#31924,#31925,#31926,
#31927,#31928,#31929,#31930,#31931),.UNSPECIFIED.,.F.,.F.,(4,3,3,3,3,3,
3,3,3,3,3,3,3,3,3,3,3,3,3,3,3,3,3,3,3,3,3,3,3,3,3,3,3,3,3,3,4),(-0.933975894023121,
-0.897518245917767,-0.854187309175765,-0.828760118641236,-0.810932623574739,
-0.801688081325471,-0.759158216653522,-0.716968557323443,-0.687692457335314,
-0.681621420365228,-0.675695062658239,-0.658416357347185,-0.616857039390373,
-0.575176631065956,-0.534137470686732,-0.507834228587468,-0.502068250144193,
-0.496724772439772,-0.456296289429253,-0.428924502289677,-0.388319492373081,
-0.348042199363598,-0.337185445339697,-0.330206196889632,-0.324918353494149,
-0.285434300515691,-0.246386216454576,-0.209399208416591,-0.183224307364517,
-0.169375884685895,-0.161952754236312,-0.156778292889002,-0.117583719666752,
-0.079296820779602,-0.039648410389801,-0.00263561129235572,0.),
 .UNSPECIFIED.);
#6014=B_SPLINE_CURVE_WITH_KNOTS('',3,(#31934,#31935,#31936,#31937,#31938,
#31939,#31940,#31941,#31942,#31943,#31944,#31945),.UNSPECIFIED.,.F.,.F.,
(4,1,1,1,1,1,1,1,1,4),(11.6147305479242,12.1128153981753,12.6109002484263,
13.1089850986774,13.6070699489284,14.1051547991795,14.6032396494305,15.1013244996816,
15.5994093499326,15.7079632679489),.UNSPECIFIED.);
#6015=B_SPLINE_CURVE_WITH_KNOTS('',3,(#32723,#32724,#32725,#32726,#32727,
#32728,#32729,#32730,#32731,#32732,#32733,#32734,#32735,#32736,#32737,#32738,
#32739,#32740,#32741,#32742,#32743,#32744,#32745,#32746,#32747,#32748,#32749,
#32750,#32751,#32752,#32753,#32754,#32755,#32756,#32757,#32758,#32759,#32760,
#32761,#32762,#32763,#32764,#32765,#32766,#32767,#32768,#32769,#32770,#32771,
#32772,#32773,#32774,#32775,#32776,#32777,#32778,#32779,#32780,#32781,#32782,
#32783,#32784,#32785,#32786,#32787,#32788,#32789,#32790,#32791,#32792,#32793,
#32794,#32795,#32796,#32797,#32798,#32799,#32800,#32801,#32802,#32803,#32804,
#32805,#32806,#32807,#32808,#32809,#32810,#32811,#32812,#32813,#32814,#32815,
#32816,#32817,#32818,#32819,#32820,#32821,#32822,#32823,#32824,#32825,#32826,
#32827,#32828,#32829,#32830,#32831,#32832,#32833,#32834),.UNSPECIFIED.,
 .F.,.F.,(4,3,3,3,3,3,3,3,3,3,3,3,3,3,3,3,3,3,3,3,3,3,3,3,3,3,3,3,3,3,3,
3,3,3,3,3,3,4),(-0.93774096308169,-0.907140654471617,-0.869270990472425,
-0.847580460655302,-0.836481370750679,-0.829351942943646,-0.823129305038796,
-0.784196547713336,-0.7450217252948,-0.731277450146466,-0.71832201906501,
-0.712280445054707,-0.695746751935441,-0.656667796256735,-0.616960752300126,
-0.581187603043312,-0.554357741100701,-0.548462262818575,-0.542574361327803,
-0.501604132950922,-0.473868155272869,-0.433137521996099,-0.392064143603576,
-0.380617572320162,-0.373704831737396,-0.367641519570074,-0.325920759661173,
-0.283682081306335,-0.241892561201191,-0.211655991051042,-0.19827764061072,
-0.190678095317729,-0.184988742720608,-0.142742049467821,-0.099595993558808,
-0.0562915030637826,-0.0133559689776526,0.),.UNSPECIFIED.);
#6016=B_SPLINE_CURVE_WITH_KNOTS('',3,(#32835,#32836,#32837,#32838,#32839,
#32840,#32841,#32842,#32843,#32844,#32845,#32846,#32847,#32848,#32849,#32850,
#32851,#32852,#32853,#32854,#32855,#32856,#32857,#32858,#32859,#32860,#32861,
#32862,#32863,#32864,#32865),.UNSPECIFIED.,.F.,.F.,(4,3,3,3,3,3,3,3,3,3,
4),(-96.6284609487036,-96.1303760984525,-95.6322912482015,-95.1342063979505,
-94.6361215476994,-94.1380366974483,-93.6399518471973,-93.1418669969462,
-92.6437821466952,-92.1456972964441,-92.0578270205389),.UNSPECIFIED.);
#7057=VERTEX_POINT('',#25123);
#7058=VERTEX_POINT('',#25124);
#7059=VERTEX_POINT('',#25126);
#7060=VERTEX_POINT('',#25143);
#7061=VERTEX_POINT('',#25156);
#7062=VERTEX_POINT('',#25157);
#7063=VERTEX_POINT('',#25240);
#7064=VERTEX_POINT('',#25241);
#7065=VERTEX_POINT('',#25330);
#7066=VERTEX_POINT('',#25331);
#7067=VERTEX_POINT('',#25420);
#7068=VERTEX_POINT('',#25421);
#7069=VERTEX_POINT('',#25504);
#7070=VERTEX_POINT('',#25505);
#7071=VERTEX_POINT('',#25594);
#7072=VERTEX_POINT('',#25595);
#7073=VERTEX_POINT('',#25678);
#7074=VERTEX_POINT('',#25679);
#7075=VERTEX_POINT('',#25765);
#7076=VERTEX_POINT('',#25766);
#7077=VERTEX_POINT('',#25840);
#7078=VERTEX_POINT('',#25841);
#7079=VERTEX_POINT('',#25924);
#7080=VERTEX_POINT('',#25925);
#7081=VERTEX_POINT('',#26014);
#7082=VERTEX_POINT('',#26015);
#7083=VERTEX_POINT('',#26098);
#7084=VERTEX_POINT('',#26099);
#7085=VERTEX_POINT('',#26185);
#7086=VERTEX_POINT('',#26186);
#7087=VERTEX_POINT('',#26275);
#7088=VERTEX_POINT('',#26276);
#7089=VERTEX_POINT('',#26359);
#7090=VERTEX_POINT('',#26360);
#7091=VERTEX_POINT('',#26362);
#7092=VERTEX_POINT('',#26372);
#7093=VERTEX_POINT('',#26381);
#7094=VERTEX_POINT('',#26382);
#7095=VERTEX_POINT('',#26418);
#7096=VERTEX_POINT('',#26419);
#7097=VERTEX_POINT('',#26455);
#7098=VERTEX_POINT('',#26456);
#7099=VERTEX_POINT('',#26493);
#7100=VERTEX_POINT('',#26494);
#7101=VERTEX_POINT('',#26530);
#7102=VERTEX_POINT('',#26531);
#7103=VERTEX_POINT('',#26567);
#7104=VERTEX_POINT('',#26568);
#7105=VERTEX_POINT('',#26604);
#7106=VERTEX_POINT('',#26605);
#7107=VERTEX_POINT('',#26639);
#7108=VERTEX_POINT('',#26640);
#7109=VERTEX_POINT('',#26673);
#7110=VERTEX_POINT('',#26674);
#7111=VERTEX_POINT('',#26710);
#7112=VERTEX_POINT('',#26711);
#7113=VERTEX_POINT('',#26747);
#7114=VERTEX_POINT('',#26748);
#7115=VERTEX_POINT('',#26784);
#7116=VERTEX_POINT('',#26785);
#7117=VERTEX_POINT('',#26821);
#7118=VERTEX_POINT('',#26822);
#7119=VERTEX_POINT('',#26859);
#7120=VERTEX_POINT('',#26860);
#7121=VERTEX_POINT('',#26896);
#7122=VERTEX_POINT('',#26897);
#7123=VERTEX_POINT('',#26899);
#7124=VERTEX_POINT('',#26916);
#7125=VERTEX_POINT('',#26929);
#7126=VERTEX_POINT('',#26930);
#7127=VERTEX_POINT('',#27013);
#7128=VERTEX_POINT('',#27014);
#7129=VERTEX_POINT('',#27103);
#7130=VERTEX_POINT('',#27104);
#7131=VERTEX_POINT('',#27193);
#7132=VERTEX_POINT('',#27194);
#7133=VERTEX_POINT('',#27277);
#7134=VERTEX_POINT('',#27278);
#7135=VERTEX_POINT('',#27367);
#7136=VERTEX_POINT('',#27368);
#7137=VERTEX_POINT('',#27451);
#7138=VERTEX_POINT('',#27452);
#7139=VERTEX_POINT('',#27538);
#7140=VERTEX_POINT('',#27539);
#7141=VERTEX_POINT('',#27613);
#7142=VERTEX_POINT('',#27614);
#7143=VERTEX_POINT('',#27697);
#7144=VERTEX_POINT('',#27698);
#7145=VERTEX_POINT('',#27787);
#7146=VERTEX_POINT('',#27788);
#7147=VERTEX_POINT('',#27871);
#7148=VERTEX_POINT('',#27872);
#7149=VERTEX_POINT('',#27958);
#7150=VERTEX_POINT('',#27959);
#7151=VERTEX_POINT('',#28048);
#7152=VERTEX_POINT('',#28049);
#7153=VERTEX_POINT('',#28132);
#7154=VERTEX_POINT('',#28133);
#7155=VERTEX_POINT('',#28135);
#7156=VERTEX_POINT('',#28145);
#7157=VERTEX_POINT('',#28154);
#7158=VERTEX_POINT('',#28155);
#7159=VERTEX_POINT('',#28191);
#7160=VERTEX_POINT('',#28192);
#7161=VERTEX_POINT('',#28228);
#7162=VERTEX_POINT('',#28229);
#7163=VERTEX_POINT('',#28266);
#7164=VERTEX_POINT('',#28267);
#7165=VERTEX_POINT('',#28303);
#7166=VERTEX_POINT('',#28304);
#7167=VERTEX_POINT('',#28340);
#7168=VERTEX_POINT('',#28341);
#7169=VERTEX_POINT('',#28377);
#7170=VERTEX_POINT('',#28378);
#7171=VERTEX_POINT('',#28412);
#7172=VERTEX_POINT('',#28413);
#7173=VERTEX_POINT('',#28446);
#7174=VERTEX_POINT('',#28447);
#7175=VERTEX_POINT('',#28483);
#7176=VERTEX_POINT('',#28484);
#7177=VERTEX_POINT('',#28520);
#7178=VERTEX_POINT('',#28521);
#7179=VERTEX_POINT('',#28557);
#7180=VERTEX_POINT('',#28558);
#7181=VERTEX_POINT('',#28594);
#7182=VERTEX_POINT('',#28595);
#7183=VERTEX_POINT('',#28632);
#7184=VERTEX_POINT('',#28633);
#7185=VERTEX_POINT('',#28669);
#7186=VERTEX_POINT('',#28782);
#7187=VERTEX_POINT('',#28784);
#7188=VERTEX_POINT('',#29708);
#7189=VERTEX_POINT('',#29836);
#7190=VERTEX_POINT('',#31544);
#7191=VERTEX_POINT('',#31691);
#7192=VERTEX_POINT('',#31819);
#7193=VERTEX_POINT('',#31822);
#7194=VERTEX_POINT('',#32722);
#7195=VERTEX_POINT('',#32867);
#7196=VERTEX_POINT('',#32874);
#7197=VERTEX_POINT('',#32877);
#7198=VERTEX_POINT('',#32882);
#8831=EDGE_CURVE('',#7057,#7058,#4103,.T.);
#8832=EDGE_CURVE('',#7057,#7059,#5881,.T.);
#8833=EDGE_CURVE('',#7059,#7060,#926,.T.);
#8834=EDGE_CURVE('',#7060,#7058,#5882,.T.);
#8835=EDGE_CURVE('',#7061,#7062,#4104,.T.);
#8836=EDGE_CURVE('',#7061,#7057,#5883,.T.);
#8837=EDGE_CURVE('',#7058,#7062,#5884,.T.);
#8838=EDGE_CURVE('',#7063,#7064,#4105,.T.);
#8839=EDGE_CURVE('',#7063,#7061,#5885,.T.);
#8840=EDGE_CURVE('',#7062,#7064,#5886,.T.);
#8841=EDGE_CURVE('',#7065,#7066,#4106,.T.);
#8842=EDGE_CURVE('',#7065,#7063,#5887,.T.);
#8843=EDGE_CURVE('',#7064,#7066,#5888,.T.);
#8844=EDGE_CURVE('',#7067,#7068,#4107,.T.);
#8845=EDGE_CURVE('',#7067,#7065,#5889,.T.);
#8846=EDGE_CURVE('',#7066,#7068,#5890,.T.);
#8847=EDGE_CURVE('',#7069,#7070,#4108,.T.);
#8848=EDGE_CURVE('',#7069,#7067,#5891,.T.);
#8849=EDGE_CURVE('',#7068,#7070,#5892,.T.);
#8850=EDGE_CURVE('',#7071,#7072,#4109,.T.);
#8851=EDGE_CURVE('',#7071,#7069,#5893,.T.);
#8852=EDGE_CURVE('',#7070,#7072,#5894,.T.);
#8853=EDGE_CURVE('',#7073,#7074,#4110,.T.);
#8854=EDGE_CURVE('',#7073,#7071,#5895,.T.);
#8855=EDGE_CURVE('',#7072,#7074,#5896,.T.);
#8856=EDGE_CURVE('',#7075,#7076,#4111,.T.);
#8857=EDGE_CURVE('',#7075,#7073,#5897,.T.);
#8858=EDGE_CURVE('',#7074,#7076,#5898,.T.);
#8859=EDGE_CURVE('',#7077,#7078,#4112,.T.);
#8860=EDGE_CURVE('',#7077,#7075,#5899,.T.);
#8861=EDGE_CURVE('',#7076,#7078,#5900,.T.);
#8862=EDGE_CURVE('',#7079,#7080,#4113,.T.);
#8863=EDGE_CURVE('',#7079,#7077,#5901,.T.);
#8864=EDGE_CURVE('',#7078,#7080,#5902,.T.);
#8865=EDGE_CURVE('',#7081,#7082,#4114,.T.);
#8866=EDGE_CURVE('',#7081,#7079,#5903,.T.);
#8867=EDGE_CURVE('',#7080,#7082,#5904,.T.);
#8868=EDGE_CURVE('',#7083,#7084,#4115,.T.);
#8869=EDGE_CURVE('',#7083,#7081,#5905,.T.);
#8870=EDGE_CURVE('',#7082,#7084,#5906,.T.);
#8871=EDGE_CURVE('',#7085,#7086,#4116,.T.);
#8872=EDGE_CURVE('',#7085,#7083,#5907,.T.);
#8873=EDGE_CURVE('',#7084,#7086,#5908,.T.);
#8874=EDGE_CURVE('',#7087,#7088,#4117,.T.);
#8875=EDGE_CURVE('',#7087,#7085,#5909,.T.);
#8876=EDGE_CURVE('',#7086,#7088,#5910,.T.);
#8877=EDGE_CURVE('',#7089,#7090,#4118,.T.);
#8878=EDGE_CURVE('',#7089,#7091,#5911,.T.);
#8879=EDGE_CURVE('',#7092,#7091,#927,.T.);
#8880=EDGE_CURVE('',#7090,#7092,#5912,.T.);
#8881=EDGE_CURVE('',#7093,#7094,#4119,.T.);
#8882=EDGE_CURVE('',#7093,#7089,#5913,.T.);
#8883=EDGE_CURVE('',#7094,#7090,#5914,.T.);
#8884=EDGE_CURVE('',#7095,#7096,#4120,.T.);
#8885=EDGE_CURVE('',#7095,#7093,#5915,.T.);
#8886=EDGE_CURVE('',#7096,#7094,#5916,.T.);
#8887=EDGE_CURVE('',#7097,#7098,#4121,.T.);
#8888=EDGE_CURVE('',#7097,#7095,#5917,.T.);
#8889=EDGE_CURVE('',#7098,#7096,#5918,.T.);
#8890=EDGE_CURVE('',#7099,#7100,#4122,.T.);
#8891=EDGE_CURVE('',#7099,#7097,#5919,.T.);
#8892=EDGE_CURVE('',#7100,#7098,#5920,.T.);
#8893=EDGE_CURVE('',#7101,#7102,#4123,.T.);
#8894=EDGE_CURVE('',#7101,#7099,#5921,.T.);
#8895=EDGE_CURVE('',#7102,#7100,#5922,.T.);
#8896=EDGE_CURVE('',#7103,#7104,#4124,.T.);
#8897=EDGE_CURVE('',#7103,#7101,#5923,.T.);
#8898=EDGE_CURVE('',#7104,#7102,#5924,.T.);
#8899=EDGE_CURVE('',#7105,#7106,#4125,.T.);
#8900=EDGE_CURVE('',#7105,#7103,#5925,.T.);
#8901=EDGE_CURVE('',#7106,#7104,#5926,.T.);
#8902=EDGE_CURVE('',#7107,#7108,#4126,.T.);
#8903=EDGE_CURVE('',#7107,#7105,#5927,.T.);
#8904=EDGE_CURVE('',#7108,#7106,#5928,.T.);
#8905=EDGE_CURVE('',#7109,#7110,#4127,.T.);
#8906=EDGE_CURVE('',#7109,#7107,#5929,.T.);
#8907=EDGE_CURVE('',#7110,#7108,#5930,.T.);
#8908=EDGE_CURVE('',#7111,#7112,#4128,.T.);
#8909=EDGE_CURVE('',#7111,#7109,#5931,.T.);
#8910=EDGE_CURVE('',#7112,#7110,#5932,.T.);
#8911=EDGE_CURVE('',#7113,#7114,#4129,.T.);
#8912=EDGE_CURVE('',#7113,#7111,#5933,.T.);
#8913=EDGE_CURVE('',#7114,#7112,#5934,.T.);
#8914=EDGE_CURVE('',#7115,#7116,#4130,.T.);
#8915=EDGE_CURVE('',#7115,#7113,#5935,.T.);
#8916=EDGE_CURVE('',#7116,#7114,#5936,.T.);
#8917=EDGE_CURVE('',#7117,#7118,#4131,.T.);
#8918=EDGE_CURVE('',#7117,#7115,#5937,.T.);
#8919=EDGE_CURVE('',#7118,#7116,#5938,.T.);
#8920=EDGE_CURVE('',#7119,#7120,#4132,.T.);
#8921=EDGE_CURVE('',#7119,#7117,#5939,.T.);
#8922=EDGE_CURVE('',#7120,#7118,#5940,.T.);
#8923=EDGE_CURVE('',#7121,#7122,#4133,.T.);
#8924=EDGE_CURVE('',#7121,#7123,#5941,.T.);
#8925=EDGE_CURVE('',#7123,#7124,#928,.F.);
#8926=EDGE_CURVE('',#7124,#7122,#5942,.T.);
#8927=EDGE_CURVE('',#7125,#7126,#4134,.T.);
#8928=EDGE_CURVE('',#7125,#7121,#5943,.T.);
#8929=EDGE_CURVE('',#7122,#7126,#5944,.T.);
#8930=EDGE_CURVE('',#7127,#7128,#4135,.T.);
#8931=EDGE_CURVE('',#7127,#7125,#5945,.T.);
#8932=EDGE_CURVE('',#7126,#7128,#5946,.T.);
#8933=EDGE_CURVE('',#7129,#7130,#4136,.T.);
#8934=EDGE_CURVE('',#7129,#7127,#5947,.T.);
#8935=EDGE_CURVE('',#7128,#7130,#5948,.T.);
#8936=EDGE_CURVE('',#7131,#7132,#4137,.T.);
#8937=EDGE_CURVE('',#7131,#7129,#5949,.T.);
#8938=EDGE_CURVE('',#7130,#7132,#5950,.T.);
#8939=EDGE_CURVE('',#7133,#7134,#4138,.T.);
#8940=EDGE_CURVE('',#7133,#7131,#5951,.T.);
#8941=EDGE_CURVE('',#7132,#7134,#5952,.T.);
#8942=EDGE_CURVE('',#7135,#7136,#4139,.T.);
#8943=EDGE_CURVE('',#7135,#7133,#5953,.T.);
#8944=EDGE_CURVE('',#7134,#7136,#5954,.T.);
#8945=EDGE_CURVE('',#7137,#7138,#4140,.T.);
#8946=EDGE_CURVE('',#7137,#7135,#5955,.T.);
#8947=EDGE_CURVE('',#7136,#7138,#5956,.T.);
#8948=EDGE_CURVE('',#7139,#7140,#4141,.T.);
#8949=EDGE_CURVE('',#7139,#7137,#5957,.T.);
#8950=EDGE_CURVE('',#7138,#7140,#5958,.T.);
#8951=EDGE_CURVE('',#7141,#7142,#4142,.T.);
#8952=EDGE_CURVE('',#7141,#7139,#5959,.T.);
#8953=EDGE_CURVE('',#7140,#7142,#5960,.T.);
#8954=EDGE_CURVE('',#7143,#7144,#4143,.T.);
#8955=EDGE_CURVE('',#7143,#7141,#5961,.T.);
#8956=EDGE_CURVE('',#7142,#7144,#5962,.T.);
#8957=EDGE_CURVE('',#7145,#7146,#4144,.T.);
#8958=EDGE_CURVE('',#7145,#7143,#5963,.T.);
#8959=EDGE_CURVE('',#7144,#7146,#5964,.T.);
#8960=EDGE_CURVE('',#7147,#7148,#4145,.T.);
#8961=EDGE_CURVE('',#7147,#7145,#5965,.T.);
#8962=EDGE_CURVE('',#7146,#7148,#5966,.T.);
#8963=EDGE_CURVE('',#7149,#7150,#4146,.T.);
#8964=EDGE_CURVE('',#7149,#7147,#5967,.T.);
#8965=EDGE_CURVE('',#7148,#7150,#5968,.T.);
#8966=EDGE_CURVE('',#7151,#7152,#4147,.T.);
#8967=EDGE_CURVE('',#7151,#7149,#5969,.T.);
#8968=EDGE_CURVE('',#7150,#7152,#5970,.T.);
#8969=EDGE_CURVE('',#7153,#7154,#4148,.T.);
#8970=EDGE_CURVE('',#7153,#7155,#5971,.T.);
#8971=EDGE_CURVE('',#7156,#7155,#929,.T.);
#8972=EDGE_CURVE('',#7154,#7156,#5972,.T.);
#8973=EDGE_CURVE('',#7157,#7158,#4149,.T.);
#8974=EDGE_CURVE('',#7157,#7153,#5973,.T.);
#8975=EDGE_CURVE('',#7158,#7154,#5974,.T.);
#8976=EDGE_CURVE('',#7159,#7160,#4150,.T.);
#8977=EDGE_CURVE('',#7159,#7157,#5975,.T.);
#8978=EDGE_CURVE('',#7160,#7158,#5976,.T.);
#8979=EDGE_CURVE('',#7161,#7162,#4151,.T.);
#8980=EDGE_CURVE('',#7161,#7159,#5977,.T.);
#8981=EDGE_CURVE('',#7162,#7160,#5978,.T.);
#8982=EDGE_CURVE('',#7163,#7164,#4152,.T.);
#8983=EDGE_CURVE('',#7163,#7161,#5979,.T.);
#8984=EDGE_CURVE('',#7164,#7162,#5980,.T.);
#8985=EDGE_CURVE('',#7165,#7166,#4153,.T.);
#8986=EDGE_CURVE('',#7165,#7163,#5981,.T.);
#8987=EDGE_CURVE('',#7166,#7164,#5982,.T.);
#8988=EDGE_CURVE('',#7167,#7168,#4154,.T.);
#8989=EDGE_CURVE('',#7167,#7165,#5983,.T.);
#8990=EDGE_CURVE('',#7168,#7166,#5984,.T.);
#8991=EDGE_CURVE('',#7169,#7170,#4155,.T.);
#8992=EDGE_CURVE('',#7169,#7167,#5985,.T.);
#8993=EDGE_CURVE('',#7170,#7168,#5986,.T.);
#8994=EDGE_CURVE('',#7171,#7172,#4156,.T.);
#8995=EDGE_CURVE('',#7171,#7169,#5987,.T.);
#8996=EDGE_CURVE('',#7172,#7170,#5988,.T.);
#8997=EDGE_CURVE('',#7173,#7174,#4157,.T.);
#8998=EDGE_CURVE('',#7173,#7171,#5989,.T.);
#8999=EDGE_CURVE('',#7174,#7172,#5990,.T.);
#9000=EDGE_CURVE('',#7175,#7176,#4158,.T.);
#9001=EDGE_CURVE('',#7175,#7173,#5991,.T.);
#9002=EDGE_CURVE('',#7176,#7174,#5992,.T.);
#9003=EDGE_CURVE('',#7177,#7178,#4159,.T.);
#9004=EDGE_CURVE('',#7177,#7175,#5993,.T.);
#9005=EDGE_CURVE('',#7178,#7176,#5994,.T.);
#9006=EDGE_CURVE('',#7179,#7180,#4160,.T.);
#9007=EDGE_CURVE('',#7179,#7177,#5995,.T.);
#9008=EDGE_CURVE('',#7180,#7178,#5996,.T.);
#9009=EDGE_CURVE('',#7181,#7182,#4161,.T.);
#9010=EDGE_CURVE('',#7181,#7179,#5997,.T.);
#9011=EDGE_CURVE('',#7182,#7180,#5998,.T.);
#9012=EDGE_CURVE('',#7183,#7184,#4162,.T.);
#9013=EDGE_CURVE('',#7183,#7181,#5999,.T.);
#9014=EDGE_CURVE('',#7184,#7182,#6000,.T.);
#9015=EDGE_CURVE('',#7155,#7185,#6001,.T.);
#9016=EDGE_CURVE('',#7186,#7185,#930,.F.);
#9017=EDGE_CURVE('',#7187,#7186,#931,.F.);
#9018=EDGE_CURVE('',#7187,#7156,#6002,.T.);
#9019=EDGE_CURVE('',#7152,#7187,#6003,.T.);
#9020=EDGE_CURVE('',#7188,#7124,#6004,.T.);
#9021=EDGE_CURVE('',#7188,#7184,#6005,.T.);
#9022=EDGE_CURVE('',#7189,#7188,#932,.T.);
#9023=EDGE_CURVE('',#7189,#7183,#6006,.T.);
#9024=EDGE_CURVE('',#7123,#7189,#6007,.T.);
#9025=EDGE_CURVE('',#7185,#7151,#6008,.T.);
#9026=EDGE_CURVE('',#7185,#7187,#933,.F.);
#9027=EDGE_CURVE('',#7190,#7092,#6009,.T.);
#9028=EDGE_CURVE('',#7088,#7190,#6010,.T.);
#9029=EDGE_CURVE('',#7191,#7060,#6011,.T.);
#9030=EDGE_CURVE('',#7191,#7120,#6012,.T.);
#9031=EDGE_CURVE('',#7060,#7192,#934,.T.);
#9032=EDGE_CURVE('',#7192,#7059,#935,.T.);
#9033=EDGE_CURVE('',#7059,#7193,#6013,.T.);
#9034=EDGE_CURVE('',#7193,#7191,#936,.T.);
#9035=EDGE_CURVE('',#7193,#7119,#6014,.T.);
#9036=EDGE_CURVE('',#7091,#7194,#6015,.T.);
#9037=EDGE_CURVE('',#7194,#7087,#6016,.T.);
#9038=EDGE_CURVE('',#7195,#7195,#937,.T.);
#9039=EDGE_CURVE('',#7192,#7195,#4163,.T.);
#9040=EDGE_CURVE('',#7194,#7190,#938,.T.);
#9041=EDGE_CURVE('',#7196,#7196,#939,.T.);
#9042=EDGE_CURVE('',#7197,#7197,#940,.T.);
#9043=EDGE_CURVE('',#7197,#7196,#4164,.T.);
#9044=EDGE_CURVE('',#7198,#7198,#941,.T.);
#9045=EDGE_CURVE('',#7198,#7186,#4165,.T.);
#11848=ORIENTED_EDGE('',*,*,#8831,.F.);
#11849=ORIENTED_EDGE('',*,*,#8832,.T.);
#11850=ORIENTED_EDGE('',*,*,#8833,.T.);
#11851=ORIENTED_EDGE('',*,*,#8834,.T.);
#11852=ORIENTED_EDGE('',*,*,#8835,.F.);
#11853=ORIENTED_EDGE('',*,*,#8836,.T.);
#11854=ORIENTED_EDGE('',*,*,#8831,.T.);
#11855=ORIENTED_EDGE('',*,*,#8837,.T.);
#11856=ORIENTED_EDGE('',*,*,#8838,.F.);
#11857=ORIENTED_EDGE('',*,*,#8839,.T.);
#11858=ORIENTED_EDGE('',*,*,#8835,.T.);
#11859=ORIENTED_EDGE('',*,*,#8840,.T.);
#11860=ORIENTED_EDGE('',*,*,#8841,.F.);
#11861=ORIENTED_EDGE('',*,*,#8842,.T.);
#11862=ORIENTED_EDGE('',*,*,#8838,.T.);
#11863=ORIENTED_EDGE('',*,*,#8843,.T.);
#11864=ORIENTED_EDGE('',*,*,#8844,.F.);
#11865=ORIENTED_EDGE('',*,*,#8845,.T.);
#11866=ORIENTED_EDGE('',*,*,#8841,.T.);
#11867=ORIENTED_EDGE('',*,*,#8846,.T.);
#11868=ORIENTED_EDGE('',*,*,#8847,.F.);
#11869=ORIENTED_EDGE('',*,*,#8848,.T.);
#11870=ORIENTED_EDGE('',*,*,#8844,.T.);
#11871=ORIENTED_EDGE('',*,*,#8849,.T.);
#11872=ORIENTED_EDGE('',*,*,#8850,.F.);
#11873=ORIENTED_EDGE('',*,*,#8851,.T.);
#11874=ORIENTED_EDGE('',*,*,#8847,.T.);
#11875=ORIENTED_EDGE('',*,*,#8852,.T.);
#11876=ORIENTED_EDGE('',*,*,#8853,.F.);
#11877=ORIENTED_EDGE('',*,*,#8854,.T.);
#11878=ORIENTED_EDGE('',*,*,#8850,.T.);
#11879=ORIENTED_EDGE('',*,*,#8855,.T.);
#11880=ORIENTED_EDGE('',*,*,#8856,.F.);
#11881=ORIENTED_EDGE('',*,*,#8857,.T.);
#11882=ORIENTED_EDGE('',*,*,#8853,.T.);
#11883=ORIENTED_EDGE('',*,*,#8858,.T.);
#11884=ORIENTED_EDGE('',*,*,#8859,.F.);
#11885=ORIENTED_EDGE('',*,*,#8860,.T.);
#11886=ORIENTED_EDGE('',*,*,#8856,.T.);
#11887=ORIENTED_EDGE('',*,*,#8861,.T.);
#11888=ORIENTED_EDGE('',*,*,#8862,.F.);
#11889=ORIENTED_EDGE('',*,*,#8863,.T.);
#11890=ORIENTED_EDGE('',*,*,#8859,.T.);
#11891=ORIENTED_EDGE('',*,*,#8864,.T.);
#11892=ORIENTED_EDGE('',*,*,#8865,.F.);
#11893=ORIENTED_EDGE('',*,*,#8866,.T.);
#11894=ORIENTED_EDGE('',*,*,#8862,.T.);
#11895=ORIENTED_EDGE('',*,*,#8867,.T.);
#11896=ORIENTED_EDGE('',*,*,#8868,.F.);
#11897=ORIENTED_EDGE('',*,*,#8869,.T.);
#11898=ORIENTED_EDGE('',*,*,#8865,.T.);
#11899=ORIENTED_EDGE('',*,*,#8870,.T.);
#11900=ORIENTED_EDGE('',*,*,#8871,.F.);
#11901=ORIENTED_EDGE('',*,*,#8872,.T.);
#11902=ORIENTED_EDGE('',*,*,#8868,.T.);
#11903=ORIENTED_EDGE('',*,*,#8873,.T.);
#11904=ORIENTED_EDGE('',*,*,#8874,.F.);
#11905=ORIENTED_EDGE('',*,*,#8875,.T.);
#11906=ORIENTED_EDGE('',*,*,#8871,.T.);
#11907=ORIENTED_EDGE('',*,*,#8876,.T.);
#11908=ORIENTED_EDGE('',*,*,#8877,.F.);
#11909=ORIENTED_EDGE('',*,*,#8878,.T.);
#11910=ORIENTED_EDGE('',*,*,#8879,.F.);
#11911=ORIENTED_EDGE('',*,*,#8880,.F.);
#11912=ORIENTED_EDGE('',*,*,#8881,.F.);
#11913=ORIENTED_EDGE('',*,*,#8882,.T.);
#11914=ORIENTED_EDGE('',*,*,#8877,.T.);
#11915=ORIENTED_EDGE('',*,*,#8883,.F.);
#11916=ORIENTED_EDGE('',*,*,#8884,.F.);
#11917=ORIENTED_EDGE('',*,*,#8885,.T.);
#11918=ORIENTED_EDGE('',*,*,#8881,.T.);
#11919=ORIENTED_EDGE('',*,*,#8886,.F.);
#11920=ORIENTED_EDGE('',*,*,#8887,.F.);
#11921=ORIENTED_EDGE('',*,*,#8888,.T.);
#11922=ORIENTED_EDGE('',*,*,#8884,.T.);
#11923=ORIENTED_EDGE('',*,*,#8889,.F.);
#11924=ORIENTED_EDGE('',*,*,#8890,.F.);
#11925=ORIENTED_EDGE('',*,*,#8891,.T.);
#11926=ORIENTED_EDGE('',*,*,#8887,.T.);
#11927=ORIENTED_EDGE('',*,*,#8892,.F.);
#11928=ORIENTED_EDGE('',*,*,#8893,.F.);
#11929=ORIENTED_EDGE('',*,*,#8894,.T.);
#11930=ORIENTED_EDGE('',*,*,#8890,.T.);
#11931=ORIENTED_EDGE('',*,*,#8895,.F.);
#11932=ORIENTED_EDGE('',*,*,#8896,.F.);
#11933=ORIENTED_EDGE('',*,*,#8897,.T.);
#11934=ORIENTED_EDGE('',*,*,#8893,.T.);
#11935=ORIENTED_EDGE('',*,*,#8898,.F.);
#11936=ORIENTED_EDGE('',*,*,#8899,.F.);
#11937=ORIENTED_EDGE('',*,*,#8900,.T.);
#11938=ORIENTED_EDGE('',*,*,#8896,.T.);
#11939=ORIENTED_EDGE('',*,*,#8901,.F.);
#11940=ORIENTED_EDGE('',*,*,#8902,.F.);
#11941=ORIENTED_EDGE('',*,*,#8903,.T.);
#11942=ORIENTED_EDGE('',*,*,#8899,.T.);
#11943=ORIENTED_EDGE('',*,*,#8904,.F.);
#11944=ORIENTED_EDGE('',*,*,#8905,.F.);
#11945=ORIENTED_EDGE('',*,*,#8906,.T.);
#11946=ORIENTED_EDGE('',*,*,#8902,.T.);
#11947=ORIENTED_EDGE('',*,*,#8907,.F.);
#11948=ORIENTED_EDGE('',*,*,#8908,.F.);
#11949=ORIENTED_EDGE('',*,*,#8909,.T.);
#11950=ORIENTED_EDGE('',*,*,#8905,.T.);
#11951=ORIENTED_EDGE('',*,*,#8910,.F.);
#11952=ORIENTED_EDGE('',*,*,#8911,.F.);
#11953=ORIENTED_EDGE('',*,*,#8912,.T.);
#11954=ORIENTED_EDGE('',*,*,#8908,.T.);
#11955=ORIENTED_EDGE('',*,*,#8913,.F.);
#11956=ORIENTED_EDGE('',*,*,#8914,.F.);
#11957=ORIENTED_EDGE('',*,*,#8915,.T.);
#11958=ORIENTED_EDGE('',*,*,#8911,.T.);
#11959=ORIENTED_EDGE('',*,*,#8916,.F.);
#11960=ORIENTED_EDGE('',*,*,#8917,.F.);
#11961=ORIENTED_EDGE('',*,*,#8918,.T.);
#11962=ORIENTED_EDGE('',*,*,#8914,.T.);
#11963=ORIENTED_EDGE('',*,*,#8919,.F.);
#11964=ORIENTED_EDGE('',*,*,#8920,.F.);
#11965=ORIENTED_EDGE('',*,*,#8921,.T.);
#11966=ORIENTED_EDGE('',*,*,#8917,.T.);
#11967=ORIENTED_EDGE('',*,*,#8922,.F.);
#11968=ORIENTED_EDGE('',*,*,#8923,.F.);
#11969=ORIENTED_EDGE('',*,*,#8924,.T.);
#11970=ORIENTED_EDGE('',*,*,#8925,.T.);
#11971=ORIENTED_EDGE('',*,*,#8926,.T.);
#11972=ORIENTED_EDGE('',*,*,#8927,.F.);
#11973=ORIENTED_EDGE('',*,*,#8928,.T.);
#11974=ORIENTED_EDGE('',*,*,#8923,.T.);
#11975=ORIENTED_EDGE('',*,*,#8929,.T.);
#11976=ORIENTED_EDGE('',*,*,#8930,.F.);
#11977=ORIENTED_EDGE('',*,*,#8931,.T.);
#11978=ORIENTED_EDGE('',*,*,#8927,.T.);
#11979=ORIENTED_EDGE('',*,*,#8932,.T.);
#11980=ORIENTED_EDGE('',*,*,#8933,.F.);
#11981=ORIENTED_EDGE('',*,*,#8934,.T.);
#11982=ORIENTED_EDGE('',*,*,#8930,.T.);
#11983=ORIENTED_EDGE('',*,*,#8935,.T.);
#11984=ORIENTED_EDGE('',*,*,#8936,.F.);
#11985=ORIENTED_EDGE('',*,*,#8937,.T.);
#11986=ORIENTED_EDGE('',*,*,#8933,.T.);
#11987=ORIENTED_EDGE('',*,*,#8938,.T.);
#11988=ORIENTED_EDGE('',*,*,#8939,.F.);
#11989=ORIENTED_EDGE('',*,*,#8940,.T.);
#11990=ORIENTED_EDGE('',*,*,#8936,.T.);
#11991=ORIENTED_EDGE('',*,*,#8941,.T.);
#11992=ORIENTED_EDGE('',*,*,#8942,.F.);
#11993=ORIENTED_EDGE('',*,*,#8943,.T.);
#11994=ORIENTED_EDGE('',*,*,#8939,.T.);
#11995=ORIENTED_EDGE('',*,*,#8944,.T.);
#11996=ORIENTED_EDGE('',*,*,#8945,.F.);
#11997=ORIENTED_EDGE('',*,*,#8946,.T.);
#11998=ORIENTED_EDGE('',*,*,#8942,.T.);
#11999=ORIENTED_EDGE('',*,*,#8947,.T.);
#12000=ORIENTED_EDGE('',*,*,#8948,.F.);
#12001=ORIENTED_EDGE('',*,*,#8949,.T.);
#12002=ORIENTED_EDGE('',*,*,#8945,.T.);
#12003=ORIENTED_EDGE('',*,*,#8950,.T.);
#12004=ORIENTED_EDGE('',*,*,#8951,.F.);
#12005=ORIENTED_EDGE('',*,*,#8952,.T.);
#12006=ORIENTED_EDGE('',*,*,#8948,.T.);
#12007=ORIENTED_EDGE('',*,*,#8953,.T.);
#12008=ORIENTED_EDGE('',*,*,#8954,.F.);
#12009=ORIENTED_EDGE('',*,*,#8955,.T.);
#12010=ORIENTED_EDGE('',*,*,#8951,.T.);
#12011=ORIENTED_EDGE('',*,*,#8956,.T.);
#12012=ORIENTED_EDGE('',*,*,#8957,.F.);
#12013=ORIENTED_EDGE('',*,*,#8958,.T.);
#12014=ORIENTED_EDGE('',*,*,#8954,.T.);
#12015=ORIENTED_EDGE('',*,*,#8959,.T.);
#12016=ORIENTED_EDGE('',*,*,#8960,.F.);
#12017=ORIENTED_EDGE('',*,*,#8961,.T.);
#12018=ORIENTED_EDGE('',*,*,#8957,.T.);
#12019=ORIENTED_EDGE('',*,*,#8962,.T.);
#12020=ORIENTED_EDGE('',*,*,#8963,.F.);
#12021=ORIENTED_EDGE('',*,*,#8964,.T.);
#12022=ORIENTED_EDGE('',*,*,#8960,.T.);
#12023=ORIENTED_EDGE('',*,*,#8965,.T.);
#12024=ORIENTED_EDGE('',*,*,#8966,.F.);
#12025=ORIENTED_EDGE('',*,*,#8967,.T.);
#12026=ORIENTED_EDGE('',*,*,#8963,.T.);
#12027=ORIENTED_EDGE('',*,*,#8968,.T.);
#12028=ORIENTED_EDGE('',*,*,#8969,.F.);
#12029=ORIENTED_EDGE('',*,*,#8970,.T.);
#12030=ORIENTED_EDGE('',*,*,#8971,.F.);
#12031=ORIENTED_EDGE('',*,*,#8972,.F.);
#12032=ORIENTED_EDGE('',*,*,#8973,.F.);
#12033=ORIENTED_EDGE('',*,*,#8974,.T.);
#12034=ORIENTED_EDGE('',*,*,#8969,.T.);
#12035=ORIENTED_EDGE('',*,*,#8975,.F.);
#12036=ORIENTED_EDGE('',*,*,#8976,.F.);
#12037=ORIENTED_EDGE('',*,*,#8977,.T.);
#12038=ORIENTED_EDGE('',*,*,#8973,.T.);
#12039=ORIENTED_EDGE('',*,*,#8978,.F.);
#12040=ORIENTED_EDGE('',*,*,#8979,.F.);
#12041=ORIENTED_EDGE('',*,*,#8980,.T.);
#12042=ORIENTED_EDGE('',*,*,#8976,.T.);
#12043=ORIENTED_EDGE('',*,*,#8981,.F.);
#12044=ORIENTED_EDGE('',*,*,#8982,.F.);
#12045=ORIENTED_EDGE('',*,*,#8983,.T.);
#12046=ORIENTED_EDGE('',*,*,#8979,.T.);
#12047=ORIENTED_EDGE('',*,*,#8984,.F.);
#12048=ORIENTED_EDGE('',*,*,#8985,.F.);
#12049=ORIENTED_EDGE('',*,*,#8986,.T.);
#12050=ORIENTED_EDGE('',*,*,#8982,.T.);
#12051=ORIENTED_EDGE('',*,*,#8987,.F.);
#12052=ORIENTED_EDGE('',*,*,#8988,.F.);
#12053=ORIENTED_EDGE('',*,*,#8989,.T.);
#12054=ORIENTED_EDGE('',*,*,#8985,.T.);
#12055=ORIENTED_EDGE('',*,*,#8990,.F.);
#12056=ORIENTED_EDGE('',*,*,#8991,.F.);
#12057=ORIENTED_EDGE('',*,*,#8992,.T.);
#12058=ORIENTED_EDGE('',*,*,#8988,.T.);
#12059=ORIENTED_EDGE('',*,*,#8993,.F.);
#12060=ORIENTED_EDGE('',*,*,#8994,.F.);
#12061=ORIENTED_EDGE('',*,*,#8995,.T.);
#12062=ORIENTED_EDGE('',*,*,#8991,.T.);
#12063=ORIENTED_EDGE('',*,*,#8996,.F.);
#12064=ORIENTED_EDGE('',*,*,#8997,.F.);
#12065=ORIENTED_EDGE('',*,*,#8998,.T.);
#12066=ORIENTED_EDGE('',*,*,#8994,.T.);
#12067=ORIENTED_EDGE('',*,*,#8999,.F.);
#12068=ORIENTED_EDGE('',*,*,#9000,.F.);
#12069=ORIENTED_EDGE('',*,*,#9001,.T.);
#12070=ORIENTED_EDGE('',*,*,#8997,.T.);
#12071=ORIENTED_EDGE('',*,*,#9002,.F.);
#12072=ORIENTED_EDGE('',*,*,#9003,.F.);
#12073=ORIENTED_EDGE('',*,*,#9004,.T.);
#12074=ORIENTED_EDGE('',*,*,#9000,.T.);
#12075=ORIENTED_EDGE('',*,*,#9005,.F.);
#12076=ORIENTED_EDGE('',*,*,#9006,.F.);
#12077=ORIENTED_EDGE('',*,*,#9007,.T.);
#12078=ORIENTED_EDGE('',*,*,#9003,.T.);
#12079=ORIENTED_EDGE('',*,*,#9008,.F.);
#12080=ORIENTED_EDGE('',*,*,#9009,.F.);
#12081=ORIENTED_EDGE('',*,*,#9010,.T.);
#12082=ORIENTED_EDGE('',*,*,#9006,.T.);
#12083=ORIENTED_EDGE('',*,*,#9011,.F.);
#12084=ORIENTED_EDGE('',*,*,#9012,.F.);
#12085=ORIENTED_EDGE('',*,*,#9013,.T.);
#12086=ORIENTED_EDGE('',*,*,#9009,.T.);
#12087=ORIENTED_EDGE('',*,*,#9014,.F.);
#12088=ORIENTED_EDGE('',*,*,#8971,.T.);
#12089=ORIENTED_EDGE('',*,*,#9015,.T.);
#12090=ORIENTED_EDGE('',*,*,#9016,.F.);
#12091=ORIENTED_EDGE('',*,*,#9017,.F.);
#12092=ORIENTED_EDGE('',*,*,#9018,.T.);
#12093=ORIENTED_EDGE('',*,*,#9018,.F.);
#12094=ORIENTED_EDGE('',*,*,#9019,.F.);
#12095=ORIENTED_EDGE('',*,*,#8968,.F.);
#12096=ORIENTED_EDGE('',*,*,#8965,.F.);
#12097=ORIENTED_EDGE('',*,*,#8962,.F.);
#12098=ORIENTED_EDGE('',*,*,#8959,.F.);
#12099=ORIENTED_EDGE('',*,*,#8956,.F.);
#12100=ORIENTED_EDGE('',*,*,#8953,.F.);
#12101=ORIENTED_EDGE('',*,*,#8950,.F.);
#12102=ORIENTED_EDGE('',*,*,#8947,.F.);
#12103=ORIENTED_EDGE('',*,*,#8944,.F.);
#12104=ORIENTED_EDGE('',*,*,#8941,.F.);
#12105=ORIENTED_EDGE('',*,*,#8938,.F.);
#12106=ORIENTED_EDGE('',*,*,#8935,.F.);
#12107=ORIENTED_EDGE('',*,*,#8932,.F.);
#12108=ORIENTED_EDGE('',*,*,#8929,.F.);
#12109=ORIENTED_EDGE('',*,*,#8926,.F.);
#12110=ORIENTED_EDGE('',*,*,#9020,.F.);
#12111=ORIENTED_EDGE('',*,*,#9021,.T.);
#12112=ORIENTED_EDGE('',*,*,#9014,.T.);
#12113=ORIENTED_EDGE('',*,*,#9011,.T.);
#12114=ORIENTED_EDGE('',*,*,#9008,.T.);
#12115=ORIENTED_EDGE('',*,*,#9005,.T.);
#12116=ORIENTED_EDGE('',*,*,#9002,.T.);
#12117=ORIENTED_EDGE('',*,*,#8999,.T.);
#12118=ORIENTED_EDGE('',*,*,#8996,.T.);
#12119=ORIENTED_EDGE('',*,*,#8993,.T.);
#12120=ORIENTED_EDGE('',*,*,#8990,.T.);
#12121=ORIENTED_EDGE('',*,*,#8987,.T.);
#12122=ORIENTED_EDGE('',*,*,#8984,.T.);
#12123=ORIENTED_EDGE('',*,*,#8981,.T.);
#12124=ORIENTED_EDGE('',*,*,#8978,.T.);
#12125=ORIENTED_EDGE('',*,*,#8975,.T.);
#12126=ORIENTED_EDGE('',*,*,#8972,.T.);
#12127=ORIENTED_EDGE('',*,*,#9012,.T.);
#12128=ORIENTED_EDGE('',*,*,#9021,.F.);
#12129=ORIENTED_EDGE('',*,*,#9022,.F.);
#12130=ORIENTED_EDGE('',*,*,#9023,.T.);
#12131=ORIENTED_EDGE('',*,*,#9015,.F.);
#12132=ORIENTED_EDGE('',*,*,#8970,.F.);
#12133=ORIENTED_EDGE('',*,*,#8974,.F.);
#12134=ORIENTED_EDGE('',*,*,#8977,.F.);
#12135=ORIENTED_EDGE('',*,*,#8980,.F.);
#12136=ORIENTED_EDGE('',*,*,#8983,.F.);
#12137=ORIENTED_EDGE('',*,*,#8986,.F.);
#12138=ORIENTED_EDGE('',*,*,#8989,.F.);
#12139=ORIENTED_EDGE('',*,*,#8992,.F.);
#12140=ORIENTED_EDGE('',*,*,#8995,.F.);
#12141=ORIENTED_EDGE('',*,*,#8998,.F.);
#12142=ORIENTED_EDGE('',*,*,#9001,.F.);
#12143=ORIENTED_EDGE('',*,*,#9004,.F.);
#12144=ORIENTED_EDGE('',*,*,#9007,.F.);
#12145=ORIENTED_EDGE('',*,*,#9010,.F.);
#12146=ORIENTED_EDGE('',*,*,#9013,.F.);
#12147=ORIENTED_EDGE('',*,*,#9023,.F.);
#12148=ORIENTED_EDGE('',*,*,#9024,.F.);
#12149=ORIENTED_EDGE('',*,*,#8924,.F.);
#12150=ORIENTED_EDGE('',*,*,#8928,.F.);
#12151=ORIENTED_EDGE('',*,*,#8931,.F.);
#12152=ORIENTED_EDGE('',*,*,#8934,.F.);
#12153=ORIENTED_EDGE('',*,*,#8937,.F.);
#12154=ORIENTED_EDGE('',*,*,#8940,.F.);
#12155=ORIENTED_EDGE('',*,*,#8943,.F.);
#12156=ORIENTED_EDGE('',*,*,#8946,.F.);
#12157=ORIENTED_EDGE('',*,*,#8949,.F.);
#12158=ORIENTED_EDGE('',*,*,#8952,.F.);
#12159=ORIENTED_EDGE('',*,*,#8955,.F.);
#12160=ORIENTED_EDGE('',*,*,#8958,.F.);
#12161=ORIENTED_EDGE('',*,*,#8961,.F.);
#12162=ORIENTED_EDGE('',*,*,#8964,.F.);
#12163=ORIENTED_EDGE('',*,*,#8967,.F.);
#12164=ORIENTED_EDGE('',*,*,#9025,.F.);
#12165=ORIENTED_EDGE('',*,*,#8966,.T.);
#12166=ORIENTED_EDGE('',*,*,#9019,.T.);
#12167=ORIENTED_EDGE('',*,*,#9026,.F.);
#12168=ORIENTED_EDGE('',*,*,#9025,.T.);
#12169=ORIENTED_EDGE('',*,*,#9027,.F.);
#12170=ORIENTED_EDGE('',*,*,#9028,.F.);
#12171=ORIENTED_EDGE('',*,*,#8876,.F.);
#12172=ORIENTED_EDGE('',*,*,#8873,.F.);
#12173=ORIENTED_EDGE('',*,*,#8870,.F.);
#12174=ORIENTED_EDGE('',*,*,#8867,.F.);
#12175=ORIENTED_EDGE('',*,*,#8864,.F.);
#12176=ORIENTED_EDGE('',*,*,#8861,.F.);
#12177=ORIENTED_EDGE('',*,*,#8858,.F.);
#12178=ORIENTED_EDGE('',*,*,#8855,.F.);
#12179=ORIENTED_EDGE('',*,*,#8852,.F.);
#12180=ORIENTED_EDGE('',*,*,#8849,.F.);
#12181=ORIENTED_EDGE('',*,*,#8846,.F.);
#12182=ORIENTED_EDGE('',*,*,#8843,.F.);
#12183=ORIENTED_EDGE('',*,*,#8840,.F.);
#12184=ORIENTED_EDGE('',*,*,#8837,.F.);
#12185=ORIENTED_EDGE('',*,*,#8834,.F.);
#12186=ORIENTED_EDGE('',*,*,#9029,.F.);
#12187=ORIENTED_EDGE('',*,*,#9030,.T.);
#12188=ORIENTED_EDGE('',*,*,#8922,.T.);
#12189=ORIENTED_EDGE('',*,*,#8919,.T.);
#12190=ORIENTED_EDGE('',*,*,#8916,.T.);
#12191=ORIENTED_EDGE('',*,*,#8913,.T.);
#12192=ORIENTED_EDGE('',*,*,#8910,.T.);
#12193=ORIENTED_EDGE('',*,*,#8907,.T.);
#12194=ORIENTED_EDGE('',*,*,#8904,.T.);
#12195=ORIENTED_EDGE('',*,*,#8901,.T.);
#12196=ORIENTED_EDGE('',*,*,#8898,.T.);
#12197=ORIENTED_EDGE('',*,*,#8895,.T.);
#12198=ORIENTED_EDGE('',*,*,#8892,.T.);
#12199=ORIENTED_EDGE('',*,*,#8889,.T.);
#12200=ORIENTED_EDGE('',*,*,#8886,.T.);
#12201=ORIENTED_EDGE('',*,*,#8883,.T.);
#12202=ORIENTED_EDGE('',*,*,#8880,.T.);
#12203=ORIENTED_EDGE('',*,*,#9031,.T.);
#12204=ORIENTED_EDGE('',*,*,#9032,.T.);
#12205=ORIENTED_EDGE('',*,*,#9033,.T.);
#12206=ORIENTED_EDGE('',*,*,#9034,.T.);
#12207=ORIENTED_EDGE('',*,*,#9029,.T.);
#12208=ORIENTED_EDGE('',*,*,#8920,.T.);
#12209=ORIENTED_EDGE('',*,*,#9030,.F.);
#12210=ORIENTED_EDGE('',*,*,#9034,.F.);
#12211=ORIENTED_EDGE('',*,*,#9035,.T.);
#12212=ORIENTED_EDGE('',*,*,#9036,.F.);
#12213=ORIENTED_EDGE('',*,*,#8878,.F.);
#12214=ORIENTED_EDGE('',*,*,#8882,.F.);
#12215=ORIENTED_EDGE('',*,*,#8885,.F.);
#12216=ORIENTED_EDGE('',*,*,#8888,.F.);
#12217=ORIENTED_EDGE('',*,*,#8891,.F.);
#12218=ORIENTED_EDGE('',*,*,#8894,.F.);
#12219=ORIENTED_EDGE('',*,*,#8897,.F.);
#12220=ORIENTED_EDGE('',*,*,#8900,.F.);
#12221=ORIENTED_EDGE('',*,*,#8903,.F.);
#12222=ORIENTED_EDGE('',*,*,#8906,.F.);
#12223=ORIENTED_EDGE('',*,*,#8909,.F.);
#12224=ORIENTED_EDGE('',*,*,#8912,.F.);
#12225=ORIENTED_EDGE('',*,*,#8915,.F.);
#12226=ORIENTED_EDGE('',*,*,#8918,.F.);
#12227=ORIENTED_EDGE('',*,*,#8921,.F.);
#12228=ORIENTED_EDGE('',*,*,#9035,.F.);
#12229=ORIENTED_EDGE('',*,*,#9033,.F.);
#12230=ORIENTED_EDGE('',*,*,#8832,.F.);
#12231=ORIENTED_EDGE('',*,*,#8836,.F.);
#12232=ORIENTED_EDGE('',*,*,#8839,.F.);
#12233=ORIENTED_EDGE('',*,*,#8842,.F.);
#12234=ORIENTED_EDGE('',*,*,#8845,.F.);
#12235=ORIENTED_EDGE('',*,*,#8848,.F.);
#12236=ORIENTED_EDGE('',*,*,#8851,.F.);
#12237=ORIENTED_EDGE('',*,*,#8854,.F.);
#12238=ORIENTED_EDGE('',*,*,#8857,.F.);
#12239=ORIENTED_EDGE('',*,*,#8860,.F.);
#12240=ORIENTED_EDGE('',*,*,#8863,.F.);
#12241=ORIENTED_EDGE('',*,*,#8866,.F.);
#12242=ORIENTED_EDGE('',*,*,#8869,.F.);
#12243=ORIENTED_EDGE('',*,*,#8872,.F.);
#12244=ORIENTED_EDGE('',*,*,#8875,.F.);
#12245=ORIENTED_EDGE('',*,*,#9037,.F.);
#12246=ORIENTED_EDGE('',*,*,#9038,.F.);
#12247=ORIENTED_EDGE('',*,*,#9031,.F.);
#12248=ORIENTED_EDGE('',*,*,#8833,.F.);
#12249=ORIENTED_EDGE('',*,*,#9032,.F.);
#12250=ORIENTED_EDGE('',*,*,#9039,.T.);
#12251=ORIENTED_EDGE('',*,*,#9038,.T.);
#12252=ORIENTED_EDGE('',*,*,#9039,.F.);
#12253=ORIENTED_EDGE('',*,*,#8874,.T.);
#12254=ORIENTED_EDGE('',*,*,#9028,.T.);
#12255=ORIENTED_EDGE('',*,*,#9040,.F.);
#12256=ORIENTED_EDGE('',*,*,#9037,.T.);
#12257=ORIENTED_EDGE('',*,*,#9041,.F.);
#12258=ORIENTED_EDGE('',*,*,#9040,.T.);
#12259=ORIENTED_EDGE('',*,*,#9027,.T.);
#12260=ORIENTED_EDGE('',*,*,#8879,.T.);
#12261=ORIENTED_EDGE('',*,*,#9036,.T.);
#12262=ORIENTED_EDGE('',*,*,#9042,.F.);
#12263=ORIENTED_EDGE('',*,*,#9043,.T.);
#12264=ORIENTED_EDGE('',*,*,#9041,.T.);
#12265=ORIENTED_EDGE('',*,*,#9043,.F.);
#12266=ORIENTED_EDGE('',*,*,#9042,.T.);
#12267=ORIENTED_EDGE('',*,*,#9024,.T.);
#12268=ORIENTED_EDGE('',*,*,#9022,.T.);
#12269=ORIENTED_EDGE('',*,*,#9020,.T.);
#12270=ORIENTED_EDGE('',*,*,#8925,.F.);
#12271=ORIENTED_EDGE('',*,*,#9044,.F.);
#12272=ORIENTED_EDGE('',*,*,#9045,.T.);
#12273=ORIENTED_EDGE('',*,*,#9016,.T.);
#12274=ORIENTED_EDGE('',*,*,#9026,.T.);
#12275=ORIENTED_EDGE('',*,*,#9017,.T.);
#12276=ORIENTED_EDGE('',*,*,#9045,.F.);
#12277=ORIENTED_EDGE('',*,*,#9044,.T.);
#15783=PLANE('',#17749);
#15784=PLANE('',#17756);
#15785=PLANE('',#17761);
#15786=PLANE('',#17766);
#15787=PLANE('',#17770);
#15788=PLANE('',#17773);
#16200=ADVANCED_FACE('',(#2029),#1321,.T.);
#16201=ADVANCED_FACE('',(#2030),#1322,.T.);
#16202=ADVANCED_FACE('',(#2031),#1323,.T.);
#16203=ADVANCED_FACE('',(#2032),#1324,.T.);
#16204=ADVANCED_FACE('',(#2033),#1325,.T.);
#16205=ADVANCED_FACE('',(#2034),#1326,.T.);
#16206=ADVANCED_FACE('',(#2035),#1327,.T.);
#16207=ADVANCED_FACE('',(#2036),#1328,.T.);
#16208=ADVANCED_FACE('',(#2037),#1329,.T.);
#16209=ADVANCED_FACE('',(#2038),#1330,.T.);
#16210=ADVANCED_FACE('',(#2039),#1331,.T.);
#16211=ADVANCED_FACE('',(#2040),#1332,.T.);
#16212=ADVANCED_FACE('',(#2041),#1333,.T.);
#16213=ADVANCED_FACE('',(#2042),#1334,.T.);
#16214=ADVANCED_FACE('',(#2043),#1335,.T.);
#16215=ADVANCED_FACE('',(#2044),#1336,.T.);
#16216=ADVANCED_FACE('',(#2045),#1337,.T.);
#16217=ADVANCED_FACE('',(#2046),#1338,.T.);
#16218=ADVANCED_FACE('',(#2047),#1339,.T.);
#16219=ADVANCED_FACE('',(#2048),#1340,.T.);
#16220=ADVANCED_FACE('',(#2049),#1341,.T.);
#16221=ADVANCED_FACE('',(#2050),#1342,.T.);
#16222=ADVANCED_FACE('',(#2051),#1343,.T.);
#16223=ADVANCED_FACE('',(#2052),#1344,.T.);
#16224=ADVANCED_FACE('',(#2053),#1345,.T.);
#16225=ADVANCED_FACE('',(#2054),#1346,.T.);
#16226=ADVANCED_FACE('',(#2055),#1347,.T.);
#16227=ADVANCED_FACE('',(#2056),#1348,.T.);
#16228=ADVANCED_FACE('',(#2057),#1349,.T.);
#16229=ADVANCED_FACE('',(#2058),#1350,.T.);
#16230=ADVANCED_FACE('',(#2059),#1351,.T.);
#16231=ADVANCED_FACE('',(#2060),#1352,.T.);
#16232=ADVANCED_FACE('',(#2061),#1353,.T.);
#16233=ADVANCED_FACE('',(#2062),#1354,.T.);
#16234=ADVANCED_FACE('',(#2063),#1355,.T.);
#16235=ADVANCED_FACE('',(#2064),#1356,.T.);
#16236=ADVANCED_FACE('',(#2065),#1357,.T.);
#16237=ADVANCED_FACE('',(#2066),#1358,.T.);
#16238=ADVANCED_FACE('',(#2067),#1359,.T.);
#16239=ADVANCED_FACE('',(#2068),#1360,.T.);
#16240=ADVANCED_FACE('',(#2069),#1361,.T.);
#16241=ADVANCED_FACE('',(#2070),#1362,.T.);
#16242=ADVANCED_FACE('',(#2071),#1363,.T.);
#16243=ADVANCED_FACE('',(#2072),#1364,.T.);
#16244=ADVANCED_FACE('',(#2073),#1365,.T.);
#16245=ADVANCED_FACE('',(#2074),#1366,.T.);
#16246=ADVANCED_FACE('',(#2075),#1367,.T.);
#16247=ADVANCED_FACE('',(#2076),#1368,.T.);
#16248=ADVANCED_FACE('',(#2077),#1369,.T.);
#16249=ADVANCED_FACE('',(#2078),#1370,.T.);
#16250=ADVANCED_FACE('',(#2079),#1371,.T.);
#16251=ADVANCED_FACE('',(#2080),#1372,.T.);
#16252=ADVANCED_FACE('',(#2081),#1373,.T.);
#16253=ADVANCED_FACE('',(#2082),#1374,.T.);
#16254=ADVANCED_FACE('',(#2083),#1375,.T.);
#16255=ADVANCED_FACE('',(#2084),#1376,.T.);
#16256=ADVANCED_FACE('',(#2085),#1377,.T.);
#16257=ADVANCED_FACE('',(#2086),#1378,.T.);
#16258=ADVANCED_FACE('',(#2087),#1379,.T.);
#16259=ADVANCED_FACE('',(#2088),#1380,.T.);
#16260=ADVANCED_FACE('',(#2089),#15783,.F.);
#16261=ADVANCED_FACE('',(#2090),#339,.F.);
#16262=ADVANCED_FACE('',(#2091),#1381,.T.);
#16263=ADVANCED_FACE('',(#2092),#340,.F.);
#16264=ADVANCED_FACE('',(#2093),#1382,.T.);
#16265=ADVANCED_FACE('',(#2094),#341,.F.);
#16266=ADVANCED_FACE('',(#2095),#15784,.T.);
#16267=ADVANCED_FACE('',(#2096),#1383,.T.);
#16268=ADVANCED_FACE('',(#2097),#342,.F.);
#16269=ADVANCED_FACE('',(#2098),#15785,.T.);
#16270=ADVANCED_FACE('',(#2099),#595,.T.);
#16271=ADVANCED_FACE('',(#2100),#1384,.T.);
#16272=ADVANCED_FACE('',(#2101,#510),#15786,.T.);
#16273=ADVANCED_FACE('',(#2102),#1385,.T.);
#16274=ADVANCED_FACE('',(#2103,#511),#15787,.T.);
#16275=ADVANCED_FACE('',(#2104),#596,.T.);
#16276=ADVANCED_FACE('',(#2105),#15788,.T.);
#16956=CLOSED_SHELL('',(#16200,#16201,#16202,#16203,#16204,#16205,#16206,
#16207,#16208,#16209,#16210,#16211,#16212,#16213,#16214,#16215,#16216,#16217,
#16218,#16219,#16220,#16221,#16222,#16223,#16224,#16225,#16226,#16227,#16228,
#16229,#16230,#16231,#16232,#16233,#16234,#16235,#16236,#16237,#16238,#16239,
#16240,#16241,#16242,#16243,#16244,#16245,#16246,#16247,#16248,#16249,#16250,
#16251,#16252,#16253,#16254,#16255,#16256,#16257,#16258,#16259,#16260,#16261,
#16262,#16263,#16264,#16265,#16266,#16267,#16268,#16269,#16270,#16271,#16272,
#16273,#16274,#16275,#16276));
#17684=AXIS2_PLACEMENT_3D('',#25121,#19979,#19980);
#17685=AXIS2_PLACEMENT_3D('',#25122,#19981,#19982);
#17686=AXIS2_PLACEMENT_3D('',#25144,#19984,#19985);
#17687=AXIS2_PLACEMENT_3D('',#25155,#19986,#19987);
#17688=AXIS2_PLACEMENT_3D('',#25239,#19989,#19990);
#17689=AXIS2_PLACEMENT_3D('',#25329,#19992,#19993);
#17690=AXIS2_PLACEMENT_3D('',#25419,#19995,#19996);
#17691=AXIS2_PLACEMENT_3D('',#25503,#19998,#19999);
#17692=AXIS2_PLACEMENT_3D('',#25593,#20001,#20002);
#17693=AXIS2_PLACEMENT_3D('',#25677,#20004,#20005);
#17694=AXIS2_PLACEMENT_3D('',#25764,#20007,#20008);
#17695=AXIS2_PLACEMENT_3D('',#25839,#20010,#20011);
#17696=AXIS2_PLACEMENT_3D('',#25923,#20013,#20014);
#17697=AXIS2_PLACEMENT_3D('',#26013,#20016,#20017);
#17698=AXIS2_PLACEMENT_3D('',#26097,#20019,#20020);
#17699=AXIS2_PLACEMENT_3D('',#26184,#20022,#20023);
#17700=AXIS2_PLACEMENT_3D('',#26274,#20025,#20026);
#17701=AXIS2_PLACEMENT_3D('',#26358,#20028,#20029);
#17702=AXIS2_PLACEMENT_3D('',#26373,#20031,#20032);
#17703=AXIS2_PLACEMENT_3D('',#26380,#20033,#20034);
#17704=AXIS2_PLACEMENT_3D('',#26417,#20036,#20037);
#17705=AXIS2_PLACEMENT_3D('',#26454,#20039,#20040);
#17706=AXIS2_PLACEMENT_3D('',#26492,#20042,#20043);
#17707=AXIS2_PLACEMENT_3D('',#26529,#20045,#20046);
#17708=AXIS2_PLACEMENT_3D('',#26566,#20048,#20049);
#17709=AXIS2_PLACEMENT_3D('',#26603,#20051,#20052);
#17710=AXIS2_PLACEMENT_3D('',#26638,#20054,#20055);
#17711=AXIS2_PLACEMENT_3D('',#26672,#20057,#20058);
#17712=AXIS2_PLACEMENT_3D('',#26709,#20060,#20061);
#17713=AXIS2_PLACEMENT_3D('',#26746,#20063,#20064);
#17714=AXIS2_PLACEMENT_3D('',#26783,#20066,#20067);
#17715=AXIS2_PLACEMENT_3D('',#26820,#20069,#20070);
#17716=AXIS2_PLACEMENT_3D('',#26858,#20072,#20073);
#17717=AXIS2_PLACEMENT_3D('',#26895,#20075,#20076);
#17718=AXIS2_PLACEMENT_3D('',#26917,#20078,#20079);
#17719=AXIS2_PLACEMENT_3D('',#26928,#20080,#20081);
#17720=AXIS2_PLACEMENT_3D('',#27012,#20083,#20084);
#17721=AXIS2_PLACEMENT_3D('',#27102,#20086,#20087);
#17722=AXIS2_PLACEMENT_3D('',#27192,#20089,#20090);
#17723=AXIS2_PLACEMENT_3D('',#27276,#20092,#20093);
#17724=AXIS2_PLACEMENT_3D('',#27366,#20095,#20096);
#17725=AXIS2_PLACEMENT_3D('',#27450,#20098,#20099);
#17726=AXIS2_PLACEMENT_3D('',#27537,#20101,#20102);
#17727=AXIS2_PLACEMENT_3D('',#27612,#20104,#20105);
#17728=AXIS2_PLACEMENT_3D('',#27696,#20107,#20108);
#17729=AXIS2_PLACEMENT_3D('',#27786,#20110,#20111);
#17730=AXIS2_PLACEMENT_3D('',#27870,#20113,#20114);
#17731=AXIS2_PLACEMENT_3D('',#27957,#20116,#20117);
#17732=AXIS2_PLACEMENT_3D('',#28047,#20119,#20120);
#17733=AXIS2_PLACEMENT_3D('',#28131,#20122,#20123);
#17734=AXIS2_PLACEMENT_3D('',#28146,#20125,#20126);
#17735=AXIS2_PLACEMENT_3D('',#28153,#20127,#20128);
#17736=AXIS2_PLACEMENT_3D('',#28190,#20130,#20131);
#17737=AXIS2_PLACEMENT_3D('',#28227,#20133,#20134);
#17738=AXIS2_PLACEMENT_3D('',#28265,#20136,#20137);
#17739=AXIS2_PLACEMENT_3D('',#28302,#20139,#20140);
#17740=AXIS2_PLACEMENT_3D('',#28339,#20142,#20143);
#17741=AXIS2_PLACEMENT_3D('',#28376,#20145,#20146);
#17742=AXIS2_PLACEMENT_3D('',#28411,#20148,#20149);
#17743=AXIS2_PLACEMENT_3D('',#28445,#20151,#20152);
#17744=AXIS2_PLACEMENT_3D('',#28482,#20154,#20155);
#17745=AXIS2_PLACEMENT_3D('',#28519,#20157,#20158);
#17746=AXIS2_PLACEMENT_3D('',#28556,#20160,#20161);
#17747=AXIS2_PLACEMENT_3D('',#28593,#20163,#20164);
#17748=AXIS2_PLACEMENT_3D('',#28631,#20166,#20167);
#17749=AXIS2_PLACEMENT_3D('',#28668,#20169,#20170);
#17750=AXIS2_PLACEMENT_3D('',#28783,#20171,#20172);
#17751=AXIS2_PLACEMENT_3D('',#28785,#20173,#20174);
#17752=AXIS2_PLACEMENT_3D('',#29835,#20175,#20176);
#17753=AXIS2_PLACEMENT_3D('',#29837,#20177,#20178);
#17754=AXIS2_PLACEMENT_3D('',#30766,#20179,#20180);
#17755=AXIS2_PLACEMENT_3D('',#30767,#20181,#20182);
#17756=AXIS2_PLACEMENT_3D('',#31818,#20183,#20184);
#17757=AXIS2_PLACEMENT_3D('',#31820,#20185,#20186);
#17758=AXIS2_PLACEMENT_3D('',#31821,#20187,#20188);
#17759=AXIS2_PLACEMENT_3D('',#31932,#20189,#20190);
#17760=AXIS2_PLACEMENT_3D('',#31933,#20191,#20192);
#17761=AXIS2_PLACEMENT_3D('',#32866,#20193,#20194);
#17762=AXIS2_PLACEMENT_3D('',#32868,#20195,#20196);
#17763=AXIS2_PLACEMENT_3D('',#32869,#20197,#20198);
#17764=AXIS2_PLACEMENT_3D('',#32871,#20200,#20201);
#17765=AXIS2_PLACEMENT_3D('',#32872,#20202,#20203);
#17766=AXIS2_PLACEMENT_3D('',#32873,#20204,#20205);
#17767=AXIS2_PLACEMENT_3D('',#32875,#20206,#20207);
#17768=AXIS2_PLACEMENT_3D('',#32876,#20208,#20209);
#17769=AXIS2_PLACEMENT_3D('',#32878,#20210,#20211);
#17770=AXIS2_PLACEMENT_3D('',#32880,#20213,#20214);
#17771=AXIS2_PLACEMENT_3D('',#32881,#20215,#20216);
#17772=AXIS2_PLACEMENT_3D('',#32883,#20217,#20218);
#17773=AXIS2_PLACEMENT_3D('',#32885,#20220,#20221);
#19979=DIRECTION('axis',(0.,0.,1.));
#19980=DIRECTION('refdir',(1.,0.,0.));
#19981=DIRECTION('center_axis',(1.,0.,0.));
#19982=DIRECTION('ref_axis',(0.,1.,0.));
#19983=DIRECTION('',(-1.,0.,0.));
#19984=DIRECTION('center_axis',(1.,0.,0.));
#19985=DIRECTION('ref_axis',(0.,1.,0.));
#19986=DIRECTION('center_axis',(1.,0.,0.));
#19987=DIRECTION('ref_axis',(0.,1.,0.));
#19988=DIRECTION('',(-1.,0.,0.));
#19989=DIRECTION('center_axis',(1.,0.,0.));
#19990=DIRECTION('ref_axis',(0.,1.,0.));
#19991=DIRECTION('',(-1.,0.,0.));
#19992=DIRECTION('center_axis',(1.,0.,0.));
#19993=DIRECTION('ref_axis',(0.,1.,0.));
#19994=DIRECTION('',(-1.,0.,0.));
#19995=DIRECTION('center_axis',(1.,0.,0.));
#19996=DIRECTION('ref_axis',(0.,1.,0.));
#19997=DIRECTION('',(-1.,0.,0.));
#19998=DIRECTION('center_axis',(1.,0.,0.));
#19999=DIRECTION('ref_axis',(0.,1.,0.));
#20000=DIRECTION('',(-1.,0.,0.));
#20001=DIRECTION('center_axis',(1.,0.,0.));
#20002=DIRECTION('ref_axis',(0.,1.,0.));
#20003=DIRECTION('',(-1.,0.,0.));
#20004=DIRECTION('center_axis',(1.,0.,0.));
#20005=DIRECTION('ref_axis',(0.,1.,0.));
#20006=DIRECTION('',(-1.,0.,0.));
#20007=DIRECTION('center_axis',(1.,0.,0.));
#20008=DIRECTION('ref_axis',(0.,1.,0.));
#20009=DIRECTION('',(-1.,0.,0.));
#20010=DIRECTION('center_axis',(1.,0.,0.));
#20011=DIRECTION('ref_axis',(0.,1.,0.));
#20012=DIRECTION('',(-1.,0.,0.));
#20013=DIRECTION('center_axis',(1.,0.,0.));
#20014=DIRECTION('ref_axis',(0.,1.,0.));
#20015=DIRECTION('',(-1.,0.,0.));
#20016=DIRECTION('center_axis',(1.,0.,0.));
#20017=DIRECTION('ref_axis',(0.,1.,0.));
#20018=DIRECTION('',(-1.,0.,0.));
#20019=DIRECTION('center_axis',(1.,0.,0.));
#20020=DIRECTION('ref_axis',(0.,1.,0.));
#20021=DIRECTION('',(-1.,0.,0.));
#20022=DIRECTION('center_axis',(1.,0.,0.));
#20023=DIRECTION('ref_axis',(0.,1.,0.));
#20024=DIRECTION('',(-1.,0.,0.));
#20025=DIRECTION('center_axis',(1.,0.,0.));
#20026=DIRECTION('ref_axis',(0.,1.,0.));
#20027=DIRECTION('',(-1.,0.,0.));
#20028=DIRECTION('center_axis',(1.,0.,0.));
#20029=DIRECTION('ref_axis',(0.,-0.313365996365904,-0.949632430112622));
#20030=DIRECTION('',(1.,0.,0.));
#20031=DIRECTION('center_axis',(1.,0.,0.));
#20032=DIRECTION('ref_axis',(0.,1.,8.41174344736429E-14));
#20033=DIRECTION('center_axis',(1.,0.,0.));
#20034=DIRECTION('ref_axis',(0.,1.,8.41174344736429E-14));
#20035=DIRECTION('',(1.,0.,0.));
#20036=DIRECTION('center_axis',(1.,0.,0.));
#20037=DIRECTION('ref_axis',(0.,1.,8.41174344736429E-14));
#20038=DIRECTION('',(1.,0.,0.));
#20039=DIRECTION('center_axis',(1.,0.,0.));
#20040=DIRECTION('ref_axis',(0.,1.,8.41174344736429E-14));
#20041=DIRECTION('',(1.,0.,0.));
#20042=DIRECTION('center_axis',(1.,0.,0.));
#20043=DIRECTION('ref_axis',(0.,1.,8.41174344736429E-14));
#20044=DIRECTION('',(1.,0.,0.));
#20045=DIRECTION('center_axis',(1.,0.,0.));
#20046=DIRECTION('ref_axis',(0.,1.,8.41174344736429E-14));
#20047=DIRECTION('',(1.,0.,0.));
#20048=DIRECTION('center_axis',(1.,0.,0.));
#20049=DIRECTION('ref_axis',(0.,1.,8.41174344736429E-14));
#20050=DIRECTION('',(1.,0.,0.));
#20051=DIRECTION('center_axis',(1.,0.,0.));
#20052=DIRECTION('ref_axis',(0.,1.,8.41174344736429E-14));
#20053=DIRECTION('',(1.,0.,0.));
#20054=DIRECTION('center_axis',(1.,0.,0.));
#20055=DIRECTION('ref_axis',(0.,1.,8.41174344736429E-14));
#20056=DIRECTION('',(1.,0.,0.));
#20057=DIRECTION('center_axis',(1.,0.,0.));
#20058=DIRECTION('ref_axis',(0.,1.,8.41174344736429E-14));
#20059=DIRECTION('',(1.,0.,0.));
#20060=DIRECTION('center_axis',(1.,0.,0.));
#20061=DIRECTION('ref_axis',(0.,1.,8.41174344736429E-14));
#20062=DIRECTION('',(1.,0.,0.));
#20063=DIRECTION('center_axis',(1.,0.,0.));
#20064=DIRECTION('ref_axis',(0.,1.,8.41174344736429E-14));
#20065=DIRECTION('',(1.,0.,0.));
#20066=DIRECTION('center_axis',(1.,0.,0.));
#20067=DIRECTION('ref_axis',(0.,1.,8.41174344736429E-14));
#20068=DIRECTION('',(1.,0.,0.));
#20069=DIRECTION('center_axis',(1.,0.,0.));
#20070=DIRECTION('ref_axis',(0.,1.,8.41174344736429E-14));
#20071=DIRECTION('',(1.,0.,0.));
#20072=DIRECTION('center_axis',(1.,0.,0.));
#20073=DIRECTION('ref_axis',(0.,1.,8.41174344736429E-14));
#20074=DIRECTION('',(1.,0.,0.));
#20075=DIRECTION('center_axis',(1.,0.,0.));
#20076=DIRECTION('ref_axis',(0.,1.,0.));
#20077=DIRECTION('',(-1.,0.,0.));
#20078=DIRECTION('center_axis',(-1.,0.,0.));
#20079=DIRECTION('ref_axis',(0.,1.,0.));
#20080=DIRECTION('center_axis',(1.,0.,0.));
#20081=DIRECTION('ref_axis',(0.,1.,0.));
#20082=DIRECTION('',(-1.,0.,0.));
#20083=DIRECTION('center_axis',(1.,0.,0.));
#20084=DIRECTION('ref_axis',(0.,1.,0.));
#20085=DIRECTION('',(-1.,0.,0.));
#20086=DIRECTION('center_axis',(1.,0.,0.));
#20087=DIRECTION('ref_axis',(0.,1.,0.));
#20088=DIRECTION('',(-1.,0.,0.));
#20089=DIRECTION('center_axis',(1.,0.,0.));
#20090=DIRECTION('ref_axis',(0.,1.,0.));
#20091=DIRECTION('',(-1.,0.,0.));
#20092=DIRECTION('center_axis',(1.,0.,0.));
#20093=DIRECTION('ref_axis',(0.,1.,0.));
#20094=DIRECTION('',(-1.,0.,0.));
#20095=DIRECTION('center_axis',(1.,0.,0.));
#20096=DIRECTION('ref_axis',(0.,1.,0.));
#20097=DIRECTION('',(-1.,0.,0.));
#20098=DIRECTION('center_axis',(1.,0.,0.));
#20099=DIRECTION('ref_axis',(0.,1.,0.));
#20100=DIRECTION('',(-1.,0.,0.));
#20101=DIRECTION('center_axis',(1.,0.,0.));
#20102=DIRECTION('ref_axis',(0.,1.,0.));
#20103=DIRECTION('',(-1.,0.,0.));
#20104=DIRECTION('center_axis',(1.,0.,0.));
#20105=DIRECTION('ref_axis',(0.,1.,0.));
#20106=DIRECTION('',(-1.,0.,0.));
#20107=DIRECTION('center_axis',(1.,0.,0.));
#20108=DIRECTION('ref_axis',(0.,1.,0.));
#20109=DIRECTION('',(-1.,0.,0.));
#20110=DIRECTION('center_axis',(1.,0.,0.));
#20111=DIRECTION('ref_axis',(0.,1.,0.));
#20112=DIRECTION('',(-1.,0.,0.));
#20113=DIRECTION('center_axis',(1.,0.,0.));
#20114=DIRECTION('ref_axis',(0.,1.,0.));
#20115=DIRECTION('',(-1.,0.,0.));
#20116=DIRECTION('center_axis',(1.,0.,0.));
#20117=DIRECTION('ref_axis',(0.,1.,0.));
#20118=DIRECTION('',(-1.,0.,0.));
#20119=DIRECTION('center_axis',(1.,0.,0.));
#20120=DIRECTION('ref_axis',(0.,1.,0.));
#20121=DIRECTION('',(-1.,0.,0.));
#20122=DIRECTION('center_axis',(1.,0.,0.));
#20123=DIRECTION('ref_axis',(0.,-0.313365995386845,-0.949632430435699));
#20124=DIRECTION('',(1.,0.,0.));
#20125=DIRECTION('center_axis',(1.,0.,0.));
#20126=DIRECTION('ref_axis',(0.,1.,8.41174344736429E-14));
#20127=DIRECTION('center_axis',(1.,0.,0.));
#20128=DIRECTION('ref_axis',(0.,1.,8.41174344736429E-14));
#20129=DIRECTION('',(1.,0.,0.));
#20130=DIRECTION('center_axis',(1.,0.,0.));
#20131=DIRECTION('ref_axis',(0.,1.,8.41174344736429E-14));
#20132=DIRECTION('',(1.,0.,0.));
#20133=DIRECTION('center_axis',(1.,0.,0.));
#20134=DIRECTION('ref_axis',(0.,1.,8.41174344736429E-14));
#20135=DIRECTION('',(1.,0.,0.));
#20136=DIRECTION('center_axis',(1.,0.,0.));
#20137=DIRECTION('ref_axis',(0.,1.,8.41174344736429E-14));
#20138=DIRECTION('',(1.,0.,0.));
#20139=DIRECTION('center_axis',(1.,0.,0.));
#20140=DIRECTION('ref_axis',(0.,1.,8.41174344736429E-14));
#20141=DIRECTION('',(1.,0.,0.));
#20142=DIRECTION('center_axis',(1.,0.,0.));
#20143=DIRECTION('ref_axis',(0.,1.,8.41174344736429E-14));
#20144=DIRECTION('',(1.,0.,0.));
#20145=DIRECTION('center_axis',(1.,0.,0.));
#20146=DIRECTION('ref_axis',(0.,1.,8.41174344736429E-14));
#20147=DIRECTION('',(1.,0.,0.));
#20148=DIRECTION('center_axis',(1.,0.,0.));
#20149=DIRECTION('ref_axis',(0.,1.,8.41174344736429E-14));
#20150=DIRECTION('',(1.,0.,0.));
#20151=DIRECTION('center_axis',(1.,0.,0.));
#20152=DIRECTION('ref_axis',(0.,1.,8.41174344736429E-14));
#20153=DIRECTION('',(1.,0.,0.));
#20154=DIRECTION('center_axis',(1.,0.,0.));
#20155=DIRECTION('ref_axis',(0.,1.,8.41174344736429E-14));
#20156=DIRECTION('',(1.,0.,0.));
#20157=DIRECTION('center_axis',(1.,0.,0.));
#20158=DIRECTION('ref_axis',(0.,1.,8.41174344736429E-14));
#20159=DIRECTION('',(1.,0.,0.));
#20160=DIRECTION('center_axis',(1.,0.,0.));
#20161=DIRECTION('ref_axis',(0.,1.,8.41174344736429E-14));
#20162=DIRECTION('',(1.,0.,0.));
#20163=DIRECTION('center_axis',(1.,0.,0.));
#20164=DIRECTION('ref_axis',(0.,1.,8.41174344736429E-14));
#20165=DIRECTION('',(1.,0.,0.));
#20166=DIRECTION('center_axis',(1.,0.,0.));
#20167=DIRECTION('ref_axis',(0.,1.,8.41174344736429E-14));
#20168=DIRECTION('',(1.,0.,0.));
#20169=DIRECTION('center_axis',(1.,0.,0.));
#20170=DIRECTION('ref_axis',(0.,0.,-1.));
#20171=DIRECTION('center_axis',(-1.,0.,0.));
#20172=DIRECTION('ref_axis',(0.,1.,0.));
#20173=DIRECTION('center_axis',(-1.,0.,0.));
#20174=DIRECTION('ref_axis',(0.,1.,0.));
#20175=DIRECTION('center_axis',(1.,0.,0.));
#20176=DIRECTION('ref_axis',(0.,0.888917223619435,0.458067865662629));
#20177=DIRECTION('center_axis',(-1.,0.,0.));
#20178=DIRECTION('ref_axis',(0.,1.,8.41174344736429E-14));
#20179=DIRECTION('center_axis',(1.,0.,0.));
#20180=DIRECTION('ref_axis',(0.,1.,0.));
#20181=DIRECTION('center_axis',(-1.,0.,0.));
#20182=DIRECTION('ref_axis',(0.,1.,0.));
#20183=DIRECTION('center_axis',(1.,0.,0.));
#20184=DIRECTION('ref_axis',(0.,0.,-1.));
#20185=DIRECTION('center_axis',(1.,0.,0.));
#20186=DIRECTION('ref_axis',(0.,1.,0.));
#20187=DIRECTION('center_axis',(1.,0.,0.));
#20188=DIRECTION('ref_axis',(0.,1.,0.));
#20189=DIRECTION('center_axis',(-1.,0.,0.));
#20190=DIRECTION('ref_axis',(0.,1.,8.41174344736429E-14));
#20191=DIRECTION('center_axis',(1.,0.,0.));
#20192=DIRECTION('ref_axis',(0.,0.888917222728707,0.458067867391156));
#20193=DIRECTION('center_axis',(-1.,0.,0.));
#20194=DIRECTION('ref_axis',(0.,0.,1.));
#20195=DIRECTION('center_axis',(1.,0.,0.));
#20196=DIRECTION('ref_axis',(0.,0.,-1.));
#20197=DIRECTION('center_axis',(1.,0.,0.));
#20198=DIRECTION('ref_axis',(0.,1.,0.));
#20199=DIRECTION('',(-0.707106781186546,0.707106781186549,8.65956056235495E-17));
#20200=DIRECTION('center_axis',(1.,0.,0.));
#20201=DIRECTION('ref_axis',(0.,1.,0.));
#20202=DIRECTION('center_axis',(1.,0.,0.));
#20203=DIRECTION('ref_axis',(0.,1.,0.));
#20204=DIRECTION('center_axis',(-1.,0.,0.));
#20205=DIRECTION('ref_axis',(0.,0.,1.));
#20206=DIRECTION('center_axis',(1.,0.,0.));
#20207=DIRECTION('ref_axis',(0.,0.,-1.));
#20208=DIRECTION('center_axis',(1.,0.,0.));
#20209=DIRECTION('ref_axis',(0.,1.,0.));
#20210=DIRECTION('center_axis',(1.,0.,0.));
#20211=DIRECTION('ref_axis',(0.,0.,-1.));
#20212=DIRECTION('',(-1.,0.,0.));
#20213=DIRECTION('center_axis',(1.,0.,0.));
#20214=DIRECTION('ref_axis',(0.,0.,-1.));
#20215=DIRECTION('center_axis',(-1.,0.,0.));
#20216=DIRECTION('ref_axis',(0.,1.,0.));
#20217=DIRECTION('center_axis',(1.,0.,0.));
#20218=DIRECTION('ref_axis',(0.,0.,-1.));
#20219=DIRECTION('',(-0.707106781186546,-0.707106781186549,-8.65956056235495E-17));
#20220=DIRECTION('center_axis',(1.,0.,0.));
#20221=DIRECTION('ref_axis',(0.,0.,-1.));
#25121=CARTESIAN_POINT('',(0.,0.,0.));
#25122=CARTESIAN_POINT('Origin',(-41.25,0.,0.));
#25123=CARTESIAN_POINT('',(-52.0911584740964,-4.92503359593706,0.000126434235863393));
#25124=CARTESIAN_POINT('',(-52.3088415259036,-4.92498877504697,8.594588268108E-5));
#25125=CARTESIAN_POINT('',(-41.25,-4.925,-6.03138548580071E-16));
#25126=CARTESIAN_POINT('',(-52.575,2.16848938207169,4.42202992386415));
#25127=CARTESIAN_POINT('Ctrl Pts',(-52.0911584740964,-4.92503359593706,
0.000126434235863393));
#25128=CARTESIAN_POINT('Ctrl Pts',(-52.0997969204186,-4.92521675924443,
0.178328848272776));
#25129=CARTESIAN_POINT('Ctrl Pts',(-52.1084353667407,-4.91573151990345,
0.356511816443558));
#25130=CARTESIAN_POINT('Ctrl Pts',(-52.1170738130628,-4.89642931932951,
0.533624833881526));
#25131=CARTESIAN_POINT('Ctrl Pts',(-52.1567101460612,-4.80786380407155,
1.3462837630126));
#25132=CARTESIAN_POINT('Ctrl Pts',(-52.1963464790595,-4.5126210099822,2.13641693282812));
#25133=CARTESIAN_POINT('Ctrl Pts',(-52.2359828120578,-4.04657310803694,
2.80802695734203));
#25134=CARTESIAN_POINT('Ctrl Pts',(-52.2756191450561,-3.58052520609168,
3.47963698185595));
#25135=CARTESIAN_POINT('Ctrl Pts',(-52.3152554780544,-2.94367219629051,
4.03272386106826));
#25136=CARTESIAN_POINT('Ctrl Pts',(-52.3548918110528,-2.21339245150104,
4.40007810178881));
#25137=CARTESIAN_POINT('Ctrl Pts',(-52.3945281440511,-1.48311270671156,
4.76743234250936));
#25138=CARTESIAN_POINT('Ctrl Pts',(-52.4341644770494,-0.659406226933773,
4.94905394473814));
#25139=CARTESIAN_POINT('Ctrl Pts',(-52.4738008100477,0.157646275526665,
4.92289359031672));
#25140=CARTESIAN_POINT('Ctrl Pts',(-52.5075338733652,0.853010395116791,
4.90062944968238));
#25141=CARTESIAN_POINT('Ctrl Pts',(-52.5412669366825,1.54355497078764,4.72786670979692));
#25142=CARTESIAN_POINT('Ctrl Pts',(-52.575,2.16858289183292,4.42210503781143));
#25143=CARTESIAN_POINT('',(-52.575,-2.16839587231069,4.42195480991676));
#25144=CARTESIAN_POINT('Origin',(-52.575,0.,0.));
#25145=CARTESIAN_POINT('Ctrl Pts',(-52.575,-2.16839587231068,4.42195480991676));
#25146=CARTESIAN_POINT('Ctrl Pts',(-52.5353636670017,-2.90256543874876,
4.06193976546849));
#25147=CARTESIAN_POINT('Ctrl Pts',(-52.4957273340034,-3.54497563996543,
3.51573282579364));
#25148=CARTESIAN_POINT('Ctrl Pts',(-52.456091001005,-4.01781939721874,2.84901257911266));
#25149=CARTESIAN_POINT('Ctrl Pts',(-52.4164546680067,-4.49066315447206,
2.18229233243166));
#25150=CARTESIAN_POINT('Ctrl Pts',(-52.3768183350084,-4.79394046776201,
1.39505877874451));
#25151=CARTESIAN_POINT('Ctrl Pts',(-52.3371820020101,-4.89076226499141,
0.583305000514948));
#25152=CARTESIAN_POINT('Ctrl Pts',(-52.3277351766413,-4.91383853217185,
0.389833616929986));
#25153=CARTESIAN_POINT('Ctrl Pts',(-52.3182883512724,-4.92518714038783,
0.194969367527474));
#25154=CARTESIAN_POINT('Ctrl Pts',(-52.3088415259036,-4.92498877504697,
8.594588268108E-5));
#25155=CARTESIAN_POINT('Origin',(-41.25,0.,0.));
#25156=CARTESIAN_POINT('',(-50.5911584740964,-4.92516278400206,-0.000113722891083023));
#25157=CARTESIAN_POINT('',(-50.8088415259036,-4.92521228692415,-0.000105349288354082));
#25158=CARTESIAN_POINT('',(-41.25,-4.925,-6.03138548580071E-16));
#25159=CARTESIAN_POINT('Ctrl Pts',(-50.5911584740964,-4.92516278400206,
-0.000113722891083023));
#25160=CARTESIAN_POINT('Ctrl Pts',(-50.6241609244387,-4.92448960067175,
0.680641940579653));
#25161=CARTESIAN_POINT('Ctrl Pts',(-50.657163374781,-4.78214557076829,1.36167034726095));
#25162=CARTESIAN_POINT('Ctrl Pts',(-50.6901658251233,-4.50788726697863,
1.98462275182099));
#25163=CARTESIAN_POINT('Ctrl Pts',(-50.7298021581216,-4.17849980199303,
2.73279595390601));
#25164=CARTESIAN_POINT('Ctrl Pts',(-50.7694384911199,-3.65883531069533,
3.39719862337027));
#25165=CARTESIAN_POINT('Ctrl Pts',(-50.8090748241183,-3.01203348417392,
3.89710525473833));
#25166=CARTESIAN_POINT('Ctrl Pts',(-50.8487111571166,-2.36523165765252,
4.39701188610637));
#25167=CARTESIAN_POINT('Ctrl Pts',(-50.8883474901149,-1.59129249590741,
4.73242247937822));
#25168=CARTESIAN_POINT('Ctrl Pts',(-50.9279838231132,-0.784250285390256,
4.8625843512811));
#25169=CARTESIAN_POINT('Ctrl Pts',(-50.9676201561115,0.0227919251269108,
4.99274622318398));
#25170=CARTESIAN_POINT('Ctrl Pts',(-51.0072564891099,0.862937184416126,
4.91765937371789));
#25171=CARTESIAN_POINT('Ctrl Pts',(-51.0468928221082,1.63410710728407,4.64644692538026));
#25172=CARTESIAN_POINT('Ctrl Pts',(-51.0865291551065,2.40527703015201,4.37523447704264));
#25173=CARTESIAN_POINT('Ctrl Pts',(-51.1261654881048,3.10747161659867,3.90789642983347));
#25174=CARTESIAN_POINT('Ctrl Pts',(-51.1658018211031,3.65537360881555,3.30121475710258));
#25175=CARTESIAN_POINT('Ctrl Pts',(-51.2054381541015,4.20327560103244,2.69453308437168));
#25176=CARTESIAN_POINT('Ctrl Pts',(-51.2450744870998,4.59688499901954,1.94850778611905));
#25177=CARTESIAN_POINT('Ctrl Pts',(-51.2847108200981,4.78837791632171,1.15378160772726));
#25178=CARTESIAN_POINT('Ctrl Pts',(-51.3243471530964,4.97987083362388,0.359055429335473));
#25179=CARTESIAN_POINT('Ctrl Pts',(-51.3639834860947,4.96924727024111,-0.484371629195479));
#25180=CARTESIAN_POINT('Ctrl Pts',(-51.4036198190931,4.75779799774183,-1.27402247672251));
#25181=CARTESIAN_POINT('Ctrl Pts',(-51.4432561520914,4.54634872524255,-2.06367332424954));
#25182=CARTESIAN_POINT('Ctrl Pts',(-51.4828924850897,4.13407374362675,-2.79954796077265));
#25183=CARTESIAN_POINT('Ctrl Pts',(-51.522528818088,3.57106482584788,-3.39223690197812));
#25184=CARTESIAN_POINT('Ctrl Pts',(-51.5621651510863,3.00805590806901,-3.98492584318359));
#25185=CARTESIAN_POINT('Ctrl Pts',(-51.6018014840847,2.29431305412705,-4.43442908907142));
#25186=CARTESIAN_POINT('Ctrl Pts',(-51.641437817083,1.51655664351954,-4.68613174316612));
#25187=CARTESIAN_POINT('Ctrl Pts',(-51.6810741500813,0.738800232912025,
-4.93783439726082));
#25188=CARTESIAN_POINT('Ctrl Pts',(-51.7207104830797,-0.102969734361041,
-4.99173645956238));
#25189=CARTESIAN_POINT('Ctrl Pts',(-51.760346816078,-0.906477464071566,
-4.84128849925518));
#25190=CARTESIAN_POINT('Ctrl Pts',(-51.7999831490763,-1.70998519378208,
-4.69084053894799));
#25191=CARTESIAN_POINT('Ctrl Pts',(-51.8396194820746,-2.47523068593005,
-4.33604255603204));
#25192=CARTESIAN_POINT('Ctrl Pts',(-51.8792558150729,-3.10923595356447,
-3.82000338107853));
#25193=CARTESIAN_POINT('Ctrl Pts',(-51.9188921480712,-3.74324122119889,
-3.30396420612501));
#25194=CARTESIAN_POINT('Ctrl Pts',(-51.9585284810696,-4.24600626431976,
-2.62668383913391));
#25195=CARTESIAN_POINT('Ctrl Pts',(-51.9981648140679,-4.55644466766691,
-1.87045131141505));
#25196=CARTESIAN_POINT('Ctrl Pts',(-52.0291627007441,-4.79922531155988,
-1.27903408328594));
#25197=CARTESIAN_POINT('Ctrl Pts',(-52.0601605874203,-4.92437633938499,
-0.639328628600892));
#25198=CARTESIAN_POINT('Ctrl Pts',(-52.0911584740964,-4.92503359593706,
0.000126434235863393));
#25199=CARTESIAN_POINT('Ctrl Pts',(-52.3088415259036,-4.92498877504697,
8.594588268108E-5));
#25200=CARTESIAN_POINT('Ctrl Pts',(-52.2786520182741,-4.92435485288396,
-0.622708941807593));
#25201=CARTESIAN_POINT('Ctrl Pts',(-52.2484625106446,-4.8057952323332,-1.24569962972635));
#25202=CARTESIAN_POINT('Ctrl Pts',(-52.2182730030151,-4.57520694571846,
-1.82405286031686));
#25203=CARTESIAN_POINT('Ctrl Pts',(-52.1786366700168,-4.27246354804726,
-2.58338294014709));
#25204=CARTESIAN_POINT('Ctrl Pts',(-52.1390003370185,-3.77661047153599,
-3.26576909703558));
#25205=CARTESIAN_POINT('Ctrl Pts',(-52.0993640040201,-3.14788146612183,
-3.78823038007532));
#25206=CARTESIAN_POINT('Ctrl Pts',(-52.0597276710218,-2.51915246070767,
-4.31069166311506));
#25207=CARTESIAN_POINT('Ctrl Pts',(-52.0200913380235,-1.75754752639063,
-4.67322807230605));
#25208=CARTESIAN_POINT('Ctrl Pts',(-51.9804550050252,-0.955608780981152,
-4.8318262860996));
#25209=CARTESIAN_POINT('Ctrl Pts',(-51.9408186720269,-0.153670035571674,
-4.99042449989316));
#25210=CARTESIAN_POINT('Ctrl Pts',(-51.9011823390286,0.688602520930237,
-4.94508451828928));
#25211=CARTESIAN_POINT('Ctrl Pts',(-51.8615460060302,1.4688752699207,-4.70129756843068));
#25212=CARTESIAN_POINT('Ctrl Pts',(-51.8219096730319,2.24914801891116,-4.45751061857207));
#25213=CARTESIAN_POINT('Ctrl Pts',(-51.7822733400336,2.96742096039018,-4.01527670045875));
#25214=CARTESIAN_POINT('Ctrl Pts',(-51.7426370070353,3.53642168058144,-3.42833645513739));
#25215=CARTESIAN_POINT('Ctrl Pts',(-51.7030006740369,4.10542240077269,-2.84139620981605));
#25216=CARTESIAN_POINT('Ctrl Pts',(-51.6633643410386,4.52515089967618,-2.10974963728667));
#25217=CARTESIAN_POINT('Ctrl Pts',(-51.6237280080403,4.7446106099284,-1.32228800957761));
#25218=CARTESIAN_POINT('Ctrl Pts',(-51.584091675042,4.96407032018062,-0.534826381868543));
#25219=CARTESIAN_POINT('Ctrl Pts',(-51.5444553420437,4.98326124178157,0.30845030102022));
#25220=CARTESIAN_POINT('Ctrl Pts',(-51.5048190090453,4.79985125332747,1.10508096343737));
#25221=CARTESIAN_POINT('Ctrl Pts',(-51.465182676047,4.61644126487337,1.90171162585452));
#25222=CARTESIAN_POINT('Ctrl Pts',(-51.4255463430487,4.23043036636422,2.65169626780005));
#25223=CARTESIAN_POINT('Ctrl Pts',(-51.3859100100504,3.68871942459624,3.26391221075199));
#25224=CARTESIAN_POINT('Ctrl Pts',(-51.3462736770521,3.14700848282826,3.87612815370392));
#25225=CARTESIAN_POINT('Ctrl Pts',(-51.3066373440538,2.44959749780146,4.35057539766226));
#25226=CARTESIAN_POINT('Ctrl Pts',(-51.2670010110554,1.68122241294815,4.6296076288689));
#25227=CARTESIAN_POINT('Ctrl Pts',(-51.2273646780571,0.912847328094825,
4.90863986007553));
#25228=CARTESIAN_POINT('Ctrl Pts',(-51.1877283450588,0.0735081434149867,
4.99225707853046));
#25229=CARTESIAN_POINT('Ctrl Pts',(-51.1480920120605,-0.734814643229353,
4.87029999855603));
#25230=CARTESIAN_POINT('Ctrl Pts',(-51.1084556790621,-1.54313742987369,
4.74834291858159));
#25231=CARTESIAN_POINT('Ctrl Pts',(-51.0688193460638,-2.32044381848253,
4.42081154017779));
#25232=CARTESIAN_POINT('Ctrl Pts',(-51.0291830130655,-2.97229042737678,
3.92750107267045));
#25233=CARTESIAN_POINT('Ctrl Pts',(-50.9895466800672,-3.62413703627103,
3.43419060516311));
#25234=CARTESIAN_POINT('Ctrl Pts',(-50.9499103470689,-4.1505238654507,2.77510104855222));
#25235=CARTESIAN_POINT('Ctrl Pts',(-50.9102740140705,-4.48749444095599,
2.03031243184926));
#25236=CARTESIAN_POINT('Ctrl Pts',(-50.8764631846815,-4.77493916087995,
1.39498824958286));
#25237=CARTESIAN_POINT('Ctrl Pts',(-50.8426523552926,-4.92455445259501,
0.697304833505213));
#25238=CARTESIAN_POINT('Ctrl Pts',(-50.8088415259036,-4.92521228692415,
-0.000105349288354082));
#25239=CARTESIAN_POINT('Origin',(-41.25,0.,0.));
#25240=CARTESIAN_POINT('',(-49.0911584740964,-4.92460059430091,3.93170950760413E-5));
#25241=CARTESIAN_POINT('',(-49.3088415259036,-4.92458892021405,2.43377720096698E-5));
#25242=CARTESIAN_POINT('',(-41.25,-4.925,-6.03138548580071E-16));
#25243=CARTESIAN_POINT('Ctrl Pts',(-49.0911584740964,-4.92460059430091,
3.93170950760413E-5));
#25244=CARTESIAN_POINT('Ctrl Pts',(-49.1088885954605,-4.92470301078537,
0.365886075098635));
#25245=CARTESIAN_POINT('Ctrl Pts',(-49.1266187168247,-4.88447438334452,
0.731710656523951));
#25246=CARTESIAN_POINT('Ctrl Pts',(-49.1443488381888,-4.80367404526498,
1.08834311923078));
#25247=CARTESIAN_POINT('Ctrl Pts',(-49.1839851711871,-4.62304194237499,
1.88560799743165));
#25248=CARTESIAN_POINT('Ctrl Pts',(-49.2236215041854,-4.23964771199399,
2.63693412870344));
#25249=CARTESIAN_POINT('Ctrl Pts',(-49.2632578371838,-3.70007408910792,
3.25103472965791));
#25250=CARTESIAN_POINT('Ctrl Pts',(-49.3028941701821,-3.16050046622184,
3.86513533061238));
#25251=CARTESIAN_POINT('Ctrl Pts',(-49.3425305031804,-2.46474745083068,
4.34201040124952));
#25252=CARTESIAN_POINT('Ctrl Pts',(-49.3821668361787,-1.69734964404053,
4.62371920256889));
#25253=CARTESIAN_POINT('Ctrl Pts',(-49.421803169177,-0.929951837250387,
4.90542800388826));
#25254=CARTESIAN_POINT('Ctrl Pts',(-49.4614395021754,-0.0909092390612466,
4.99197053588986));
#25255=CARTESIAN_POINT('Ctrl Pts',(-49.5010758351737,0.717833739536359,
4.87283180509178));
#25256=CARTESIAN_POINT('Ctrl Pts',(-49.540712168172,1.52657671813397,4.7536930742937));
#25257=CARTESIAN_POINT('Ctrl Pts',(-49.5803485011703,2.30502007714005,4.42887308069593));
#25258=CARTESIAN_POINT('Ctrl Pts',(-49.6199848341686,2.9585822662321,3.93783773818377));
#25259=CARTESIAN_POINT('Ctrl Pts',(-49.659621167167,3.61214445532415,3.44680239567161));
#25260=CARTESIAN_POINT('Ctrl Pts',(-49.6992575001653,4.14082547450218,2.78955170424504));
#25261=CARTESIAN_POINT('Ctrl Pts',(-49.7388938331636,4.48039011661659,2.04594219890398));
#25262=CARTESIAN_POINT('Ctrl Pts',(-49.7785301661619,4.81995475873101,1.30233269356293));
#25263=CARTESIAN_POINT('Ctrl Pts',(-49.8181664991602,4.97040302378181,0.472364374307389));
#25264=CARTESIAN_POINT('Ctrl Pts',(-49.8578028321585,4.91345531571728,-0.343120880710482));
#25265=CARTESIAN_POINT('Ctrl Pts',(-49.8974391651569,4.85650760765276,-1.15860613572836));
#25266=CARTESIAN_POINT('Ctrl Pts',(-49.9370754981552,4.59216392647291,-1.95960832650857));
#25267=CARTESIAN_POINT('Ctrl Pts',(-49.9767118311536,4.1525422611034,-2.64880498490713));
#25268=CARTESIAN_POINT('Ctrl Pts',(-50.0163481641519,3.71292059573389,-3.33800164330569));
#25269=CARTESIAN_POINT('Ctrl Pts',(-50.0559844971501,3.09802094617472,-3.91539276932261));
#25270=CARTESIAN_POINT('Ctrl Pts',(-50.0956208301485,2.38255415872639,-4.31082483512157));
#25271=CARTESIAN_POINT('Ctrl Pts',(-50.1352571631468,1.66708737127806,-4.70625690092052));
#25272=CARTESIAN_POINT('Ctrl Pts',(-50.1748934961451,0.851053445940566,
-4.91972990650151));
#25273=CARTESIAN_POINT('Ctrl Pts',(-50.2145298291434,0.0336012197881862,
-4.92530669464102));
#25274=CARTESIAN_POINT('Ctrl Pts',(-50.2541661621418,-0.7838510063642,-4.93088348278053));
#25275=CARTESIAN_POINT('Ctrl Pts',(-50.2938024951401,-1.60272153333147,
-4.72856405347856));
#25276=CARTESIAN_POINT('Ctrl Pts',(-50.3334388281384,-2.32351687445336,
-4.34293039463065));
#25277=CARTESIAN_POINT('Ctrl Pts',(-50.3730751611367,-3.04431221557524,
-3.95729673578274));
#25278=CARTESIAN_POINT('Ctrl Pts',(-50.4127114941351,-3.66703237085174,
-3.38834884738889));
#25279=CARTESIAN_POINT('Ctrl Pts',(-50.4523478271334,-4.11601629568715,
-2.70521439663872));
#25280=CARTESIAN_POINT('Ctrl Pts',(-50.4919841601317,-4.56500022052256,
-2.02207994588855));
#25281=CARTESIAN_POINT('Ctrl Pts',(-50.53162049313,-4.84024791491689,-1.22475893278206));
#25282=CARTESIAN_POINT('Ctrl Pts',(-50.5712568261283,-4.90831654277731,
-0.410126558875938));
#25283=CARTESIAN_POINT('Ctrl Pts',(-50.5778907087843,-4.91970910247252,
-0.27378257426661));
#25284=CARTESIAN_POINT('Ctrl Pts',(-50.5845245914404,-4.92529810180946,
-0.136953658776159));
#25285=CARTESIAN_POINT('Ctrl Pts',(-50.5911584740964,-4.92516278400206,
-0.000113722891083023));
#25286=CARTESIAN_POINT('Ctrl Pts',(-50.8088415259036,-4.92521228692415,
-0.000105349288354082));
#25287=CARTESIAN_POINT('Ctrl Pts',(-50.8030160222942,-4.92532562978879,
-0.120267013775082));
#25288=CARTESIAN_POINT('Ctrl Pts',(-50.7971905186849,-4.92101698471771,
-0.240420566990935));
#25289=CARTESIAN_POINT('Ctrl Pts',(-50.7913650150756,-4.91222943350402,
-0.36024565322302));
#25290=CARTESIAN_POINT('Ctrl Pts',(-50.7517286820772,-4.85243952871584,
-1.17552744479729));
#25291=CARTESIAN_POINT('Ctrl Pts',(-50.7120923490789,-4.58530539730858,
-1.97560335115078));
#25292=CARTESIAN_POINT('Ctrl Pts',(-50.6724560160806,-4.14328406711282,
-2.66326343083852));
#25293=CARTESIAN_POINT('Ctrl Pts',(-50.6328196830823,-3.70126273691706,
-3.35092351052627));
#25294=CARTESIAN_POINT('Ctrl Pts',(-50.593183350084,-3.08435420793282,-3.92616776354825));
#25295=CARTESIAN_POINT('Ctrl Pts',(-50.5535470170856,-2.36751340869681,
-4.31910351789033));
#25296=CARTESIAN_POINT('Ctrl Pts',(-50.5139106840873,-1.65067260946082,
-4.71203927223239));
#25297=CARTESIAN_POINT('Ctrl Pts',(-50.474274351089,-0.833899539973056,
-4.92266652789455));
#25298=CARTESIAN_POINT('Ctrl Pts',(-50.4346380180907,-0.0164328431554427,
-4.92539388428815));
#25299=CARTESIAN_POINT('Ctrl Pts',(-50.3950016850924,0.801033853662174,
-4.92812124068174));
#25300=CARTESIAN_POINT('Ctrl Pts',(-50.355365352094,1.61919417780964,-4.72294869780679));
#25301=CARTESIAN_POINT('Ctrl Pts',(-50.3157290190957,2.33864093248448,-4.33480490165446));
#25302=CARTESIAN_POINT('Ctrl Pts',(-50.2760926860974,3.05808768715931,-3.94666110550212));
#25303=CARTESIAN_POINT('Ctrl Pts',(-50.2364563530991,3.67882087236151,-3.3755460560724));
#25304=CARTESIAN_POINT('Ctrl Pts',(-50.1968200201008,4.1254208623028,-2.6908507312628));
#25305=CARTESIAN_POINT('Ctrl Pts',(-50.1571836871024,4.57202085224408,-2.00615540645321));
#25306=CARTESIAN_POINT('Ctrl Pts',(-50.1175473541041,4.84448764692445,-1.20787980626376));
#25307=CARTESIAN_POINT('Ctrl Pts',(-50.0779110211058,4.90971629190624,-0.393015116260266));
#25308=CARTESIAN_POINT('Ctrl Pts',(-50.0382746881075,4.97494493688802,0.421849573743228));
#25309=CARTESIAN_POINT('Ctrl Pts',(-49.9986383551092,4.83293543217122,1.25330335356076));
#25310=CARTESIAN_POINT('Ctrl Pts',(-49.9590020221108,4.50094205708306,2.00032386056488));
#25311=CARTESIAN_POINT('Ctrl Pts',(-49.9193656891125,4.1689486819949,2.747344367569));
#25312=CARTESIAN_POINT('Ctrl Pts',(-49.8797293561142,3.64697143653539,3.40993160175972));
#25313=CARTESIAN_POINT('Ctrl Pts',(-49.8400930231159,2.99843101344648,3.90758063337172));
#25314=CARTESIAN_POINT('Ctrl Pts',(-49.8004566901176,2.34989059035758,4.40522966498371));
#25315=CARTESIAN_POINT('Ctrl Pts',(-49.7608203571192,1.57478698963928,4.73794049401699));
#25316=CARTESIAN_POINT('Ctrl Pts',(-49.7211840241209,0.767295978068213,
4.86528846323715));
#25317=CARTESIAN_POINT('Ctrl Pts',(-49.6815476911226,-0.0401950335028599,
4.99263643245731));
#25318=CARTESIAN_POINT('Ctrl Pts',(-49.6419113581243,-0.880073455926696,
4.91462154186436));
#25319=CARTESIAN_POINT('Ctrl Pts',(-49.6022750251259,-1.65029332484226,
4.64072266899981));
#25320=CARTESIAN_POINT('Ctrl Pts',(-49.5626386921276,-2.42051319375783,
4.36682379613526));
#25321=CARTESIAN_POINT('Ctrl Pts',(-49.5230023591293,-3.12107450916513,
3.89704094099911));
#25322=CARTESIAN_POINT('Ctrl Pts',(-49.483366026131,-3.66685845728901,3.28845313221103));
#25323=CARTESIAN_POINT('Ctrl Pts',(-49.4437296931327,-4.21264240541289,
2.67986532342297));
#25324=CARTESIAN_POINT('Ctrl Pts',(-49.4040933601344,-4.60364898625336,
1.93247256098297));
#25325=CARTESIAN_POINT('Ctrl Pts',(-49.364457027136,-4.79237055757407,1.13708372051014));
#25326=CARTESIAN_POINT('Ctrl Pts',(-49.3459185267252,-4.88063843360605,
0.765068571013696));
#25327=CARTESIAN_POINT('Ctrl Pts',(-49.3273800263144,-4.92465501661941,
0.382553936074322));
#25328=CARTESIAN_POINT('Ctrl Pts',(-49.3088415259036,-4.92458892021405,
2.43377720096698E-5));
#25329=CARTESIAN_POINT('Origin',(-41.25,0.,0.));
#25330=CARTESIAN_POINT('',(-47.5911584740964,-4.92537656845547,5.17146674012571E-5));
#25331=CARTESIAN_POINT('',(-47.8088415259036,-4.92534557603861,6.69665181946809E-5));
#25332=CARTESIAN_POINT('',(-41.25,-4.925,-6.03138548580071E-16));
#25333=CARTESIAN_POINT('Ctrl Pts',(-47.5911584740964,-4.92537656845547,
5.17146674012571E-5));
#25334=CARTESIAN_POINT('Ctrl Pts',(-47.5936162664824,-4.92540395716342,
0.0507432792115421));
#25335=CARTESIAN_POINT('Ctrl Pts',(-47.5960740588683,-4.92463762300913,
0.101434014089762));
#25336=CARTESIAN_POINT('Ctrl Pts',(-47.5985318512543,-4.92307227746004,
0.152100063227692));
#25337=CARTESIAN_POINT('Ctrl Pts',(-47.6381681842526,-4.89782825856099,
0.969181443579074));
#25338=CARTESIAN_POINT('Ctrl Pts',(-47.6778045172509,-4.66478233650121,
1.77984271046711));
#25339=CARTESIAN_POINT('Ctrl Pts',(-47.7174408502493,-4.25224979504508,
2.48558780952685));
#25340=CARTESIAN_POINT('Ctrl Pts',(-47.7570771832476,-3.83971725358897,
3.19133290858659));
#25341=CARTESIAN_POINT('Ctrl Pts',(-47.7967135162459,-3.24769809273652,
3.79216183981804));
#25342=CARTESIAN_POINT('Ctrl Pts',(-47.8363498492442,-2.54812315935826,
4.21507336152901));
#25343=CARTESIAN_POINT('Ctrl Pts',(-47.8759861822425,-1.84854822598001,
4.63798488323999));
#25344=CARTESIAN_POINT('Ctrl Pts',(-47.9156225152409,-1.04141752007597,
4.88297899543049));
#25345=CARTESIAN_POINT('Ctrl Pts',(-47.9552588482392,-0.224798129757426,
4.92028869876423));
#25346=CARTESIAN_POINT('Ctrl Pts',(-47.9948951812375,0.591821260561127,
4.95759840209797));
#25347=CARTESIAN_POINT('Ctrl Pts',(-48.0345315142358,1.41792933529417,4.78722369657496));
#25348=CARTESIAN_POINT('Ctrl Pts',(-48.0741678472341,2.15315323938652,4.42986525822725));
#25349=CARTESIAN_POINT('Ctrl Pts',(-48.1138041802324,2.88837714347886,4.07250681987955));
#25350=CARTESIAN_POINT('Ctrl Pts',(-48.1534405132308,3.5327168769305,3.52816464870717));
#25351=CARTESIAN_POINT('Ctrl Pts',(-48.1930768462291,4.00788459744799,2.8629767955519));
#25352=CARTESIAN_POINT('Ctrl Pts',(-48.2327131792274,4.48305231796546,2.19778894239665));
#25353=CARTESIAN_POINT('Ctrl Pts',(-48.2723495122258,4.7890480255488,1.41175540725851));
#25354=CARTESIAN_POINT('Ctrl Pts',(-48.3119858452241,4.8886929735616,0.600379953511863));
#25355=CARTESIAN_POINT('Ctrl Pts',(-48.3516221782224,4.9883379215744,-0.21099550023481));
#25356=CARTESIAN_POINT('Ctrl Pts',(-48.3912585112207,4.88163211001666,-1.04771287259));
#25357=CARTESIAN_POINT('Ctrl Pts',(-48.430894844219,4.58154038850627,-1.80811026953979));
#25358=CARTESIAN_POINT('Ctrl Pts',(-48.4705311772173,4.28144866699588,-2.56850766648958));
#25359=CARTESIAN_POINT('Ctrl Pts',(-48.5101675102157,3.78797103553283,-3.25258508803395));
#25360=CARTESIAN_POINT('Ctrl Pts',(-48.549803843214,3.16106545880817,-3.77722652795134));
#25361=CARTESIAN_POINT('Ctrl Pts',(-48.5894401762123,2.5341598820835,-4.30186796786874));
#25362=CARTESIAN_POINT('Ctrl Pts',(-48.6290765092106,1.77382636009721,-4.66707342615914));
#25363=CARTESIAN_POINT('Ctrl Pts',(-48.6687128422089,0.972446082103007,
-4.8284701195857));
#25364=CARTESIAN_POINT('Ctrl Pts',(-48.7083491752073,0.171065804108807,
-4.98986681301226));
#25365=CARTESIAN_POINT('Ctrl Pts',(-48.7479855082056,-0.671361229893299,
-4.94745474157497));
#25366=CARTESIAN_POINT('Ctrl Pts',(-48.7876218412039,-1.4524793969955,-4.70638700912207));
#25367=CARTESIAN_POINT('Ctrl Pts',(-48.8272581742023,-2.2335975640977,-4.46531927666918));
#25368=CARTESIAN_POINT('Ctrl Pts',(-48.8668945072005,-2.9534068643,-4.02559588320067));
#25369=CARTESIAN_POINT('Ctrl Pts',(-48.9065308401989,-3.52444983680959,
-3.44064360638272));
#25370=CARTESIAN_POINT('Ctrl Pts',(-48.9461671731972,-4.09549280931918,
-2.85569132956477));
#25371=CARTESIAN_POINT('Ctrl Pts',(-48.9858035061955,-4.51776945413606,
-2.12551016939737));
#25372=CARTESIAN_POINT('Ctrl Pts',(-49.0254398391939,-4.73997278884501,
-1.3388177767487));
#25373=CARTESIAN_POINT('Ctrl Pts',(-49.0473460508281,-4.86278014532179,
-0.904028563399918));
#25374=CARTESIAN_POINT('Ctrl Pts',(-49.0692522624622,-4.92447405499882,
-0.451977696320464));
#25375=CARTESIAN_POINT('Ctrl Pts',(-49.0911584740964,-4.92460059430091,
3.93170950760413E-5));
#25376=CARTESIAN_POINT('Ctrl Pts',(-49.3088415259036,-4.92458892021405,
2.43377720096698E-5));
#25377=CARTESIAN_POINT('Ctrl Pts',(-49.2877436933161,-4.92451369887121,
-0.435315373957988));
#25378=CARTESIAN_POINT('Ctrl Pts',(-49.2666458607286,-4.86734395233281,
-0.870674465773623));
#25379=CARTESIAN_POINT('Ctrl Pts',(-49.2455480281411,-4.75332821260385,
-1.29059902828803));
#25380=CARTESIAN_POINT('Ctrl Pts',(-49.2059116951427,-4.53912773451197,
-2.07950801810765));
#25381=CARTESIAN_POINT('Ctrl Pts',(-49.1662753621445,-4.12429021652726,
-2.81394107924121));
#25382=CARTESIAN_POINT('Ctrl Pts',(-49.1266390291461,-3.55921878063583,
-3.40466395112918));
#25383=CARTESIAN_POINT('Ctrl Pts',(-49.0870026961478,-2.9941473447444,-3.99538682301714));
#25384=CARTESIAN_POINT('Ctrl Pts',(-49.0473663631495,-2.27884199094625,
-4.44239950565951));
#25385=CARTESIAN_POINT('Ctrl Pts',(-49.0077300301511,-1.50021294659875,
-4.69138956636627));
#25386=CARTESIAN_POINT('Ctrl Pts',(-48.9680936971528,-0.721583902251253,
-4.94037962707302));
#25387=CARTESIAN_POINT('Ctrl Pts',(-48.9284573641545,0.120368832645595,
-4.99134706584417));
#25388=CARTESIAN_POINT('Ctrl Pts',(-48.8888210311562,0.923347262940818,
-4.8380992942033));
#25389=CARTESIAN_POINT('Ctrl Pts',(-48.8491846981579,1.72632569323603,-4.68485152256244));
#25390=CARTESIAN_POINT('Ctrl Pts',(-48.8095483651595,2.49032981892962,-4.32738854050958));
#25391=CARTESIAN_POINT('Ctrl Pts',(-48.7699120321612,3.1225324692007,-3.80914241363316));
#25392=CARTESIAN_POINT('Ctrl Pts',(-48.7302756991629,3.75473511947177,-3.29089628675674));
#25393=CARTESIAN_POINT('Ctrl Pts',(-48.6906393661646,4.25513629432032,-2.61186701505678));
#25394=CARTESIAN_POINT('Ctrl Pts',(-48.6510030331663,4.56293681246637,-1.85455725012484));
#25395=CARTESIAN_POINT('Ctrl Pts',(-48.611366700168,4.87073733061243,-1.0972474851929));
#25396=CARTESIAN_POINT('Ctrl Pts',(-48.5717303671696,4.98593719205599,-0.261657227028983));
#25397=CARTESIAN_POINT('Ctrl Pts',(-48.5320940341713,4.89453951267414,0.550688575715041));
#25398=CARTESIAN_POINT('Ctrl Pts',(-48.492457701173,4.80314183329228,1.36303437845905));
#25399=CARTESIAN_POINT('Ctrl Pts',(-48.4528213681747,4.50514661308501,2.15213572578318));
#25400=CARTESIAN_POINT('Ctrl Pts',(-48.4131850351763,4.03676053246116,2.82211611244389));
#25401=CARTESIAN_POINT('Ctrl Pts',(-48.373548702178,3.5683744518373,3.4920964991046));
#25402=CARTESIAN_POINT('Ctrl Pts',(-48.3339123691797,2.92959751079684,4.04295592510191));
#25403=CARTESIAN_POINT('Ctrl Pts',(-48.2942760361814,2.19804166748022,4.40776448742128));
#25404=CARTESIAN_POINT('Ctrl Pts',(-48.2546397031831,1.4664858241636,4.77257304974066));
#25405=CARTESIAN_POINT('Ctrl Pts',(-48.2150033701847,0.642151078570819,
4.9513307483821));
#25406=CARTESIAN_POINT('Ctrl Pts',(-48.1753670371864,-0.174805175287565,
4.92231836630303));
#25407=CARTESIAN_POINT('Ctrl Pts',(-48.1357307041881,-0.99176142914595,
4.89330598422397));
#25408=CARTESIAN_POINT('Ctrl Pts',(-48.0960943711898,-1.80133919126995,
4.65652352142439));
#25409=CARTESIAN_POINT('Ctrl Pts',(-48.0564580381915,-2.50517405407298,
4.24074025464317));
#25410=CARTESIAN_POINT('Ctrl Pts',(-48.0168217051931,-3.20900891687601,
3.82495698786194));
#25411=CARTESIAN_POINT('Ctrl Pts',(-47.9771853721948,-3.80710088035809,
3.23017291709908));
#25412=CARTESIAN_POINT('Ctrl Pts',(-47.9375490391965,-4.22678124680716,
2.52865482820229));
#25413=CARTESIAN_POINT('Ctrl Pts',(-47.8979127061982,-4.64646161325623,
1.82713673930551));
#25414=CARTESIAN_POINT('Ctrl Pts',(-47.8582763731999,-4.88773038267229,
1.01888463227482));
#25415=CARTESIAN_POINT('Ctrl Pts',(-47.8186400402016,-4.92127318813094,
0.202101846441171));
#25416=CARTESIAN_POINT('Ctrl Pts',(-47.8153738687689,-4.92403723174125,
0.134796109508387));
#25417=CARTESIAN_POINT('Ctrl Pts',(-47.8121076973363,-4.92539074707072,
0.067432446433504));
#25418=CARTESIAN_POINT('Ctrl Pts',(-47.8088415259036,-4.92534557603861,
6.69665181946809E-5));
#25419=CARTESIAN_POINT('Origin',(-41.25,0.,0.));
#25420=CARTESIAN_POINT('',(-46.0911584740964,-4.92478006052077,-0.000110922936781277));
#25421=CARTESIAN_POINT('',(-46.3088415259036,-4.92482432270619,-0.000117749303604396));
#25422=CARTESIAN_POINT('',(-41.25,-4.925,-6.03138548580071E-16));
#25423=CARTESIAN_POINT('Ctrl Pts',(-46.0911584740964,-4.92478006052077,
-0.000110922936781277));
#25424=CARTESIAN_POINT('Ctrl Pts',(-46.1179802705025,-4.92432113727213,
0.553277446459616));
#25425=CARTESIAN_POINT('Ctrl Pts',(-46.1448020669086,-4.83122565564324,
1.10681635025798));
#25426=CARTESIAN_POINT('Ctrl Pts',(-46.1716238633147,-4.64828498189497,
1.62887132868731));
#25427=CARTESIAN_POINT('Ctrl Pts',(-46.2112601963131,-4.37794151370094,
2.4003463132539));
#25428=CARTESIAN_POINT('Ctrl Pts',(-46.2508965293114,-3.91139485952201,
3.10306696251328));
#25429=CARTESIAN_POINT('Ctrl Pts',(-46.2905328623097,-3.30533084670784,
3.65165210173844));
#25430=CARTESIAN_POINT('Ctrl Pts',(-46.330169195308,-2.69926683389369,4.20023724096358));
#25431=CARTESIAN_POINT('Ctrl Pts',(-46.3698055283064,-1.95368546244432,
4.59468687015451));
#25432=CARTESIAN_POINT('Ctrl Pts',(-46.4094418613047,-1.15917552239483,
4.78707501368114));
#25433=CARTESIAN_POINT('Ctrl Pts',(-46.449078194303,-0.364665582345333,
4.97946315720777));
#25434=CARTESIAN_POINT('Ctrl Pts',(-46.4887145273013,0.478772926304282,
4.96978981507011));
#25435=CARTESIAN_POINT('Ctrl Pts',(-46.5283508602996,1.26866148559008,4.75923030681535));
#25436=CARTESIAN_POINT('Ctrl Pts',(-46.567987193298,2.05855004487589,4.54867079856059));
#25437=CARTESIAN_POINT('Ctrl Pts',(-46.6076235262963,2.79488865479788,4.13722512418875));
#25438=CARTESIAN_POINT('Ctrl Pts',(-46.6472598592946,3.38821152894656,3.57488429371401));
#25439=CARTESIAN_POINT('Ctrl Pts',(-46.6868961922929,3.98153440309523,3.01254346323927));
#25440=CARTESIAN_POINT('Ctrl Pts',(-46.7265325252913,4.4318415414706,2.29930747666162));
#25441=CARTESIAN_POINT('Ctrl Pts',(-46.7661688582896,4.68442023212502,1.52183513140787));
#25442=CARTESIAN_POINT('Ctrl Pts',(-46.8058051912879,4.93699892277945,0.744362786154099));
#25443=CARTESIAN_POINT('Ctrl Pts',(-46.8454415242862,4.99184916571294,-0.097345917775786));
#25444=CARTESIAN_POINT('Ctrl Pts',(-46.8850778572845,4.84230660834004,-0.901022635207284));
#25445=CARTESIAN_POINT('Ctrl Pts',(-46.9247141902828,4.69276405096713,-1.70469935263878));
#25446=CARTESIAN_POINT('Ctrl Pts',(-46.9643505232812,4.33882869328785,-2.47034408357189));
#25447=CARTESIAN_POINT('Ctrl Pts',(-47.0039868562795,3.82350399143802,-3.10493032221128));
#25448=CARTESIAN_POINT('Ctrl Pts',(-47.0436231892778,3.3081792895882,-3.73951656085065));
#25449=CARTESIAN_POINT('Ctrl Pts',(-47.0832595222761,2.63146524356784,-4.24304430719631));
#25450=CARTESIAN_POINT('Ctrl Pts',(-47.1228958552744,1.87558320301932,-4.55433449879137));
#25451=CARTESIAN_POINT('Ctrl Pts',(-47.1625321882727,1.11970116247081,-4.86562469038643));
#25452=CARTESIAN_POINT('Ctrl Pts',(-47.2021685212711,0.284651127394135,
-4.9846773272309));
#25453=CARTESIAN_POINT('Ctrl Pts',(-47.2418048542694,-0.5281075911373,-4.89702740961419));
#25454=CARTESIAN_POINT('Ctrl Pts',(-47.2814411872678,-1.34086630966875,
-4.80937749199747));
#25455=CARTESIAN_POINT('Ctrl Pts',(-47.3210775202661,-2.13133371165496,
-4.51502501991956));
#25456=CARTESIAN_POINT('Ctrl Pts',(-47.3607138532644,-2.80346731501383,
-4.04973407669918));
#25457=CARTESIAN_POINT('Ctrl Pts',(-47.4003501862627,-3.4756009183727,-3.58444313347881));
#25458=CARTESIAN_POINT('Ctrl Pts',(-47.439986519261,-4.02940072310423,-2.94821371911597));
#25459=CARTESIAN_POINT('Ctrl Pts',(-47.4796228522593,-4.39757956760083,
-2.21834826502719));
#25460=CARTESIAN_POINT('Ctrl Pts',(-47.5168013928717,-4.74292816791932,
-1.53374072508281));
#25461=CARTESIAN_POINT('Ctrl Pts',(-47.553979933484,-4.92496226487288,-0.766749583062766));
#25462=CARTESIAN_POINT('Ctrl Pts',(-47.5911584740964,-4.92537656845547,
5.17146674012571E-5));
#25463=CARTESIAN_POINT('Ctrl Pts',(-47.8088415259036,-4.92534557603861,
6.69665181946809E-5));
#25464=CARTESIAN_POINT('Ctrl Pts',(-47.7724713643379,-4.92484257802704,
-0.750075345052349));
#25465=CARTESIAN_POINT('Ctrl Pts',(-47.7361012027722,-4.75090613579548,
-1.50044294007547));
#25466=CARTESIAN_POINT('Ctrl Pts',(-47.6997310412066,-4.41988711904088,
-2.17356223823657));
#25467=CARTESIAN_POINT('Ctrl Pts',(-47.6600947082082,-4.05914140299093,
-2.90713007244404));
#25468=CARTESIAN_POINT('Ctrl Pts',(-47.6204583752099,-3.51183312938981,
-3.54895227622236));
#25469=CARTESIAN_POINT('Ctrl Pts',(-47.5808220422116,-2.8444607331238,-4.02104688933967));
#25470=CARTESIAN_POINT('Ctrl Pts',(-47.5411857092133,-2.17708833685779,
-4.49314150245699));
#25471=CARTESIAN_POINT('Ctrl Pts',(-47.501549376215,-1.3896518179269,-4.7955085249133));
#25472=CARTESIAN_POINT('Ctrl Pts',(-47.4619130432167,-0.577825403465827,
-4.89141009849522));
#25473=CARTESIAN_POINT('Ctrl Pts',(-47.4222767102183,0.234001010995242,
-4.98731167207714));
#25474=CARTESIAN_POINT('Ctrl Pts',(-47.38264037722,1.07021732098649,-4.87674779678467));
#25475=CARTESIAN_POINT('Ctrl Pts',(-47.3430040442217,1.82922251201032,-4.57315208036056));
#25476=CARTESIAN_POINT('Ctrl Pts',(-47.3033677112234,2.58822770303417,-4.26955636393644));
#25477=CARTESIAN_POINT('Ctrl Pts',(-47.2637313782251,3.27002177509061,-3.77292880638065));
#25478=CARTESIAN_POINT('Ctrl Pts',(-47.2240950452267,3.79176615092188,-3.14361009116501));
#25479=CARTESIAN_POINT('Ctrl Pts',(-47.1844587122284,4.31351052675315,-2.51429137594937));
#25480=CARTESIAN_POINT('Ctrl Pts',(-47.1448223792301,4.67520520635928,-1.75228150307386));
#25481=CARTESIAN_POINT('Ctrl Pts',(-47.1051860462318,4.83290396919025,-0.950165339894358));
#25482=CARTESIAN_POINT('Ctrl Pts',(-47.0655497132334,4.99060273202123,-0.148049176714858));
#25483=CARTESIAN_POINT('Ctrl Pts',(-47.0259133802351,4.94430557807706,0.694173276768634));
#25484=CARTESIAN_POINT('Ctrl Pts',(-46.9862770472368,4.69963765213535,1.47417125436063));
#25485=CARTESIAN_POINT('Ctrl Pts',(-46.9466407142385,4.45496972619363,2.25416923195263));
#25486=CARTESIAN_POINT('Ctrl Pts',(-46.9070043812402,4.01193102825436,2.97194273365312));
#25487=CARTESIAN_POINT('Ctrl Pts',(-46.8673680482418,3.42435114838233,3.54028164997137));
#25488=CARTESIAN_POINT('Ctrl Pts',(-46.8277317152435,2.83677126851031,4.10862056628962));
#25489=CARTESIAN_POINT('Ctrl Pts',(-46.7880953822452,2.10465020670554,4.52752489722563));
#25490=CARTESIAN_POINT('Ctrl Pts',(-46.7484590492469,1.31694131358517,4.74609739945611));
#25491=CARTESIAN_POINT('Ctrl Pts',(-46.7088227162486,0.529232420464796,
4.96466990168658));
#25492=CARTESIAN_POINT('Ctrl Pts',(-46.6691863832503,-0.314064303971186,
4.98291057521152));
#25493=CARTESIAN_POINT('Ctrl Pts',(-46.6295500502519,-1.11048756866507,
4.79860316221208));
#25494=CARTESIAN_POINT('Ctrl Pts',(-46.5899137172536,-1.90691083335896,
4.61429574921265));
#25495=CARTESIAN_POINT('Ctrl Pts',(-46.5502773842553,-2.65646063831076,
4.22744024968884));
#25496=CARTESIAN_POINT('Ctrl Pts',(-46.5106410512569,-3.26806602533696,
3.6850399458608));
#25497=CARTESIAN_POINT('Ctrl Pts',(-46.4710047182586,-3.87967141236316,
3.14263964203275));
#25498=CARTESIAN_POINT('Ctrl Pts',(-46.4313683852603,-4.35333238146376,
2.44469453390046));
#25499=CARTESIAN_POINT('Ctrl Pts',(-46.391732052262,-4.63149870979145,1.67600556375914));
#25500=CARTESIAN_POINT('Ctrl Pts',(-46.3641018768092,-4.82540626569679,
1.14015853889599));
#25501=CARTESIAN_POINT('Ctrl Pts',(-46.3364717013564,-4.92431565913374,
0.569934423846609));
#25502=CARTESIAN_POINT('Ctrl Pts',(-46.3088415259036,-4.92482432270619,
-0.000117749303604396));
#25503=CARTESIAN_POINT('Origin',(-41.25,0.,0.));
#25504=CARTESIAN_POINT('',(-44.5911584740964,-4.92485068894608,0.000120817416453672));
#25505=CARTESIAN_POINT('',(-44.8088415259036,-4.9248046659208,0.000114993715491958));
#25506=CARTESIAN_POINT('',(-41.25,-4.925,-6.03138548580071E-16));
#25507=CARTESIAN_POINT('Ctrl Pts',(-44.5911584740964,-4.92485068894608,
0.000120817416453672));
#25508=CARTESIAN_POINT('Ctrl Pts',(-44.6027079415244,-4.92507068379112,
0.238400082149576));
#25509=CARTESIAN_POINT('Ctrl Pts',(-44.6142574089523,-4.90808726014739,
0.476648255516139));
#25510=CARTESIAN_POINT('Ctrl Pts',(-44.6258068763803,-4.87363743235764,
0.712343494047093));
#25511=CARTESIAN_POINT('Ctrl Pts',(-44.6654432093786,-4.75540991628145,
1.52122018198193));
#25512=CARTESIAN_POINT('Ctrl Pts',(-44.7050795423769,-4.43146713264999,
2.30002899398948));
#25513=CARTESIAN_POINT('Ctrl Pts',(-44.7447158753752,-3.94116841268779,
2.95414397473762));
#25514=CARTESIAN_POINT('Ctrl Pts',(-44.7843522083736,-3.4508696927256,3.60825895548577));
#25515=CARTESIAN_POINT('Ctrl Pts',(-44.8239885413719,-2.79421503643267,
4.13768010497451));
#25516=CARTESIAN_POINT('Ctrl Pts',(-44.8636248743702,-2.05098856046108,
4.47808229065024));
#25517=CARTESIAN_POINT('Ctrl Pts',(-44.9032612073685,-1.3077620844895,4.81848447632595));
#25518=CARTESIAN_POINT('Ctrl Pts',(-44.9428975403668,-0.47796378883926,
4.96986769818865));
#25519=CARTESIAN_POINT('Ctrl Pts',(-44.9825338733652,0.33758510658002,4.91383876157463));
#25520=CARTESIAN_POINT('Ctrl Pts',(-45.0221702063635,1.1531340019993,4.85780982496061));
#25521=CARTESIAN_POINT('Ctrl Pts',(-45.0618065393618,1.95443349718762,4.59436872986986));
#25522=CARTESIAN_POINT('Ctrl Pts',(-45.1014428723601,2.64412500113517,4.15552380049798));
#25523=CARTESIAN_POINT('Ctrl Pts',(-45.1410792053584,3.33381650508272,3.71667887112609));
#25524=CARTESIAN_POINT('Ctrl Pts',(-45.1807155383567,3.9119000177895,3.10243010747307));
#25525=CARTESIAN_POINT('Ctrl Pts',(-45.2203518713551,4.30813788590293,2.38740927249545));
#25526=CARTESIAN_POINT('Ctrl Pts',(-45.2599882043534,4.70437575401636,1.67238843751783));
#25527=CARTESIAN_POINT('Ctrl Pts',(-45.2996245373517,4.91876797753645,0.856595531215603));
#25528=CARTESIAN_POINT('Ctrl Pts',(-45.33926087035,4.9252657133911,0.039150106707696));
#25529=CARTESIAN_POINT('Ctrl Pts',(-45.3788972033484,4.93176344924574,-0.778295317800222));
#25530=CARTESIAN_POINT('Ctrl Pts',(-45.4185335363467,4.73036669743492,-1.59739326051383));
#25531=CARTESIAN_POINT('Ctrl Pts',(-45.458169869345,4.34554533981538,-2.31862260359579));
#25532=CARTESIAN_POINT('Ctrl Pts',(-45.4978062023433,3.96072398219585,-3.03985194667775));
#25533=CARTESIAN_POINT('Ctrl Pts',(-45.5374425353416,3.39247801876759,-3.66321269012808));
#25534=CARTESIAN_POINT('Ctrl Pts',(-45.57707886834,2.70984983207305,-4.11296595730674));
#25535=CARTESIAN_POINT('Ctrl Pts',(-45.6167152013383,2.02722164537851,-4.5627192244854));
#25536=CARTESIAN_POINT('Ctrl Pts',(-45.6563515343366,1.23021123541768,-4.8388650153924));
#25537=CARTESIAN_POINT('Ctrl Pts',(-45.6959878673349,0.415656065479166,
-4.90785137443562));
#25538=CARTESIAN_POINT('Ctrl Pts',(-45.7356242003332,-0.398899104459364,
-4.97683773347883));
#25539=CARTESIAN_POINT('Ctrl Pts',(-45.7752605333315,-1.23099903437559,
-4.83866466065824));
#25540=CARTESIAN_POINT('Ctrl Pts',(-45.8148968663299,-1.97954285356023,
-4.51012030540781));
#25541=CARTESIAN_POINT('Ctrl Pts',(-45.8545331993282,-2.72808667274487,
-4.18157595015737));
#25542=CARTESIAN_POINT('Ctrl Pts',(-45.8941695323265,-3.39307438119792,
-3.6626603124771));
#25543=CARTESIAN_POINT('Ctrl Pts',(-45.9338058653248,-3.89370938956717,
-3.01642209710863));
#25544=CARTESIAN_POINT('Ctrl Pts',(-45.9734421983232,-4.39434439793641,
-2.37018388174015));
#25545=CARTESIAN_POINT('Ctrl Pts',(-46.0130785313215,-4.73062670622184,
-1.59662308868348));
#25546=CARTESIAN_POINT('Ctrl Pts',(-46.0527148643198,-4.86169771925999,
-0.789728032218253));
#25547=CARTESIAN_POINT('Ctrl Pts',(-46.065529400912,-4.90407334197024,-0.528856618417667));
#25548=CARTESIAN_POINT('Ctrl Pts',(-46.0783439375042,-4.92499931834652,
-0.264500951179397));
#25549=CARTESIAN_POINT('Ctrl Pts',(-46.0911584740964,-4.92478006052077,
-0.000110922936781277));
#25550=CARTESIAN_POINT('Ctrl Pts',(-46.3088415259036,-4.92482432270619,
-0.000117749303604396));
#25551=CARTESIAN_POINT('Ctrl Pts',(-46.2968353683581,-4.92504535260877,
-0.247822879214976));
#25552=CARTESIAN_POINT('Ctrl Pts',(-46.2848292108125,-4.90668666485232,
-0.495495543595402));
#25553=CARTESIAN_POINT('Ctrl Pts',(-46.272823053267,-4.86946908996704,-0.740301107933112));
#25554=CARTESIAN_POINT('Ctrl Pts',(-46.2331867202687,-4.74660145426015,
-1.54848597733368));
#25555=CARTESIAN_POINT('Ctrl Pts',(-46.1935503872704,-4.41819449529159,
-2.32542288398449));
#25556=CARTESIAN_POINT('Ctrl Pts',(-46.1539140542721,-3.92414994638157,
-2.97671331284438));
#25557=CARTESIAN_POINT('Ctrl Pts',(-46.1142777212738,-3.43010539747155,
-3.62800374170428));
#25558=CARTESIAN_POINT('Ctrl Pts',(-46.0746413882754,-2.77042325862007,
-4.15364769277325));
#25559=CARTESIAN_POINT('Ctrl Pts',(-46.0350050552771,-2.02525548782224,
-4.48977896533864));
#25560=CARTESIAN_POINT('Ctrl Pts',(-45.9953687222788,-1.28008771702442,
-4.82591023790403));
#25561=CARTESIAN_POINT('Ctrl Pts',(-45.9557323892805,-0.449434314280258,
-4.97252883196583));
#25562=CARTESIAN_POINT('Ctrl Pts',(-45.9160960562821,0.365779604018302,
-4.91182045985354));
#25563=CARTESIAN_POINT('Ctrl Pts',(-45.8764597232838,1.18099352231686,-4.85111208774125));
#25564=CARTESIAN_POINT('Ctrl Pts',(-45.8368233902855,1.98076795616981,-4.58307674945487));
#25565=CARTESIAN_POINT('Ctrl Pts',(-45.7971870572872,2.6679296109669,-4.14028097349408));
#25566=CARTESIAN_POINT('Ctrl Pts',(-45.7575507242889,3.35509126576401,-3.69748519753329));
#25567=CARTESIAN_POINT('Ctrl Pts',(-45.7179143912905,3.92964014150524,-3.07992898389807));
#25568=CARTESIAN_POINT('Ctrl Pts',(-45.6782780582922,4.32176804627143,-2.36264595375167));
#25569=CARTESIAN_POINT('Ctrl Pts',(-45.6386417252939,4.71389595103761,-1.64536292360528));
#25570=CARTESIAN_POINT('Ctrl Pts',(-45.5990053922956,4.92360288482874,-0.828353076947685));
#25571=CARTESIAN_POINT('Ctrl Pts',(-45.5593690592973,4.92540927140877,-0.0108838261501201));
#25572=CARTESIAN_POINT('Ctrl Pts',(-45.519732726299,4.9272156579888,0.806585424647439));
#25573=CARTESIAN_POINT('Ctrl Pts',(-45.4800963933006,4.72112149735772,1.62451407958498));
#25574=CARTESIAN_POINT('Ctrl Pts',(-45.4404600603023,4.3321674106464,2.34352309028179));
#25575=CARTESIAN_POINT('Ctrl Pts',(-45.4008237273039,3.94321332393509,3.06253210097861));
#25576=CARTESIAN_POINT('Ctrl Pts',(-45.3611873943057,3.37139931114353,3.6826214674347));
#25577=CARTESIAN_POINT('Ctrl Pts',(-45.3215510613074,2.68620127594623,4.12844978819655));
#25578=CARTESIAN_POINT('Ctrl Pts',(-45.281914728309,2.00100324074892,4.5742781089584));
#25579=CARTESIAN_POINT('Ctrl Pts',(-45.2422783953107,1.20242118314586,4.84584538402601));
#25580=CARTESIAN_POINT('Ctrl Pts',(-45.2026420623123,0.387483522987002,
4.9101559514902));
#25581=CARTESIAN_POINT('Ctrl Pts',(-45.163005729314,-0.427454137171852,
4.9744665189544));
#25582=CARTESIAN_POINT('Ctrl Pts',(-45.1233693963158,-1.25874739988651,
4.83152037881518));
#25583=CARTESIAN_POINT('Ctrl Pts',(-45.0837330633174,-2.00539340521582,
4.49868561236386));
#25584=CARTESIAN_POINT('Ctrl Pts',(-45.0440967303191,-2.75203941054511,
4.16585084591255));
#25585=CARTESIAN_POINT('Ctrl Pts',(-45.0044603973208,-3.41403815848903,
3.64312745314915));
#25586=CARTESIAN_POINT('Ctrl Pts',(-44.9648240643225,-3.91095622102169,
2.9940267844109));
#25587=CARTESIAN_POINT('Ctrl Pts',(-44.9251877313241,-4.40787428355437,
2.34492611567263));
#25588=CARTESIAN_POINT('Ctrl Pts',(-44.8855513983258,-4.73971166067577,
1.5694481709595));
#25589=CARTESIAN_POINT('Ctrl Pts',(-44.8459150653275,-4.8661498202455,0.761814200122423));
#25590=CARTESIAN_POINT('Ctrl Pts',(-44.8335572188529,-4.90557080716081,
0.510009457748148));
#25591=CARTESIAN_POINT('Ctrl Pts',(-44.8211993723782,-4.92502550111584,
0.255078916523799));
#25592=CARTESIAN_POINT('Ctrl Pts',(-44.8088415259036,-4.9248046659208,0.000114993715491958));
#25593=CARTESIAN_POINT('Origin',(-41.25,0.,0.));
#25594=CARTESIAN_POINT('',(-43.0911584740964,-4.92532729948334,-7.01527563526372E-5));
#25595=CARTESIAN_POINT('',(-43.3088415259036,-4.92535985208058,-6.05620874156806E-5));
#25596=CARTESIAN_POINT('',(-41.25,-4.925,-6.03138548580071E-16));
#25597=CARTESIAN_POINT('Ctrl Pts',(-43.0911584740964,-4.92532729948334,
-7.01527563526372E-5));
#25598=CARTESIAN_POINT('Ctrl Pts',(-43.1270719455445,-4.92478402712806,
0.740663394333482));
#25599=CARTESIAN_POINT('Ctrl Pts',(-43.1629854169926,-4.75533079067205,
1.48162892060557));
#25600=CARTESIAN_POINT('Ctrl Pts',(-43.1988988884407,-4.43228738909528,
2.14815911814967));
#25601=CARTESIAN_POINT('Ctrl Pts',(-43.2385352214391,-4.07575666896397,
2.8837831555383));
#25602=CARTESIAN_POINT('Ctrl Pts',(-43.2781715544374,-3.53214241241189,
3.52873976951395));
#25603=CARTESIAN_POINT('Ctrl Pts',(-43.3178078874357,-2.8674907220931,4.00465760137893));
#25604=CARTESIAN_POINT('Ctrl Pts',(-43.357444220434,-2.20283903177432,4.4805754332439));
#25605=CARTESIAN_POINT('Ctrl Pts',(-43.3970805534323,-1.41714990768884,
4.7874544829982));
#25606=CARTESIAN_POINT('Ctrl Pts',(-43.4367168864307,-0.605887023971831,
4.88801296947649));
#25607=CARTESIAN_POINT('Ctrl Pts',(-43.476353219429,0.20537585974518,4.98857145595478));
#25608=CARTESIAN_POINT('Ctrl Pts',(-43.5159895524273,1.04221250309372,4.88280937915706));
#25609=CARTESIAN_POINT('Ctrl Pts',(-43.5556258854256,1.80294740105899,4.58357477299046));
#25610=CARTESIAN_POINT('Ctrl Pts',(-43.5952622184239,2.56368229902428,4.28434016682385));
#25611=CARTESIAN_POINT('Ctrl Pts',(-43.6348985514223,3.24831545160629,3.79163303128835));
#25612=CARTESIAN_POINT('Ctrl Pts',(-43.6745348844206,3.77366288949504,3.16531879318089));
#25613=CARTESIAN_POINT('Ctrl Pts',(-43.7141712174189,4.29901032738379,2.53900455507344));
#25614=CARTESIAN_POINT('Ctrl Pts',(-43.7538075504172,4.66507205057929,1.77908321439402));
#25615=CARTESIAN_POINT('Ctrl Pts',(-43.7934438834155,4.82737146005745,0.977885339744746));
#25616=CARTESIAN_POINT('Ctrl Pts',(-43.8330802164138,4.98967086953561,0.176687465095475));
#25617=CARTESIAN_POINT('Ctrl Pts',(-43.8727165494122,4.94820796529643,-0.665786943523648));
#25618=CARTESIAN_POINT('Ctrl Pts',(-43.9123528824105,4.7080204157121,-1.44717623639338));
#25619=CARTESIAN_POINT('Ctrl Pts',(-43.9519892154088,4.46783286612776,-2.22856552926312));
#25620=CARTESIAN_POINT('Ctrl Pts',(-43.9916255484071,4.02892067119828,-2.94886970638347));
#25621=CARTESIAN_POINT('Ctrl Pts',(-44.0312618814055,3.44461210279907,-3.52057131467165));
#25622=CARTESIAN_POINT('Ctrl Pts',(-44.0708982144038,2.86030353439988,-4.09227292295982));
#25623=CARTESIAN_POINT('Ctrl Pts',(-44.1105345474021,2.13059859253097,-4.51537196241583));
#25624=CARTESIAN_POINT('Ctrl Pts',(-44.1501708804004,1.34415703928449,-4.73846146095394));
#25625=CARTESIAN_POINT('Ctrl Pts',(-44.1898072133987,0.557715486037999,
-4.96155095949204));
#25626=CARTESIAN_POINT('Ctrl Pts',(-44.2294435463971,-0.285462678586069,
-4.98463091711224));
#25627=CARTESIAN_POINT('Ctrl Pts',(-44.2690798793954,-1.08293055470127,
-4.80489713281615));
#25628=CARTESIAN_POINT('Ctrl Pts',(-44.3087162123937,-1.88039843081648,
-4.62516334852005));
#25629=CARTESIAN_POINT('Ctrl Pts',(-44.348352545392,-2.63215601842282,-4.24261582230765));
#25630=CARTESIAN_POINT('Ctrl Pts',(-44.3879888783903,-3.24686411880041,
-3.70373439678756));
#25631=CARTESIAN_POINT('Ctrl Pts',(-44.4276252113887,-3.86157221917799,
-3.16485297126747));
#25632=CARTESIAN_POINT('Ctrl Pts',(-44.467261544387,-4.33923083232682,-2.4696376464397));
#25633=CARTESIAN_POINT('Ctrl Pts',(-44.5068978773853,-4.62180401464078,
-1.70255770209476));
#25634=CARTESIAN_POINT('Ctrl Pts',(-44.5349847429557,-4.82203936400522,
-1.15899401573013));
#25635=CARTESIAN_POINT('Ctrl Pts',(-44.563071608526,-4.92431568889719,-0.579344661707689));
#25636=CARTESIAN_POINT('Ctrl Pts',(-44.5911584740964,-4.92485068894608,
0.000120817416453672));
#25637=CARTESIAN_POINT('Ctrl Pts',(-44.8088415259036,-4.9248046659208,0.000114993715491958));
#25638=CARTESIAN_POINT('Ctrl Pts',(-44.7815630393799,-4.92431719831031,
-0.562687752428751));
#25639=CARTESIAN_POINT('Ctrl Pts',(-44.7542845528562,-4.82796002993066,
-1.12565315150297));
#25640=CARTESIAN_POINT('Ctrl Pts',(-44.7270060663325,-4.63886048406004,
-1.65552057009204));
#25641=CARTESIAN_POINT('Ctrl Pts',(-44.6873697333342,-4.36409404628679,
-2.42543137250844));
#25642=CARTESIAN_POINT('Ctrl Pts',(-44.6477334003359,-3.89352222872223,
-3.12546298038023));
#25643=CARTESIAN_POINT('Ctrl Pts',(-44.6080970673376,-3.28431991956177,
-3.67056094000945));
#25644=CARTESIAN_POINT('Ctrl Pts',(-44.5684607343393,-2.6751176104013,-4.21565889963868));
#25645=CARTESIAN_POINT('Ctrl Pts',(-44.5288244013409,-1.92728480964494,
-4.60582321102533));
#25646=CARTESIAN_POINT('Ctrl Pts',(-44.4891880683426,-1.13168385802756,
-4.79364856812068));
#25647=CARTESIAN_POINT('Ctrl Pts',(-44.4495517353443,-0.336082906410188,
-4.98147392521603));
#25648=CARTESIAN_POINT('Ctrl Pts',(-44.409915402346,0.507286196068199,-4.96696032802006));
#25649=CARTESIAN_POINT('Ctrl Pts',(-44.3702790693476,1.29595336448566,-4.75187119188491));
#25650=CARTESIAN_POINT('Ctrl Pts',(-44.3306427363493,2.08462053290311,-4.53678205574976));
#25651=CARTESIAN_POINT('Ctrl Pts',(-44.291006403351,2.81858576725963,-4.12111738067542));
#25652=CARTESIAN_POINT('Ctrl Pts',(-44.2513700703527,3.40867164809488,-3.55538078781478));
#25653=CARTESIAN_POINT('Ctrl Pts',(-44.2117337373544,3.99875752893012,-2.98964419495414));
#25654=CARTESIAN_POINT('Ctrl Pts',(-44.1720974043561,4.44496405624409,-2.2738356843072));
#25655=CARTESIAN_POINT('Ctrl Pts',(-44.1324610713577,4.69307674644938,-1.49492661951182));
#25656=CARTESIAN_POINT('Ctrl Pts',(-44.0928247383594,4.94118943665468,-0.716017554716438));
#25657=CARTESIAN_POINT('Ctrl Pts',(-44.0531884053611,4.9912082897513,0.12599206422738));
#25658=CARTESIAN_POINT('Ctrl Pts',(-44.0135520723628,4.83705597021055,0.928797335259682));
#25659=CARTESIAN_POINT('Ctrl Pts',(-43.9739157393644,4.68290365066981,1.73160260629197));
#25660=CARTESIAN_POINT('Ctrl Pts',(-43.9342794063661,4.32458015849171,2.49520352941275));
#25661=CARTESIAN_POINT('Ctrl Pts',(-43.8946430733678,3.80562211407888,3.12682191418588));
#25662=CARTESIAN_POINT('Ctrl Pts',(-43.8550067403695,3.28666406966605,3.75844029895903));
#25663=CARTESIAN_POINT('Ctrl Pts',(-43.8153704073711,2.60707147301845,4.25807614538456));
#25664=CARTESIAN_POINT('Ctrl Pts',(-43.7757340743728,1.84941541605414,4.56502327837135));
#25665=CARTESIAN_POINT('Ctrl Pts',(-43.7360977413745,1.09175935908982,4.87197041135815));
#25666=CARTESIAN_POINT('Ctrl Pts',(-43.6964614083762,0.256039841808794,
4.98622883090624));
#25667=CARTESIAN_POINT('Ctrl Pts',(-43.6568250753779,-0.556202473766204,
4.89391600277317));
#25668=CARTESIAN_POINT('Ctrl Pts',(-43.6171887423796,-1.36844478934118,
4.80160317464009));
#25669=CARTESIAN_POINT('Ctrl Pts',(-43.5775524093812,-2.15720990321009,
4.50271909882586));
#25670=CARTESIAN_POINT('Ctrl Pts',(-43.5379160763829,-2.8266621792954,4.03357852455539));
#25671=CARTESIAN_POINT('Ctrl Pts',(-43.4982797433846,-3.49611445538071,
3.56443795028493));
#25672=CARTESIAN_POINT('Ctrl Pts',(-43.4586434103863,-4.04625389368242,
2.92504087755824));
#25673=CARTESIAN_POINT('Ctrl Pts',(-43.419007077388,-4.41023803739531,2.19307446727405));
#25674=CARTESIAN_POINT('Ctrl Pts',(-43.3822852268932,-4.7474582163777,1.51492997073843));
#25675=CARTESIAN_POINT('Ctrl Pts',(-43.3455633763984,-4.92489281945989,
0.757328991673029));
#25676=CARTESIAN_POINT('Ctrl Pts',(-43.3088415259036,-4.92535985208058,
-6.05620874156806E-5));
#25677=CARTESIAN_POINT('Origin',(-41.25,0.,0.));
#25678=CARTESIAN_POINT('',(-41.5911584740964,-4.92312360382807,0.0065423075118709));
#25679=CARTESIAN_POINT('',(-41.8088415259036,-4.92470507325415,0.000456942424287175));
#25680=CARTESIAN_POINT('',(-41.25,-4.925,-6.03138548580071E-16));
#25681=CARTESIAN_POINT('Ctrl Pts',(-41.5911584740964,-4.92312360382807,
0.0065423075118709));
#25682=CARTESIAN_POINT('Ctrl Pts',(-41.6117996165663,-4.92719160457478,
0.433012434324011));
#25683=CARTESIAN_POINT('Ctrl Pts',(-41.6324407590363,-4.87680224873628,
0.858320394691805));
#25684=CARTESIAN_POINT('Ctrl Pts',(-41.6530819015062,-4.76835722634153,
1.26767901413433));
#25685=CARTESIAN_POINT('Ctrl Pts',(-41.7323545675029,-4.35187223517315,
2.83982789877944));
#25686=CARTESIAN_POINT('Ctrl Pts',(-41.8116272334995,-3.07909091744468,
4.17673080563311));
#25687=CARTESIAN_POINT('Ctrl Pts',(-41.8908998994962,-1.52838050839828,
4.68726148274619));
#25688=CARTESIAN_POINT('Ctrl Pts',(-41.9305362324945,-0.753025303875076,
4.94252682130273));
#25689=CARTESIAN_POINT('Ctrl Pts',(-41.9701725654928,0.0918121734776089,
4.99119910242413));
#25690=CARTESIAN_POINT('Ctrl Pts',(-42.0098088984911,0.896430390440525,
4.84098316384975));
#25691=CARTESIAN_POINT('Ctrl Pts',(-42.0494452314894,1.70104860740344,4.69076722527537));
#25692=CARTESIAN_POINT('Ctrl Pts',(-42.0890815644878,2.46544756397659,4.34166306700522));
#25693=CARTESIAN_POINT('Ctrl Pts',(-42.1287178974861,3.10020506573018,3.82803047845904));
#25694=CARTESIAN_POINT('Ctrl Pts',(-42.1683542304844,3.7349625674838,3.31439788991284));
#25695=CARTESIAN_POINT('Ctrl Pts',(-42.2079905634827,4.24007861441785,2.63623687109061));
#25696=CARTESIAN_POINT('Ctrl Pts',(-42.247626896481,4.55242617457846,1.88020454684251));
#25697=CARTESIAN_POINT('Ctrl Pts',(-42.2872632294794,4.86477373473906,1.12417222259442));
#25698=CARTESIAN_POINT('Ctrl Pts',(-42.3268995624777,4.98435280812624,0.290268592920477));
#25699=CARTESIAN_POINT('Ctrl Pts',(-42.366535895476,4.89751528977223,-0.52233608303516));
#25700=CARTESIAN_POINT('Ctrl Pts',(-42.4061722284743,4.81067777141822,-1.3349407589908));
#25701=CARTESIAN_POINT('Ctrl Pts',(-42.4458085614726,4.51742366132304,-2.12624648122812));
#25702=CARTESIAN_POINT('Ctrl Pts',(-42.485444894471,4.05294203299736,-2.79903036183311));
#25703=CARTESIAN_POINT('Ctrl Pts',(-42.5250812274693,3.58846040467168,-3.47181424243811));
#25704=CARTESIAN_POINT('Ctrl Pts',(-42.5647175604676,2.95275125811554,-4.02607628141074));
#25705=CARTESIAN_POINT('Ctrl Pts',(-42.6043538934659,2.22327510854644,-4.3950137648464));
#25706=CARTESIAN_POINT('Ctrl Pts',(-42.6439902264642,1.49379895897736,-4.76395124828203));
#25707=CARTESIAN_POINT('Ctrl Pts',(-42.6836265594626,0.670555806395326,
-4.94756417618069));
#25708=CARTESIAN_POINT('Ctrl Pts',(-42.7232628924609,-0.146540489007751,
-4.9232724815208));
#25709=CARTESIAN_POINT('Ctrl Pts',(-42.7628992254592,-0.963636784410876,
-4.89898078686091));
#25710=CARTESIAN_POINT('Ctrl Pts',(-42.8025355584575,-1.77458622263507,
-4.66678446964245));
#25711=CARTESIAN_POINT('Ctrl Pts',(-42.8421718914558,-2.4808021561186,-4.2550313666284));
#25712=CARTESIAN_POINT('Ctrl Pts',(-42.8818082244542,-3.18701808960212,
-3.84327826361436));
#25713=CARTESIAN_POINT('Ctrl Pts',(-42.9214445574525,-3.78850051834497,
-3.25196837480472));
#25714=CARTESIAN_POINT('Ctrl Pts',(-42.9610808904508,-4.2121966543097,-2.55287832287441));
#25715=CARTESIAN_POINT('Ctrl Pts',(-43.0007172234491,-4.63589279027442,
-1.8537882709441));
#25716=CARTESIAN_POINT('Ctrl Pts',(-43.0403535564474,-4.88180263346103,
-1.04691805589312));
#25717=CARTESIAN_POINT('Ctrl Pts',(-43.0799898894458,-4.92003396319907,
-0.230337217966836));
#25718=CARTESIAN_POINT('Ctrl Pts',(-43.083712750996,-4.92362485914551,-0.153639471878947));
#25719=CARTESIAN_POINT('Ctrl Pts',(-43.0874356125462,-4.92538361617124,
-0.0768560587192995));
#25720=CARTESIAN_POINT('Ctrl Pts',(-43.0911584740964,-4.92532729948334,
-7.01527563526372E-5));
#25721=CARTESIAN_POINT('Ctrl Pts',(-43.3088415259036,-4.92535985208058,
-6.05620874156806E-5));
#25722=CARTESIAN_POINT('Ctrl Pts',(-43.3059270434001,-4.92539691879654,
-0.0601718738282288));
#25723=CARTESIAN_POINT('Ctrl Pts',(-43.3030125608965,-4.92431926118984,
-0.12028185379436));
#25724=CARTESIAN_POINT('Ctrl Pts',(-43.300098078393,-4.92211828943658,-0.180350673472536));
#25725=CARTESIAN_POINT('Ctrl Pts',(-43.2604617453947,-4.89218554864086,
-0.997273656093239));
#25726=CARTESIAN_POINT('Ctrl Pts',(-43.2208254123963,-4.65449121792534,
-1.80658387349296));
#25727=CARTESIAN_POINT('Ctrl Pts',(-43.181189079398,-4.23791523576072,-2.50994999714146));
#25728=CARTESIAN_POINT('Ctrl Pts',(-43.1415527463997,-3.8213392535961,-3.21331612078998));
#25729=CARTESIAN_POINT('Ctrl Pts',(-43.1019164134014,-3.22588161998236,
-3.81073815068729));
#25730=CARTESIAN_POINT('Ctrl Pts',(-43.0622800804031,-2.52389122059721,
-4.22962764535383));
#25731=CARTESIAN_POINT('Ctrl Pts',(-43.0226437474048,-1.82190082121208,
-4.64851714002037));
#25732=CARTESIAN_POINT('Ctrl Pts',(-42.9830074144065,-1.01337765605554,
-4.88887409945616));
#25733=CARTESIAN_POINT('Ctrl Pts',(-42.9433710814081,-0.196557476917921,
-4.92149721905324));
#25734=CARTESIAN_POINT('Ctrl Pts',(-42.9037347484098,0.620262702219694,
-4.95412033865032));
#25735=CARTESIAN_POINT('Ctrl Pts',(-42.8640984154114,1.44537989533838,-4.77900961840868));
#25736=CARTESIAN_POINT('Ctrl Pts',(-42.8244620824131,2.17854060041163,-4.41743662298954));
#25737=CARTESIAN_POINT('Ctrl Pts',(-42.7848257494148,2.91170130548488,-4.0558636275704));
#25738=CARTESIAN_POINT('Ctrl Pts',(-42.7451894164165,3.55290552251269,-3.50782835697374));
#25739=CARTESIAN_POINT('Ctrl Pts',(-42.7055530834182,4.02424845167079,-2.83992663573984));
#25740=CARTESIAN_POINT('Ctrl Pts',(-42.6659167504199,4.4955913808289,-2.17202491450593));
#25741=CARTESIAN_POINT('Ctrl Pts',(-42.6262804174215,4.79707302211729,-1.38425674263476));
#25742=CARTESIAN_POINT('Ctrl Pts',(-42.5866440844232,4.89205895380208,-0.572318572971036));
#25743=CARTESIAN_POINT('Ctrl Pts',(-42.5470077514249,4.98704488548686,0.239619596692683));
#25744=CARTESIAN_POINT('Ctrl Pts',(-42.5073714184266,4.87553510756804,1.07572776414893));
#25745=CARTESIAN_POINT('Ctrl Pts',(-42.4677350854283,4.57108641037318,1.83438200794185));
#25746=CARTESIAN_POINT('Ctrl Pts',(-42.42809875243,4.26663771317832,2.59303625173476));
#25747=CARTESIAN_POINT('Ctrl Pts',(-42.3884624194316,3.76925009670744,3.27423657186432));
#25748=CARTESIAN_POINT('Ctrl Pts',(-42.3488260864333,3.13934012622938,3.79528843677308));
#25749=CARTESIAN_POINT('Ctrl Pts',(-42.309189753435,2.5094301557513,4.31634030168184));
#25750=CARTESIAN_POINT('Ctrl Pts',(-42.2695534204367,1.74699783126604,4.6772437113698));
#25751=CARTESIAN_POINT('Ctrl Pts',(-42.2299170874383,0.94471219436256,4.83400515256402));
#25752=CARTESIAN_POINT('Ctrl Pts',(-42.19028075444,0.142426557459092,4.99076659375824));
#25753=CARTESIAN_POINT('Ctrl Pts',(-42.1506444214417,-0.6997123918626,4.94338606645873));
#25754=CARTESIAN_POINT('Ctrl Pts',(-42.1110080884434,-1.47944955361049,
4.69790646084692));
#25755=CARTESIAN_POINT('Ctrl Pts',(-42.0713717554451,-2.25918671535837,
4.45242685523511));
#25756=CARTESIAN_POINT('Ctrl Pts',(-42.0317354224467,-2.97652208953246,
4.00884817131102));
#25757=CARTESIAN_POINT('Ctrl Pts',(-41.9920990894484,-3.54416810026081,
3.42049488856083));
#25758=CARTESIAN_POINT('Ctrl Pts',(-41.9524627564501,-4.11181411098918,
2.83214160581061));
#25759=CARTESIAN_POINT('Ctrl Pts',(-41.9128264234518,-4.52977075827182,
2.09901372423428));
#25760=CARTESIAN_POINT('Ctrl Pts',(-41.8731900904534,-4.74751667129617,
1.31132519489558));
#25761=CARTESIAN_POINT('Ctrl Pts',(-41.8517405689368,-4.86535162961004,
0.885061189616368));
#25762=CARTESIAN_POINT('Ctrl Pts',(-41.8302910474202,-4.92455446234782,
0.442818986350074));
#25763=CARTESIAN_POINT('Ctrl Pts',(-41.8088415259036,-4.92470507325415,
0.000456942424287175));
#25764=CARTESIAN_POINT('Origin',(-41.25,0.,0.));
#25765=CARTESIAN_POINT('',(-40.0911584740964,-4.92524004259795,0.000110578359120081));
#25766=CARTESIAN_POINT('',(-40.3088415259036,-4.92524227782323,-0.000582878416294945));
#25767=CARTESIAN_POINT('',(-41.25,-4.925,-6.03138548580071E-16));
#25768=CARTESIAN_POINT('Ctrl Pts',(-40.0911584740964,-4.92524004259795,
0.000110578359120081));
#25769=CARTESIAN_POINT('Ctrl Pts',(-40.0965272875882,-4.92534070715902,
0.110850123093416));
#25770=CARTESIAN_POINT('Ctrl Pts',(-40.1018961010799,-4.92168160674078,
0.221582646226159));
#25771=CARTESIAN_POINT('Ctrl Pts',(-40.1072649145717,-4.91421674044945,
0.332057546016099));
#25772=CARTESIAN_POINT('Ctrl Pts',(-40.14690124757,-4.85910588093371,1.14766045767274));
#25773=CARTESIAN_POINT('Ctrl Pts',(-40.1865375805684,-4.5965646381192,1.94922180436547));
#25774=CARTESIAN_POINT('Ctrl Pts',(-40.2261739135667,-4.15849852897051,
2.63942441705466));
#25775=CARTESIAN_POINT('Ctrl Pts',(-40.265810246565,-3.72043241982181,3.32962702974388));
#25776=CARTESIAN_POINT('Ctrl Pts',(-40.3054465795633,-3.1068414443389,3.90847090842957));
#25777=CARTESIAN_POINT('Ctrl Pts',(-40.3450829125617,-2.39226442208597,
4.30547987767221));
#25778=CARTESIAN_POINT('Ctrl Pts',(-40.38471924556,-1.67768739983307,4.70248884691484));
#25779=CARTESIAN_POINT('Ctrl Pts',(-40.4243555785583,-0.862124330810157,
4.91766290671443));
#25780=CARTESIAN_POINT('Ctrl Pts',(-40.4639919115566,-0.0446928256683937,
4.92514982034103));
#25781=CARTESIAN_POINT('Ctrl Pts',(-40.5036282445549,0.772738679473369,
4.93263673396762));
#25782=CARTESIAN_POINT('Ctrl Pts',(-40.5432645775532,1.59203862073399,4.73243650142123));
#25783=CARTESIAN_POINT('Ctrl Pts',(-40.5829009105516,2.31371317843134,4.3482917815222));
#25784=CARTESIAN_POINT('Ctrl Pts',(-40.6225372435499,3.03538773612872,3.96414706162317));
#25785=CARTESIAN_POINT('Ctrl Pts',(-40.6621735765482,3.65943691026281,3.39605785437153));
#25786=CARTESIAN_POINT('Ctrl Pts',(-40.7018099095465,4.10993480374446,2.71420833875427));
#25787=CARTESIAN_POINT('Ctrl Pts',(-40.7414462425449,4.56043269722609,2.03235882313705));
#25788=CARTESIAN_POINT('Ctrl Pts',(-40.7810825755432,4.83737931005529,1.23674899915422));
#25789=CARTESIAN_POINT('Ctrl Pts',(-40.8207189085415,4.907330772549,0.421732025992796));
#25790=CARTESIAN_POINT('Ctrl Pts',(-40.8603552415398,4.97728223504271,-0.393284947168637));
#25791=CARTESIAN_POINT('Ctrl Pts',(-40.8999915745381,4.84023854720093,-1.22770906950873));
#25792=CARTESIAN_POINT('Ctrl Pts',(-40.9396279075365,4.51245206730997,-1.97556704108476));
#25793=CARTESIAN_POINT('Ctrl Pts',(-40.9792642405348,4.18466558741899,-2.72342501266081));
#25794=CARTESIAN_POINT('Ctrl Pts',(-41.0189005735331,3.66613631547886,-3.38471683347276));
#25795=CARTESIAN_POINT('Ctrl Pts',(-41.0585369065314,3.02050095021258,-3.88783737408691));
#25796=CARTESIAN_POINT('Ctrl Pts',(-41.0981732395297,2.37486558494632,-4.39095791470104));
#25797=CARTESIAN_POINT('Ctrl Pts',(-41.1378095725281,1.60212412635394,-4.73590717511732));
#25798=CARTESIAN_POINT('Ctrl Pts',(-41.1774459055264,0.796172436899315,
-4.86543694202377));
#25799=CARTESIAN_POINT('Ctrl Pts',(-41.256718571523,-0.815730942009943,
-5.12449647583667));
#25800=CARTESIAN_POINT('Ctrl Pts',(-41.3359912375197,-2.5604752443682,-4.52187803561028));
#25801=CARTESIAN_POINT('Ctrl Pts',(-41.4152639035163,-3.65275306324319,
-3.3168713842788));
#25802=CARTESIAN_POINT('Ctrl Pts',(-41.473895427043,-4.46062185168256,-2.42562627552507));
#25803=CARTESIAN_POINT('Ctrl Pts',(-41.5325269505697,-4.91156837708445,
-1.20485349143866));
#25804=CARTESIAN_POINT('Ctrl Pts',(-41.5911584740964,-4.92312360382807,
0.0065423075118709));
#25805=CARTESIAN_POINT('Ctrl Pts',(-41.8088415259036,-4.92470507325415,
0.000456942424287175));
#25806=CARTESIAN_POINT('Ctrl Pts',(-41.7906547144219,-4.9248327745718,-0.374616930123598));
#25807=CARTESIAN_POINT('Ctrl Pts',(-41.7724679029402,-4.88250691188772,
-0.749776957992148));
#25808=CARTESIAN_POINT('Ctrl Pts',(-41.7542810914585,-4.79747141108739,
-1.11535651178711));
#25809=CARTESIAN_POINT('Ctrl Pts',(-41.7146447584602,-4.61214505908818,
-1.91210051203008));
#25810=CARTESIAN_POINT('Ctrl Pts',(-41.6750084254619,-4.22395717632369,
-2.66333933541497));
#25811=CARTESIAN_POINT('Ctrl Pts',(-41.6353720924635,-3.68111291696794,
-3.27330228550321));
#25812=CARTESIAN_POINT('Ctrl Pts',(-41.5957357594652,-3.13826865761218,
-3.88326523559146));
#25813=CARTESIAN_POINT('Ctrl Pts',(-41.5560994264669,-2.44076802166517,
-4.35195231238306));
#25814=CARTESIAN_POINT('Ctrl Pts',(-41.5164630934686,-1.67125955808265,
-4.63093578122739));
#25815=CARTESIAN_POINT('Ctrl Pts',(-41.4768267604703,-0.901751094500133,
-4.90991925007172));
#25816=CARTESIAN_POINT('Ctrl Pts',(-41.4371904274719,-0.0602348032821162,
-4.99919911096879));
#25817=CARTESIAN_POINT('Ctrl Pts',(-41.3975540944736,0.746297840191277,
-4.87333819933832));
#25818=CARTESIAN_POINT('Ctrl Pts',(-41.318281428477,2.35936312713807,-4.62161637607737));
#25819=CARTESIAN_POINT('Ctrl Pts',(-41.2390087624803,3.83249382310637,-3.5093314627062));
#25820=CARTESIAN_POINT('Ctrl Pts',(-41.1597360964837,4.49894414693498,-2.02576869565901));
#25821=CARTESIAN_POINT('Ctrl Pts',(-41.0804634304871,5.16539447076359,-0.542205928611831));
#25822=CARTESIAN_POINT('Ctrl Pts',(-41.0011907644904,5.02516442245251,1.31263469211137));
#25823=CARTESIAN_POINT('Ctrl Pts',(-40.9219180984938,4.14324287363601,2.6791371251985));
#25824=CARTESIAN_POINT('Ctrl Pts',(-40.8426454324971,3.26132132481951,4.04563955828564));
#25825=CARTESIAN_POINT('Ctrl Pts',(-40.7633727665005,1.63770827549757,4.9238038037367));
#25826=CARTESIAN_POINT('Ctrl Pts',(-40.6841001005038,0.00513262720455543,
4.93014800260014));
#25827=CARTESIAN_POINT('Ctrl Pts',(-40.6444637675055,-0.811155196941947,
4.93332010203186));
#25828=CARTESIAN_POINT('Ctrl Pts',(-40.6048274345072,-1.62968367083122,
4.71853718981668));
#25829=CARTESIAN_POINT('Ctrl Pts',(-40.5651911015089,-2.34850178207576,
4.32703294416875));
#25830=CARTESIAN_POINT('Ctrl Pts',(-40.5255547685105,-3.06731989332033,
3.93552869852081));
#25831=CARTESIAN_POINT('Ctrl Pts',(-40.4859184355122,-3.68642764192017,
3.36730311944011));
#25832=CARTESIAN_POINT('Ctrl Pts',(-40.4462821025139,-4.13139676932224,
2.6826592952111));
#25833=CARTESIAN_POINT('Ctrl Pts',(-40.4066457695156,-4.5763658967243,1.99801547098211));
#25834=CARTESIAN_POINT('Ctrl Pts',(-40.3670094365173,-4.84719640292859,
1.19695340160483));
#25835=CARTESIAN_POINT('Ctrl Pts',(-40.327373103519,-4.91062970795906,0.381402621774772));
#25836=CARTESIAN_POINT('Ctrl Pts',(-40.3211959109805,-4.92051558056338,
0.254301706760495));
#25837=CARTESIAN_POINT('Ctrl Pts',(-40.3150187184421,-4.92536414836018,
0.126848887041597));
#25838=CARTESIAN_POINT('Ctrl Pts',(-40.3088415259036,-4.92524227782323,
-0.000582878416294945));
#25839=CARTESIAN_POINT('Origin',(-41.25,0.,0.));
#25840=CARTESIAN_POINT('',(-38.5911584740964,-4.92495184350011,-0.000126817359744069));
#25841=CARTESIAN_POINT('',(-38.8088415259036,-4.92500387630964,-0.000126728579282317));
#25842=CARTESIAN_POINT('',(-41.25,-4.925,-6.03138548580071E-16));
#25843=CARTESIAN_POINT('Ctrl Pts',(-38.5911584740964,-4.92495184350011,
-0.000126817359744069));
#25844=CARTESIAN_POINT('Ctrl Pts',(-38.6208912916084,-4.92433626585009,
0.613260413089466));
#25845=CARTESIAN_POINT('Ctrl Pts',(-38.6506241091203,-4.80942795756713,
1.226871817165));
#25846=CARTESIAN_POINT('Ctrl Pts',(-38.6803569266322,-4.58560283228258,
1.79778245415366));
#25847=CARTESIAN_POINT('Ctrl Pts',(-38.7199932596305,-4.2872252165181,2.55885409194545));
#25848=CARTESIAN_POINT('Ctrl Pts',(-38.7596295926288,-3.79529021528604,
3.2440416829727));
#25849=CARTESIAN_POINT('Ctrl Pts',(-38.7992659256272,-3.16956836399035,
3.77009435283018));
#25850=CARTESIAN_POINT('Ctrl Pts',(-38.8389022586255,-2.54384651269465,
4.29614702268767));
#25851=CARTESIAN_POINT('Ctrl Pts',(-38.8785385916238,-1.78433781133531,
4.66306477137538));
#25852=CARTESIAN_POINT('Ctrl Pts',(-38.9181749246221,-0.98332322946878,
4.82626673419433));
#25853=CARTESIAN_POINT('Ctrl Pts',(-38.9578112576204,-0.182308647602273,
4.98946869701328));
#25854=CARTESIAN_POINT('Ctrl Pts',(-38.9974475906188,0.660211814771426,
4.94895487396347));
#25855=CARTESIAN_POINT('Ctrl Pts',(-39.0370839236171,1.441871176594,4.70964780323818));
#25856=CARTESIAN_POINT('Ctrl Pts',(-39.0767202566154,2.22353053841658,4.47034073251288));
#25857=CARTESIAN_POINT('Ctrl Pts',(-39.1163565896137,2.94432879968803,4.03224041411209));
#25858=CARTESIAN_POINT('Ctrl Pts',(-39.155992922612,3.5166883529919,3.4485762746204));
#25859=CARTESIAN_POINT('Ctrl Pts',(-39.1956292556103,4.08904790629577,2.86491213512871));
#25860=CARTESIAN_POINT('Ctrl Pts',(-39.2352655886087,4.51296875163206,2.13568417454611));
#25861=CARTESIAN_POINT('Ctrl Pts',(-39.274901921607,4.73694410881552,1.3494945205605));
#25862=CARTESIAN_POINT('Ctrl Pts',(-39.3145382546053,4.96091946599899,0.563304866574897));
#25863=CARTESIAN_POINT('Ctrl Pts',(-39.3541745876036,4.98494933502962,-0.279846480813713));
#25864=CARTESIAN_POINT('Ctrl Pts',(-39.393810920602,4.80611411757365,-1.07751647545427));
#25865=CARTESIAN_POINT('Ctrl Pts',(-39.4334472536003,4.62727890011768,-1.87518647009483));
#25866=CARTESIAN_POINT('Ctrl Pts',(-39.4730835865986,4.2455785961751,-2.62737511198735));
#25867=CARTESIAN_POINT('Ctrl Pts',(-39.5127199195969,3.70739002379865,-3.242689661688));
#25868=CARTESIAN_POINT('Ctrl Pts',(-39.5523562525952,3.1692014514222,-3.85800421138865));
#25869=CARTESIAN_POINT('Ctrl Pts',(-39.5919925855936,2.47452461061189,-4.33644466889744));
#25870=CARTESIAN_POINT('Ctrl Pts',(-39.6316289185919,1.70776355261603,-4.61988241451491));
#25871=CARTESIAN_POINT('Ctrl Pts',(-39.6712652515902,0.941002494620145,
-4.90332016013239));
#25872=CARTESIAN_POINT('Ctrl Pts',(-39.7109015845885,0.102157219438717,
-4.99175519385855));
#25873=CARTESIAN_POINT('Ctrl Pts',(-39.7505379175868,-0.706852248500371,
-4.8744379618949));
#25874=CARTESIAN_POINT('Ctrl Pts',(-39.7901742505852,-1.51586171643944,
-4.75712072993124));
#25875=CARTESIAN_POINT('Ctrl Pts',(-39.8298105835835,-2.29503537713616,
-4.43405123227779));
#25876=CARTESIAN_POINT('Ctrl Pts',(-39.8694469165818,-2.94970212657891,
-3.94449191416061));
#25877=CARTESIAN_POINT('Ctrl Pts',(-39.9090832495801,-3.60436887602165,
-3.45493259604344));
#25878=CARTESIAN_POINT('Ctrl Pts',(-39.9487195825784,-4.13452871421041,
-2.79888345746255));
#25879=CARTESIAN_POINT('Ctrl Pts',(-39.9883559155767,-4.4757683951963,-2.05603664986182));
#25880=CARTESIAN_POINT('Ctrl Pts',(-40.0226234350833,-4.77078653991438,
-1.41380979525057));
#25881=CARTESIAN_POINT('Ctrl Pts',(-40.0568909545898,-4.92459753102333,
-0.706706582480056));
#25882=CARTESIAN_POINT('Ctrl Pts',(-40.0911584740964,-4.92524004259795,
0.000110578359120081));
#25883=CARTESIAN_POINT('Ctrl Pts',(-40.3088415259036,-4.92524227782323,
-0.000582878416294945));
#25884=CARTESIAN_POINT('Ctrl Pts',(-40.2753823854437,-4.92458215862047,
-0.690824814856074));
#25885=CARTESIAN_POINT('Ctrl Pts',(-40.2419232449839,-4.77809368542024,
-1.38044903752072));
#25886=CARTESIAN_POINT('Ctrl Pts',(-40.208464104524,-4.49640309152601,-2.01018594899038));
#25887=CARTESIAN_POINT('Ctrl Pts',(-40.1688277715257,-4.16270706620585,
-2.75618424964264));
#25888=CARTESIAN_POINT('Ctrl Pts',(-40.1291914385274,-3.63927891170889,
-3.41814136066434));
#25889=CARTESIAN_POINT('Ctrl Pts',(-40.0895551055291,-2.98962897640359,
-3.91446438086044));
#25890=CARTESIAN_POINT('Ctrl Pts',(-40.0499187725307,-2.33997904109829,
-4.41078740105654));
#25891=CARTESIAN_POINT('Ctrl Pts',(-40.0102824395324,-1.56410732498466,
-4.74147633042705));
#25892=CARTESIAN_POINT('Ctrl Pts',(-39.9706461065341,-0.756326330344129,
-4.86693605655279));
#25893=CARTESIAN_POINT('Ctrl Pts',(-39.9310097735357,0.0514546642963978,
-4.99239578267854));
#25894=CARTESIAN_POINT('Ctrl Pts',(-39.8913734405374,0.891144937463817,
-4.91262630555953));
#25895=CARTESIAN_POINT('Ctrl Pts',(-39.8517371075391,1.66074314480816,-4.63702697341363));
#25896=CARTESIAN_POINT('Ctrl Pts',(-39.8121007745408,2.43034135215252,-4.36142764126772));
#25897=CARTESIAN_POINT('Ctrl Pts',(-39.7724644415425,3.12984749367381,-3.8899984540949));
#25898=CARTESIAN_POINT('Ctrl Pts',(-39.7328281085442,3.6742600519052,-3.28016521191097));
#25899=CARTESIAN_POINT('Ctrl Pts',(-39.6931917755458,4.21867261013657,-2.67033196972706));
#25900=CARTESIAN_POINT('Ctrl Pts',(-39.6535554425475,4.60799158507806,-1.92209467253203));
#25901=CARTESIAN_POINT('Ctrl Pts',(-39.6139191095492,4.7949198484931,-1.12629124505432));
#25902=CARTESIAN_POINT('Ctrl Pts',(-39.5742827765509,4.98184811190814,-0.330487817576609));
#25903=CARTESIAN_POINT('Ctrl Pts',(-39.5346464435525,4.96638566379675,0.512881740183794));
#25904=CARTESIAN_POINT('Ctrl Pts',(-39.4950101105542,4.75040846378853,1.301310410167));
#25905=CARTESIAN_POINT('Ctrl Pts',(-39.4553737775559,4.53443126378031,2.08973908015021));
#25906=CARTESIAN_POINT('Ctrl Pts',(-39.4157374445576,4.11793931187527,2.82322686235623));
#25907=CARTESIAN_POINT('Ctrl Pts',(-39.3761011115593,3.55153811950529,3.41267283560264));
#25908=CARTESIAN_POINT('Ctrl Pts',(-39.3364647785609,2.98513692713531,4.00211880884906));
#25909=CARTESIAN_POINT('Ctrl Pts',(-39.2968284455626,2.26882649430039,4.44752297313588));
#25910=CARTESIAN_POINT('Ctrl Pts',(-39.2571921125643,1.48963847740388,4.69475906436197));
#25911=CARTESIAN_POINT('Ctrl Pts',(-39.217555779566,0.710450460507369,4.94199515558807));
#25912=CARTESIAN_POINT('Ctrl Pts',(-39.1779194465677,-0.131615140450732,
4.99106317375344));
#25913=CARTESIAN_POINT('Ctrl Pts',(-39.1382831135694,-0.934246271622569,
4.83600595769282));
#25914=CARTESIAN_POINT('Ctrl Pts',(-39.098646780571,-1.73687740279441,4.6809487416322));
#25915=CARTESIAN_POINT('Ctrl Pts',(-39.0590104475727,-2.50007406417998,
4.32176629134559));
#25916=CARTESIAN_POINT('Ctrl Pts',(-39.0193741145744,-3.13110736571771,
3.80209726021013));
#25917=CARTESIAN_POINT('Ctrl Pts',(-38.979737781576,-3.76214066725545,3.28242822907467));
#25918=CARTESIAN_POINT('Ctrl Pts',(-38.9401014485777,-4.26101060894535,
2.60227261709036));
#25919=CARTESIAN_POINT('Ctrl Pts',(-38.9004651155794,-4.56710396888216,
1.84427109478626));
#25920=CARTESIAN_POINT('Ctrl Pts',(-38.8699239190208,-4.80295972959322,
1.26020411045154));
#25921=CARTESIAN_POINT('Ctrl Pts',(-38.8393827224622,-4.92435926091217,
0.629918081833665));
#25922=CARTESIAN_POINT('Ctrl Pts',(-38.8088415259036,-4.92500387630964,
-0.000126728579282317));
#25923=CARTESIAN_POINT('Origin',(-41.25,0.,0.));
#25924=CARTESIAN_POINT('',(-37.0911584740964,-4.92470114822472,9.20081863105271E-5));
#25925=CARTESIAN_POINT('',(-37.3088415259036,-4.92466879478489,8.05726076643189E-5));
#25926=CARTESIAN_POINT('',(-41.25,-4.925,-6.03138548580071E-16));
#25927=CARTESIAN_POINT('Ctrl Pts',(-37.0911584740964,-4.92470114822472,
9.20081863105271E-5));
#25928=CARTESIAN_POINT('Ctrl Pts',(-37.1056189626302,-4.92490181486345,
0.29845508628429));
#25929=CARTESIAN_POINT('Ctrl Pts',(-37.1200794511639,-4.89822120621134,
0.596782699785559));
#25930=CARTESIAN_POINT('Ctrl Pts',(-37.1345399396977,-4.84432452014131,
0.890109556114513));
#25931=CARTESIAN_POINT('Ctrl Pts',(-37.174176272696,-4.69659320445376,1.69412118598857));
#25932=CARTESIAN_POINT('Ctrl Pts',(-37.2138126056943,-4.3443839128035,2.46056146826631));
#25933=CARTESIAN_POINT('Ctrl Pts',(-37.2534489386926,-3.83049038279097,
3.09630723696455));
#25934=CARTESIAN_POINT('Ctrl Pts',(-37.293085271691,-3.31659685277845,3.73205300566278));
#25935=CARTESIAN_POINT('Ctrl Pts',(-37.3327216046893,-2.64101908440367,
4.2371042607815));
#25936=CARTESIAN_POINT('Ctrl Pts',(-37.3723579376876,-1.88584036857968,
4.55009683221736));
#25937=CARTESIAN_POINT('Ctrl Pts',(-37.4119942706859,-1.13066165275566,
4.86308940365323));
#25938=CARTESIAN_POINT('Ctrl Pts',(-37.4516306036843,-0.295881989482435,
4.98402329140623));
#25939=CARTESIAN_POINT('Ctrl Pts',(-37.4912669366826,0.517072160578491,
4.89820492212251));
#25940=CARTESIAN_POINT('Ctrl Pts',(-37.5309032696809,1.33002631063939,4.81238655283879));
#25941=CARTESIAN_POINT('Ctrl Pts',(-37.5705396026792,2.12115494748799,4.51981592651836));
#25942=CARTESIAN_POINT('Ctrl Pts',(-37.6101759356775,2.79433524842529,4.05604063067722));
#25943=CARTESIAN_POINT('Ctrl Pts',(-37.6498122686759,3.46751554936259,3.59226533483608));
#25944=CARTESIAN_POINT('Ctrl Pts',(-37.6894486016742,4.0227475143886,2.95728536947423));
#25945=CARTESIAN_POINT('Ctrl Pts',(-37.7290849346725,4.39256997316809,2.22825135682294));
#25946=CARTESIAN_POINT('Ctrl Pts',(-37.7687212676708,4.76239243194758,1.49921734417164));
#25947=CARTESIAN_POINT('Ctrl Pts',(-37.8083576006691,4.94680538448055,0.676129284230918));
#25948=CARTESIAN_POINT('Ctrl Pts',(-37.8479939336675,4.92340249541402,-0.141006902314823));
#25949=CARTESIAN_POINT('Ctrl Pts',(-37.8876302666658,4.89999960634749,-0.958143088860554));
#25950=CARTESIAN_POINT('Ctrl Pts',(-37.9272665996641,4.66878087568145,-1.76932740201133));
#25951=CARTESIAN_POINT('Ctrl Pts',(-37.9669029326624,4.25783958183768,-2.4760002369688));
#25952=CARTESIAN_POINT('Ctrl Pts',(-38.0065392656607,3.84689828799389,-3.18267307192628));
#25953=CARTESIAN_POINT('Ctrl Pts',(-38.0461755986591,3.25623443097236,-3.78483442869049));
#25954=CARTESIAN_POINT('Ctrl Pts',(-38.0858119316574,2.55761418701446,-4.20932117440809));
#25955=CARTESIAN_POINT('Ctrl Pts',(-38.1254482646557,1.85899394305657,-4.63380792012569));
#25956=CARTESIAN_POINT('Ctrl Pts',(-38.165084597654,1.05241731216232,-4.88062005479668));
#25957=CARTESIAN_POINT('Ctrl Pts',(-38.2047209306523,0.235884061895514,
-4.91976968834123));
#25958=CARTESIAN_POINT('Ctrl Pts',(-38.2443572636507,-0.580649188371287,
-4.95891932188577));
#25959=CARTESIAN_POINT('Ctrl Pts',(-38.283993596649,-1.40713905801063,-4.79040645430388));
#25960=CARTESIAN_POINT('Ctrl Pts',(-38.3236299296473,-2.14316630365493,
-4.43470554552663));
#25961=CARTESIAN_POINT('Ctrl Pts',(-38.3632662626456,-2.87919354929924,
-4.07900463674938));
#25962=CARTESIAN_POINT('Ctrl Pts',(-38.4029025956439,-3.52475817094849,
-3.53611568677679));
#25963=CARTESIAN_POINT('Ctrl Pts',(-38.4425389286422,-4.00142350111364,
-2.87200018111494));
#25964=CARTESIAN_POINT('Ctrl Pts',(-38.4821752616406,-4.47808883127881,
-2.20788467545306));
#25965=CARTESIAN_POINT('Ctrl Pts',(-38.5218115946389,-4.78585486995985,
-1.42254261410192));
#25966=CARTESIAN_POINT('Ctrl Pts',(-38.5614479276372,-4.88732777415191,
-0.611393741148177));
#25967=CARTESIAN_POINT('Ctrl Pts',(-38.5713514431236,-4.9126817461795,-0.408720465963794));
#25968=CARTESIAN_POINT('Ctrl Pts',(-38.58125495861,-4.9251568823528,-0.204436077101899));
#25969=CARTESIAN_POINT('Ctrl Pts',(-38.5911584740964,-4.92495184350011,
-0.000126817359744069));
#25970=CARTESIAN_POINT('Ctrl Pts',(-38.8088415259036,-4.92500387630964,
-0.000126728579282317));
#25971=CARTESIAN_POINT('Ctrl Pts',(-38.7997463894639,-4.92519584210181,
-0.187753415138211));
#25972=CARTESIAN_POINT('Ctrl Pts',(-38.7906512530242,-4.91467875260689,
-0.37535870944927));
#25973=CARTESIAN_POINT('Ctrl Pts',(-38.7815561165845,-4.89328625908847,
-0.561715592844029));
#25974=CARTESIAN_POINT('Ctrl Pts',(-38.7419197835861,-4.80005841117423,
-1.37385332554627));
#25975=CARTESIAN_POINT('Ctrl Pts',(-38.7022834505878,-4.50028593716205,
-2.16228135832685));
#25976=CARTESIAN_POINT('Ctrl Pts',(-38.6626471175895,-4.03039143354269,
-2.83120470081615));
#25977=CARTESIAN_POINT('Ctrl Pts',(-38.6230107845912,-3.56049692992333,
-3.50012804330547));
#25978=CARTESIAN_POINT('Ctrl Pts',(-38.5833744515929,-2.92048039669678,
-4.04954669550349));
#25979=CARTESIAN_POINT('Ctrl Pts',(-38.5437381185945,-2.18810441447545,
-4.41270595677602));
#25980=CARTESIAN_POINT('Ctrl Pts',(-38.5041017855962,-1.45572843225415,
-4.77586521804853));
#25981=CARTESIAN_POINT('Ctrl Pts',(-38.4644654525979,-0.630993001038065,
-4.95276508839556));
#25982=CARTESIAN_POINT('Ctrl Pts',(-38.4248291195996,0.185895806989685,
-4.92191200479718));
#25983=CARTESIAN_POINT('Ctrl Pts',(-38.3851927866013,1.00278461501741,-4.89105892119881));
#25984=CARTESIAN_POINT('Ctrl Pts',(-38.3455564536029,1.81182679985681,-4.65245288365504));
#25985=CARTESIAN_POINT('Ctrl Pts',(-38.3059201206046,2.51472302428267,-4.23508477180253));
#25986=CARTESIAN_POINT('Ctrl Pts',(-38.2662837876063,3.21761924870857,-3.81771665994999));
#25987=CARTESIAN_POINT('Ctrl Pts',(-38.226647454608,3.81436951272092,-3.22158647378869));
#25988=CARTESIAN_POINT('Ctrl Pts',(-38.1870111216097,4.23246813764672,-2.5191245348344));
#25989=CARTESIAN_POINT('Ctrl Pts',(-38.1473747886113,4.6505667625725,-1.81666259588013));
#25990=CARTESIAN_POINT('Ctrl Pts',(-38.107738455613,4.89001374841174,-1.00786890413288));
#25991=CARTESIAN_POINT('Ctrl Pts',(-38.0681021226147,4.92171607585052,-0.191012611231857));
#25992=CARTESIAN_POINT('Ctrl Pts',(-38.0284657896164,4.95341840328931,0.625843681669167));
#25993=CARTESIAN_POINT('Ctrl Pts',(-37.988829456618,4.77737607232763,1.45076257572397));
#25994=CARTESIAN_POINT('Ctrl Pts',(-37.9491931236197,4.41497838080154,2.18351570702937));
#25995=CARTESIAN_POINT('Ctrl Pts',(-37.9095567906214,4.05258068927544,2.91626883833478));
#25996=CARTESIAN_POINT('Ctrl Pts',(-37.8699204576231,3.50382763718491,3.55685620689079));
#25997=CARTESIAN_POINT('Ctrl Pts',(-37.8302841246248,2.8353932010953,4.02744588369239));
#25998=CARTESIAN_POINT('Ctrl Pts',(-37.7906477916265,2.1669587650057,4.498035560494));
#25999=CARTESIAN_POINT('Ctrl Pts',(-37.7510114586281,1.37884294491701,4.79862754554121));
#26000=CARTESIAN_POINT('Ctrl Pts',(-37.7113751256298,0.566802503736936,
4.89269965039189));
#26001=CARTESIAN_POINT('Ctrl Pts',(-37.6717387926315,-0.245237937443135,
4.98677175524258));
#26002=CARTESIAN_POINT('Ctrl Pts',(-37.6321024596332,-1.08120299971459,
4.87432397989675));
#26003=CARTESIAN_POINT('Ctrl Pts',(-37.5924661266348,-1.83952219544158,
4.56901882701783));
#26004=CARTESIAN_POINT('Ctrl Pts',(-37.5528297936365,-2.59784139116857,
4.26371367413892));
#26005=CARTESIAN_POINT('Ctrl Pts',(-37.5131934606382,-3.2785147203511,3.76555114372692));
#26006=CARTESIAN_POINT('Ctrl Pts',(-37.4735571276399,-3.79883977695093,
3.13505842009503));
#26007=CARTESIAN_POINT('Ctrl Pts',(-37.4339207946416,-4.31916483355077,
2.50456569646312));
#26008=CARTESIAN_POINT('Ctrl Pts',(-37.3942844616432,-4.6791416175679,1.7417427796113));
#26009=CARTESIAN_POINT('Ctrl Pts',(-37.3546481286449,-4.83503263428287,
0.939273322303626));
#26010=CARTESIAN_POINT('Ctrl Pts',(-37.3393792610645,-4.89508559859979,
0.63014281112589));
#26011=CARTESIAN_POINT('Ctrl Pts',(-37.324110393484,-4.92485273578263,0.315128850619065));
#26012=CARTESIAN_POINT('Ctrl Pts',(-37.3088415259036,-4.92466879478489,
8.05726076643189E-5));
#26013=CARTESIAN_POINT('Origin',(-41.25,0.,0.));
#26014=CARTESIAN_POINT('',(-35.5911584740964,-4.92541600273781,-1.76250312958204E-5));
#26015=CARTESIAN_POINT('',(-35.8088415259036,-4.92542129650244,-7.54510851721086E-8));
#26016=CARTESIAN_POINT('',(-41.25,-4.925,-6.03138548580071E-16));
#26017=CARTESIAN_POINT('Ctrl Pts',(-35.5911584740964,-4.92541600273781,
-1.76250312958204E-5));
#26018=CARTESIAN_POINT('Ctrl Pts',(-35.6299829666503,-4.9252530757446,0.80071250682744));
#26019=CARTESIAN_POINT('Ctrl Pts',(-35.6688074592043,-4.72610527736418,
1.6015207460239));
#26020=CARTESIAN_POINT('Ctrl Pts',(-35.7076319517582,-4.35075868010393,
2.30882523934354));
#26021=CARTESIAN_POINT('Ctrl Pts',(-35.7472682847565,-3.96756338918973,
3.0309198395368));
#26022=CARTESIAN_POINT('Ctrl Pts',(-35.7869046177548,-3.4007234384037,3.65555938488601));
#26023=CARTESIAN_POINT('Ctrl Pts',(-35.8265409507531,-2.71911037852704,
4.1068496232168));
#26024=CARTESIAN_POINT('Ctrl Pts',(-35.8661772837514,-2.03749731865039,
4.55813986154758));
#26025=CARTESIAN_POINT('Ctrl Pts',(-35.9058136167498,-1.2411111496831,4.83608079285994));
#26026=CARTESIAN_POINT('Ctrl Pts',(-35.9454499497481,-0.426713489082491,
4.90690235042073));
#26027=CARTESIAN_POINT('Ctrl Pts',(-35.9850862827464,0.387684171518116,
4.97772390798152));
#26028=CARTESIAN_POINT('Ctrl Pts',(-36.0247226157447,1.22009332375204,4.84142609179075));
#26029=CARTESIAN_POINT('Ctrl Pts',(-36.064358948743,1.96937552612566,4.5145692059627));
#26030=CARTESIAN_POINT('Ctrl Pts',(-36.1039952817413,2.71865772849929,4.18771232013466));
#26031=CARTESIAN_POINT('Ctrl Pts',(-36.1436316147397,3.38481298101262,3.67029636466934));
#26032=CARTESIAN_POINT('Ctrl Pts',(-36.183267947738,3.88690283668777,3.02518783160286));
#26033=CARTESIAN_POINT('Ctrl Pts',(-36.2229042807363,4.38899269236293,2.38007929853637));
#26034=CARTESIAN_POINT('Ctrl Pts',(-36.2625406137347,4.7270171511999,1.6072781878687));
#26035=CARTESIAN_POINT('Ctrl Pts',(-36.302176946733,4.859905945216,0.800680511804564));
#26036=CARTESIAN_POINT('Ctrl Pts',(-36.3418132797313,4.99279473923209,-0.00591716425955069));
#26037=CARTESIAN_POINT('Ctrl Pts',(-36.3814496127296,4.92054786842731,-0.846311405720133));
#26038=CARTESIAN_POINT('Ctrl Pts',(-36.4210859457279,4.65194339091933,-1.61839357574463));
#26039=CARTESIAN_POINT('Ctrl Pts',(-36.4607222787262,4.38333891341134,-2.39047574576912));
#26040=CARTESIAN_POINT('Ctrl Pts',(-36.5003586117246,3.91837682920014,-3.09424584435753));
#26041=CARTESIAN_POINT('Ctrl Pts',(-36.5399949447229,3.31355043899555,-3.64419518776942));
#26042=CARTESIAN_POINT('Ctrl Pts',(-36.5796312777212,2.70872404879096,-4.1941445311813));
#26043=CARTESIAN_POINT('Ctrl Pts',(-36.6192676107195,1.96403335259296,-4.59027311941667));
#26044=CARTESIAN_POINT('Ctrl Pts',(-36.6589039437178,1.16995892261312,-4.78445098185022));
#26045=CARTESIAN_POINT('Ctrl Pts',(-36.6985402767162,0.375884492633281,
-4.97862884428377));
#26046=CARTESIAN_POINT('Ctrl Pts',(-36.7381766097145,-0.467573671128411,
-4.97085598091549));
#26047=CARTESIAN_POINT('Ctrl Pts',(-36.7778129427128,-1.25793466259469,
-4.76207680145668));
#26048=CARTESIAN_POINT('Ctrl Pts',(-36.8174492757111,-2.048295654061,-4.55329762199787));
#26049=CARTESIAN_POINT('Ctrl Pts',(-36.8570856087095,-2.78555947323189,
-4.1435121264485));
#26050=CARTESIAN_POINT('Ctrl Pts',(-36.8967219417078,-3.3801479199633,-3.58250961164066));
#26051=CARTESIAN_POINT('Ctrl Pts',(-36.9363582747061,-3.9747363666947,-3.02150709683283));
#26052=CARTESIAN_POINT('Ctrl Pts',(-36.9759946077044,-4.42664944098663,
-2.30928756276654));
#26053=CARTESIAN_POINT('Ctrl Pts',(-37.0156309407027,-4.68097930827017,
-1.53238630699822));
#26054=CARTESIAN_POINT('Ctrl Pts',(-37.0408067851673,-4.84252223358805,
-1.03892125359955));
#26055=CARTESIAN_POINT('Ctrl Pts',(-37.0659826296318,-4.92435178574819,
-0.51936087410214));
#26056=CARTESIAN_POINT('Ctrl Pts',(-37.0911584740964,-4.92470114822472,
9.20081863105271E-5));
#26057=CARTESIAN_POINT('Ctrl Pts',(-37.3088415259036,-4.92466879478489,
8.05726076643189E-5));
#26058=CARTESIAN_POINT('Ctrl Pts',(-37.2844740604857,-4.92437524479646,
-0.502702490966497));
#26059=CARTESIAN_POINT('Ctrl Pts',(-37.2601065950678,-4.84780014286267,
-1.00557295682021));
#26060=CARTESIAN_POINT('Ctrl Pts',(-37.23573912965,-4.69630408694853,-1.48475683918074));
#26061=CARTESIAN_POINT('Ctrl Pts',(-37.1961027966517,-4.44987927348641,
-2.26420154559395));
#26062=CARTESIAN_POINT('Ctrl Pts',(-37.1564664636533,-4.00522439714935,
-2.98097496065685));
#26063=CARTESIAN_POINT('Ctrl Pts',(-37.116830130655,-3.4163654150966,-3.54798848631869));
#26064=CARTESIAN_POINT('Ctrl Pts',(-37.0771937976567,-2.82750643304386,
-4.11500201198053));
#26065=CARTESIAN_POINT('Ctrl Pts',(-37.0375574646584,-2.09444334527543,
-4.53225564824131));
#26066=CARTESIAN_POINT('Ctrl Pts',(-36.99792113166,-1.30624395938722,-4.74905271260881));
#26067=CARTESIAN_POINT('Ctrl Pts',(-36.9582847986617,-0.518044573499021,
-4.96584977697631));
#26068=CARTESIAN_POINT('Ctrl Pts',(-36.9186484656634,0.325291110508953,
-4.98219026945052));
#26069=CARTESIAN_POINT('Ctrl Pts',(-36.8790121326651,1.12129706795617,-4.79608880588485));
#26070=CARTESIAN_POINT('Ctrl Pts',(-36.8393757996668,1.91730302540342,-4.60998734231918));
#26071=CARTESIAN_POINT('Ctrl Pts',(-36.7997394666684,2.66597925628991,-4.22144392271361));
#26072=CARTESIAN_POINT('Ctrl Pts',(-36.7601031336701,3.27636094244697,-3.67766691305279));
#26073=CARTESIAN_POINT('Ctrl Pts',(-36.7204668006718,3.88674262860402,-3.13388990339198));
#26074=CARTESIAN_POINT('Ctrl Pts',(-36.6808304676735,4.35882977003166,-2.43487930367593));
#26075=CARTESIAN_POINT('Ctrl Pts',(-36.6411941346751,4.63526336532393,-1.66556551436338));
#26076=CARTESIAN_POINT('Ctrl Pts',(-36.6015578016768,4.91169696061621,-0.896251725050832));
#26077=CARTESIAN_POINT('Ctrl Pts',(-36.5619214686785,4.99247700977312,-0.0566347461417782));
#26078=CARTESIAN_POINT('Ctrl Pts',(-36.5222851356802,4.86778866602909,0.751271223613593));
#26079=CARTESIAN_POINT('Ctrl Pts',(-36.4826488026819,4.74310032228506,1.55917719336896));
#26080=CARTESIAN_POINT('Ctrl Pts',(-36.4430124696835,4.4129435856401,2.33537215397065));
#26081=CARTESIAN_POINT('Ctrl Pts',(-36.4033761366852,3.9174327889355,2.98554773747212));
#26082=CARTESIAN_POINT('Ctrl Pts',(-36.3637398036869,3.4219219922309,3.63572332097359));
#26083=CARTESIAN_POINT('Ctrl Pts',(-36.3241034706886,2.76105713546667,4.15987952737483));
#26084=CARTESIAN_POINT('Ctrl Pts',(-36.2844671376903,2.01513387790084,4.49433091824439));
#26085=CARTESIAN_POINT('Ctrl Pts',(-36.244830804692,1.26921062033501,4.82878230911394));
#26086=CARTESIAN_POINT('Ctrl Pts',(-36.2051944716936,0.438228961967596,
4.97352888445181));
#26087=CARTESIAN_POINT('Ctrl Pts',(-36.1655581386953,-0.376846097463596,
4.91098380850294));
#26088=CARTESIAN_POINT('Ctrl Pts',(-36.125921805697,-1.19192115689479,4.84843873255408));
#26089=CARTESIAN_POINT('Ctrl Pts',(-36.0862854726987,-1.99108961738975,
4.57860200531848));
#26090=CARTESIAN_POINT('Ctrl Pts',(-36.0466491397003,-2.67725181063225,
4.13425902563176));
#26091=CARTESIAN_POINT('Ctrl Pts',(-36.007012806702,-3.36341400387475,3.68991604594505));
#26092=CARTESIAN_POINT('Ctrl Pts',(-35.9673764737037,-3.93656992986478,
3.07106681380722));
#26093=CARTESIAN_POINT('Ctrl Pts',(-35.9277401407054,-4.32708064129874,
2.35290205326299));
#26094=CARTESIAN_POINT('Ctrl Pts',(-35.8881072691048,-4.7175572498583,1.63480000926379));
#26095=CARTESIAN_POINT('Ctrl Pts',(-35.8484743975042,-4.92542054288352,
0.817399782334272));
#26096=CARTESIAN_POINT('Ctrl Pts',(-35.8088415259036,-4.92542129645401,
-7.54510764981203E-8));
#26097=CARTESIAN_POINT('Origin',(-41.25,0.,0.));
#26098=CARTESIAN_POINT('',(-34.0911584740964,-4.92464097398149,-6.78464643288912E-5));
#26099=CARTESIAN_POINT('',(-34.3088415259036,-4.92466853775765,-8.04693041996219E-5));
#26100=CARTESIAN_POINT('',(-41.25,-4.925,-6.03138548580071E-16));
#26101=CARTESIAN_POINT('Ctrl Pts',(-34.0911584740964,-4.92464097398149,
-6.78464643288912E-5));
#26102=CARTESIAN_POINT('Ctrl Pts',(-34.1147106376722,-4.92440379270329,
0.485900653683976));
#26103=CARTESIAN_POINT('Ctrl Pts',(-34.1382628012479,-4.85294370455535,
0.97193739581646));
#26104=CARTESIAN_POINT('Ctrl Pts',(-34.1618149648236,-4.71126926056628,
1.43656431557125));
#26105=CARTESIAN_POINT('Ctrl Pts',(-34.201451297822,-4.47284295118532,2.21849278902783));
#26106=CARTESIAN_POINT('Ctrl Pts',(-34.2410876308203,-4.03555490192482,
2.93978416801083));
#26107=CARTESIAN_POINT('Ctrl Pts',(-34.2807239638186,-3.45253599399545,
3.51280091785676));
#26108=CARTESIAN_POINT('Ctrl Pts',(-34.320360296817,-2.86951708606611,4.08581766770266));
#26109=CARTESIAN_POINT('Ctrl Pts',(-34.3599966298152,-2.1407673194679,4.51055978841149));
#26110=CARTESIAN_POINT('Ctrl Pts',(-34.3996329628136,-1.35483042949589,
4.73542074008651));
#26111=CARTESIAN_POINT('Ctrl Pts',(-34.4392692958119,-0.568893539523873,
4.96028169176152));
#26112=CARTESIAN_POINT('Ctrl Pts',(-34.4789056288102,0.274230473821956,
4.98526147440271));
#26113=CARTESIAN_POINT('Ctrl Pts',(-34.5185419618086,1.07210130403271,4.80732502252769));
#26114=CARTESIAN_POINT('Ctrl Pts',(-34.5581782948069,1.86997213424345,4.62938857065266));
#26115=CARTESIAN_POINT('Ctrl Pts',(-34.5978146278052,2.62258978131911,4.24853588426143));
#26116=CARTESIAN_POINT('Ctrl Pts',(-34.6374509608035,3.23851054156959,3.71104089851783));
#26117=CARTESIAN_POINT('Ctrl Pts',(-34.6770872938018,3.85443130182009,3.17354591277422));
#26118=CARTESIAN_POINT('Ctrl Pts',(-34.7167236268002,4.3336551752454,2.47940862767824));
#26119=CARTESIAN_POINT('Ctrl Pts',(-34.7563599597985,4.61795604124761,1.71296733168913));
#26120=CARTESIAN_POINT('Ctrl Pts',(-34.7959962927968,4.90225690724982,0.946526035699991));
#26121=CARTESIAN_POINT('Ctrl Pts',(-34.8356326257951,4.99163476582893,0.107780728817722));
#26122=CARTESIAN_POINT('Ctrl Pts',(-34.8752689587934,4.87523012883963,-0.701360299121477));
#26123=CARTESIAN_POINT('Ctrl Pts',(-34.9149052917917,4.75882549185033,-1.51050132706065));
#26124=CARTESIAN_POINT('Ctrl Pts',(-34.9545416247901,4.43663835929263,-2.29003807605676));
#26125=CARTESIAN_POINT('Ctrl Pts',(-34.9941779577884,3.94781475012695,-2.94525614794529));
#26126=CARTESIAN_POINT('Ctrl Pts',(-35.0338142907867,3.45899114096128,-3.60047421983382));
#26127=CARTESIAN_POINT('Ctrl Pts',(-35.073450623785,2.80353105518763,-4.13137361461476));
#26128=CARTESIAN_POINT('Ctrl Pts',(-35.1130869567833,2.0610734676521,-4.47344959055872));
#26129=CARTESIAN_POINT('Ctrl Pts',(-35.1527232897817,1.31861588011658,-4.81552556650267));
#26130=CARTESIAN_POINT('Ctrl Pts',(-35.19235962278,0.489160790819186,-4.96877812360963));
#26131=CARTESIAN_POINT('Ctrl Pts',(-35.2319959557783,-0.326512279982104,
-4.91458694188538));
#26132=CARTESIAN_POINT('Ctrl Pts',(-35.2716322887766,-1.14218535078339,
-4.86039576016113));
#26133=CARTESIAN_POINT('Ctrl Pts',(-35.3112686217749,-1.94407640308858,
-4.59876083960567));
#26134=CARTESIAN_POINT('Ctrl Pts',(-35.3509049547733,-2.63475497129048,
-4.16147105235511));
#26135=CARTESIAN_POINT('Ctrl Pts',(-35.3905412877716,-3.32543353949239,
-3.72418126510454));
#26136=CARTESIAN_POINT('Ctrl Pts',(-35.4301776207699,-3.90489962359101,
-3.11123661115887));
#26137=CARTESIAN_POINT('Ctrl Pts',(-35.4698139537682,-4.30274758654252,
-2.3971104031379));
#26138=CARTESIAN_POINT('Ctrl Pts',(-35.5094502867666,-4.70059554949403,
-1.68298419511693));
#26139=CARTESIAN_POINT('Ctrl Pts',(-35.5490866197649,-4.91682539129844,
-0.867676433020666));
#26140=CARTESIAN_POINT('Ctrl Pts',(-35.5887229527632,-4.92516499667947,
-0.0502477244538784));
#26141=CARTESIAN_POINT('Ctrl Pts',(-35.5895347932076,-4.92533581038564,
-0.0335049625525403));
#26142=CARTESIAN_POINT('Ctrl Pts',(-35.590346633652,-4.92541940962645,-0.0167613108681338));
#26143=CARTESIAN_POINT('Ctrl Pts',(-35.5911584740964,-4.92541600273781,
-1.76250312958204E-5));
#26144=CARTESIAN_POINT('Ctrl Pts',(-35.8088415259036,-4.92542129645401,
-7.54510764981203E-8));
#26145=CARTESIAN_POINT('Ctrl Pts',(-35.7692017315076,-4.92542205015613,
-0.817542710980693));
#26146=CARTESIAN_POINT('Ctrl Pts',(-35.7295619371115,-4.71748323020035,
-1.63508497704526));
#26147=CARTESIAN_POINT('Ctrl Pts',(-35.6899221427155,-4.32687593559207,
-2.35327847619989));
#26148=CARTESIAN_POINT('Ctrl Pts',(-35.6502858097172,-3.93630274931405,
-3.07140926177648));
#26149=CARTESIAN_POINT('Ctrl Pts',(-35.6106494767188,-3.36309298906717,
-3.69020863020926));
#26150=CARTESIAN_POINT('Ctrl Pts',(-35.5710131437205,-2.67689214306444,
-4.13449191593736));
#26151=CARTESIAN_POINT('Ctrl Pts',(-35.5313768107222,-1.99069129706169,
-4.57877520166546));
#26152=CARTESIAN_POINT('Ctrl Pts',(-35.4917404777239,-1.19149936530308,
-4.84854240468886));
#26153=CARTESIAN_POINT('Ctrl Pts',(-35.4521041447255,-0.376418867883944,
-4.91101657342473));
#26154=CARTESIAN_POINT('Ctrl Pts',(-35.4124678117272,0.438661629535188,
-4.9734907421606));
#26155=CARTESIAN_POINT('Ctrl Pts',(-35.3728314787289,1.26963069261483,-4.82867187660894));
#26156=CARTESIAN_POINT('Ctrl Pts',(-35.3331951457306,2.01552485195566,-4.49415559584896));
#26157=CARTESIAN_POINT('Ctrl Pts',(-35.2935588127323,2.76141901129648,-4.159639315089));
#26158=CARTESIAN_POINT('Ctrl Pts',(-35.2539224797339,3.42223826689847,-3.63542561912073));
#26159=CARTESIAN_POINT('Ctrl Pts',(-35.2142861467356,3.91769250008482,-2.98520693140871));
#26160=CARTESIAN_POINT('Ctrl Pts',(-35.1746498137373,4.41314673327116,-2.33498824369668));
#26161=CARTESIAN_POINT('Ctrl Pts',(-35.135013480739,4.74323594404185,-1.5587645642409));
#26162=CARTESIAN_POINT('Ctrl Pts',(-35.0953771477407,4.86785400400843,-0.750847750353243));
#26163=CARTESIAN_POINT('Ctrl Pts',(-35.0557408147424,4.99247206397501,0.0570690635343918));
#26164=CARTESIAN_POINT('Ctrl Pts',(-35.016104481744,4.9116189731375,0.896679011853955));
#26165=CARTESIAN_POINT('Ctrl Pts',(-34.9764681487457,4.63511845288976,1.66596875007676));
#26166=CARTESIAN_POINT('Ctrl Pts',(-34.9368318157474,4.35861793264201,2.43525848829959));
#26167=CARTESIAN_POINT('Ctrl Pts',(-34.897195482749,3.88646998298403,3.1342280164257));
#26168=CARTESIAN_POINT('Ctrl Pts',(-34.8575591497507,3.27604099357486,3.6779519242329));
#26169=CARTESIAN_POINT('Ctrl Pts',(-34.8179228167524,2.66561200416568,4.22167583204011));
#26170=CARTESIAN_POINT('Ctrl Pts',(-34.7782864837541,1.91690197500532,4.61015411952837));
#26171=CARTESIAN_POINT('Ctrl Pts',(-34.7386501507558,1.12087983078267,4.79618633431772));
#26172=CARTESIAN_POINT('Ctrl Pts',(-34.6990138177574,0.324857686560062,
4.98221854910706));
#26173=CARTESIAN_POINT('Ctrl Pts',(-34.6593774847591,-0.518476572724812,
4.96580469119751));
#26174=CARTESIAN_POINT('Ctrl Pts',(-34.6197411517608,-1.30665709549724,
4.74893905870966));
#26175=CARTESIAN_POINT('Ctrl Pts',(-34.5801048187625,-2.0948376182697,4.5320734262218));
#26176=CARTESIAN_POINT('Ctrl Pts',(-34.5404684857642,-2.8278644045297,4.11475601915564));
#26177=CARTESIAN_POINT('Ctrl Pts',(-34.5008321527658,-3.41667405734504,
3.54769126819355));
#26178=CARTESIAN_POINT('Ctrl Pts',(-34.4611958197675,-4.00548371016042,
2.98062651723144));
#26179=CARTESIAN_POINT('Ctrl Pts',(-34.4215594867692,-4.45007622953113,
2.26381442237339));
#26180=CARTESIAN_POINT('Ctrl Pts',(-34.3819231537709,-4.69643323472671,
1.48434828133623));
#26181=CARTESIAN_POINT('Ctrl Pts',(-34.3575626111485,-4.84784457557038,
1.00528736133934));
#26182=CARTESIAN_POINT('Ctrl Pts',(-34.333202068526,-4.92437546731788,0.502559828752335));
#26183=CARTESIAN_POINT('Ctrl Pts',(-34.3088415259036,-4.92466853775765,
-8.04693041996219E-5));
#26184=CARTESIAN_POINT('Origin',(-41.25,0.,0.));
#26185=CARTESIAN_POINT('',(-32.5911584740964,-4.92505699337764,0.000124540890476602));
#26186=CARTESIAN_POINT('',(-32.8088415259036,-4.92500432546286,0.000126715614278523));
#26187=CARTESIAN_POINT('',(-41.25,-4.925,-6.03138548580071E-16));
#26188=CARTESIAN_POINT('Ctrl Pts',(-32.5911584740964,-4.92505699337764,
0.000124540890476602));
#26189=CARTESIAN_POINT('Ctrl Pts',(-32.599438308694,-4.92523260524548,0.170926811184958));
#26190=CARTESIAN_POINT('Ctrl Pts',(-32.6077181432915,-4.9165200525162,0.341711253364765));
#26191=CARTESIAN_POINT('Ctrl Pts',(-32.6159979778891,-4.89878435312716,
0.51155345732391));
#26192=CARTESIAN_POINT('Ctrl Pts',(-32.6556343108875,-4.81388192196659,
1.32460377541339));
#26193=CARTESIAN_POINT('Ctrl Pts',(-32.6952706438858,-4.52220277615496,
2.11606152374493));
#26194=CARTESIAN_POINT('Ctrl Pts',(-32.7349069768841,-4.05918618745925,
2.78976389216296));
#26195=CARTESIAN_POINT('Ctrl Pts',(-32.7745433098825,-3.59616959876357,
3.46346626058094));
#26196=CARTESIAN_POINT('Ctrl Pts',(-32.8141796428808,-2.96181556718383,
4.01941324908544));
#26197=CARTESIAN_POINT('Ctrl Pts',(-32.8538159758791,-2.23319866351874,
4.39005681142113));
#26198=CARTESIAN_POINT('Ctrl Pts',(-32.8934523088774,-1.50458175985363,
4.76070037375683));
#26199=CARTESIAN_POINT('Ctrl Pts',(-32.9330886418757,-0.681701984103161,
4.94604050992373));
#26200=CARTESIAN_POINT('Ctrl Pts',(-32.972724974874,0.135460049849992,4.92355823091998));
#26201=CARTESIAN_POINT('Ctrl Pts',(-33.0123613078724,0.952622083803168,
4.90107595191623));
#26202=CARTESIAN_POINT('Ctrl Pts',(-33.0519976408707,1.76406637595904,4.67077125774183));
#26203=CARTESIAN_POINT('Ctrl Pts',(-33.091633973869,2.4712017336879,4.26062637058644));
#26204=CARTESIAN_POINT('Ctrl Pts',(-33.1312703068673,3.17833709141674,3.85048148343106));
#26205=CARTESIAN_POINT('Ctrl Pts',(-33.1709066398656,3.78116351471858,3.26049640329468));
#26206=CARTESIAN_POINT('Ctrl Pts',(-33.210542972864,4.20643706486838,2.56235483445041));
#26207=CARTESIAN_POINT('Ctrl Pts',(-33.2501793058623,4.63171061501819,1.86421326560614));
#26208=CARTESIAN_POINT('Ctrl Pts',(-33.2898156388606,4.87943129201598,1.05791520805396));
#26209=CARTESIAN_POINT('Ctrl Pts',(-33.3294519718589,4.91950081650975,0.241426582404654));
#26210=CARTESIAN_POINT('Ctrl Pts',(-33.3690883048572,4.95957034100353,-0.575062043244695));
#26211=CARTESIAN_POINT('Ctrl Pts',(-33.4087246378556,4.7919887129933,-1.40174123699112));
#26212=CARTESIAN_POINT('Ctrl Pts',(-33.4483609708539,4.43711724714662,-2.13816875232085));
#26213=CARTESIAN_POINT('Ctrl Pts',(-33.4879973038522,4.08224578129997,-2.87459626765054));
#26214=CARTESIAN_POINT('Ctrl Pts',(-33.5276336368505,3.54008447761688,-3.5207721045635));
#26215=CARTESIAN_POINT('Ctrl Pts',(-33.5672699698489,2.87650640962745,-3.99818533258564));
#26216=CARTESIAN_POINT('Ctrl Pts',(-33.6069063028472,2.21292834163802,-4.47559856060777));
#26217=CARTESIAN_POINT('Ctrl Pts',(-33.6465426358455,1.42793350934223,-4.78424917973909));
#26218=CARTESIAN_POINT('Ctrl Pts',(-33.6861789688438,0.616899472809076,
-4.88663586926392));
#26219=CARTESIAN_POINT('Ctrl Pts',(-33.7258153018421,-0.194134563724077,
-4.98902255878875));
#26220=CARTESIAN_POINT('Ctrl Pts',(-33.7654516348405,-1.0312078044946,-4.8851453187071));
#26221=CARTESIAN_POINT('Ctrl Pts',(-33.8050879678388,-1.79261511716435,
-4.5876253247234));
#26222=CARTESIAN_POINT('Ctrl Pts',(-33.8447243008371,-2.5540224298341,-4.29010533073969));
#26223=CARTESIAN_POINT('Ctrl Pts',(-33.8843606338354,-3.23976381440308,
-3.79894258285393));
#26224=CARTESIAN_POINT('Ctrl Pts',(-33.9239969668337,-3.76652109168392,
-3.17381378537394));
#26225=CARTESIAN_POINT('Ctrl Pts',(-33.963633299832,-4.29327836896475,-2.54868498789394));
#26226=CARTESIAN_POINT('Ctrl Pts',(-34.0032696328304,-4.66105153895743,
-1.7895901408197));
#26227=CARTESIAN_POINT('Ctrl Pts',(-34.0429059658287,-4.82515583920305,
-0.988759933317539));
#26228=CARTESIAN_POINT('Ctrl Pts',(-34.0589901352513,-4.89174831051554,
-0.663788177309668));
#26229=CARTESIAN_POINT('Ctrl Pts',(-34.0750743046738,-4.92480294907351,
-0.331943925079275));
#26230=CARTESIAN_POINT('Ctrl Pts',(-34.0911584740964,-4.92464097398149,
-6.78464643288912E-5));
#26231=CARTESIAN_POINT('Ctrl Pts',(-34.3088415259036,-4.92466853775765,
-8.04693041996219E-5));
#26232=CARTESIAN_POINT('Ctrl Pts',(-34.2935657355277,-4.92485231373804,
-0.315271635058983));
#26233=CARTESIAN_POINT('Ctrl Pts',(-34.2782899451518,-4.89505800095221,
-0.630428498620279));
#26234=CARTESIAN_POINT('Ctrl Pts',(-34.2630141547759,-4.834950904457,-0.939693939557906));
#26235=CARTESIAN_POINT('Ctrl Pts',(-34.2233778217776,-4.67899007797124,
-1.74214983219882));
#26236=CARTESIAN_POINT('Ctrl Pts',(-34.1837414887793,-4.31894693397922,
-2.50494143026443));
#26237=CARTESIAN_POINT('Ctrl Pts',(-34.144105155781,-3.79856703000646,-3.13538888610318));
#26238=CARTESIAN_POINT('Ctrl Pts',(-34.1044688227826,-3.27818712603374,
-3.76583634194189));
#26239=CARTESIAN_POINT('Ctrl Pts',(-34.0648324897843,-2.59747046208028,
-4.26393965555378));
#26240=CARTESIAN_POINT('Ctrl Pts',(-34.025196156786,-1.83912470937512,-4.56917883781291));
#26241=CARTESIAN_POINT('Ctrl Pts',(-33.9855598237877,-1.0807789566699,-4.87441802007206));
#26242=CARTESIAN_POINT('Ctrl Pts',(-33.9459234907894,-0.24480411521302,
-4.98679307097843));
#26243=CARTESIAN_POINT('Ctrl Pts',(-33.906287157791,0.567228139136565,-4.89265032336495));
#26244=CARTESIAN_POINT('Ctrl Pts',(-33.8666508247927,1.3792603934861,-4.79850757575147));
#26245=CARTESIAN_POINT('Ctrl Pts',(-33.8270144917944,2.16735006072829,-4.49784702961813));
#26246=CARTESIAN_POINT('Ctrl Pts',(-33.7873781587961,2.83574355563621,-4.02719920480961));
#26247=CARTESIAN_POINT('Ctrl Pts',(-33.7477418257978,3.50413705054412,-3.55655138000108));
#26248=CARTESIAN_POINT('Ctrl Pts',(-33.7081054927994,4.05283437311776,-2.91591627651736));
#26249=CARTESIAN_POINT('Ctrl Pts',(-33.6684691598011,4.41516831780336,-2.18313162086415));
#26250=CARTESIAN_POINT('Ctrl Pts',(-33.6288328268028,4.77750226248896,-1.45034696521094));
#26251=CARTESIAN_POINT('Ctrl Pts',(-33.5891964938045,4.95347282928651,-0.625412757388233));
#26252=CARTESIAN_POINT('Ctrl Pts',(-33.5495601608062,4.92169944011505,0.191440773407072));
#26253=CARTESIAN_POINT('Ctrl Pts',(-33.5099238278078,4.88992605094358,1.00829430420238));
#26254=CARTESIAN_POINT('Ctrl Pts',(-33.4702874948095,4.65040870580311,1.8170671579703));
#26255=CARTESIAN_POINT('Ctrl Pts',(-33.4306511618112,4.23224897203365,2.519492724195));
#26256=CARTESIAN_POINT('Ctrl Pts',(-33.3910148288129,3.81408923826417,3.22191829041972));
#26257=CARTESIAN_POINT('Ctrl Pts',(-33.3513784958145,3.21728711586574,3.81799656910118));
#26258=CARTESIAN_POINT('Ctrl Pts',(-33.3117421628162,2.51435458572833,4.23530352699527));
#26259=CARTESIAN_POINT('Ctrl Pts',(-33.2721058298179,1.81142205559096,4.65261048488934));
#26260=CARTESIAN_POINT('Ctrl Pts',(-33.2324694968196,1.00235911771458,4.89114612199604));
#26261=CARTESIAN_POINT('Ctrl Pts',(-33.1928331638213,0.185467628088543,
4.921928149362));
#26262=CARTESIAN_POINT('Ctrl Pts',(-33.153196830823,-0.631423861537568,
4.95271017672796));
#26263=CARTESIAN_POINT('Ctrl Pts',(-33.1135604978246,-1.45614390291336,
4.77573859435319));
#26264=CARTESIAN_POINT('Ctrl Pts',(-33.0739241648263,-2.1884882882529,4.412515604588));
#26265=CARTESIAN_POINT('Ctrl Pts',(-33.034287831828,-2.9208326735924,4.04929261482283));
#26266=CARTESIAN_POINT('Ctrl Pts',(-32.9946514988297,-3.5608014028956,3.49981821766725));
#26267=CARTESIAN_POINT('Ctrl Pts',(-32.9550151658314,-4.03063771470406,
2.83085403391884));
#26268=CARTESIAN_POINT('Ctrl Pts',(-32.915378832833,-4.50047402651251,2.16188985017043));
#26269=CARTESIAN_POINT('Ctrl Pts',(-32.8757424998347,-4.80017792082623,
1.37343587982916));
#26270=CARTESIAN_POINT('Ctrl Pts',(-32.8361061668364,-4.89333511183429,
0.561289971265626));
#26271=CARTESIAN_POINT('Ctrl Pts',(-32.8270179531921,-4.91469512146023,
0.375073059432364));
#26272=CARTESIAN_POINT('Ctrl Pts',(-32.8179297395479,-4.92519616725995,
0.187610570225986));
#26273=CARTESIAN_POINT('Ctrl Pts',(-32.8088415259036,-4.92500432546286,
0.000126715614278523));
#26274=CARTESIAN_POINT('Origin',(-41.25,0.,0.));
#26275=CARTESIAN_POINT('',(-31.0911584740964,-4.92514031288301,-0.000116505347877993));
#26276=CARTESIAN_POINT('',(-31.3088415259036,-4.9251906134473,-0.000109311167407344));
#26277=CARTESIAN_POINT('',(-41.25,-4.925,-6.03138548580071E-16));
#26278=CARTESIAN_POINT('Ctrl Pts',(-31.0911584740964,-4.92514031288301,
-0.000116505347877993));
#26279=CARTESIAN_POINT('Ctrl Pts',(-31.1238023127141,-4.92446467357143,
0.673250866068188));
#26280=CARTESIAN_POINT('Ctrl Pts',(-31.1564461513319,-4.78528366208081,
1.34688857869454));
#26281=CARTESIAN_POINT('Ctrl Pts',(-31.1890899899496,-4.51678499905435,
1.9642879928124));
#26282=CARTESIAN_POINT('Ctrl Pts',(-31.2287263229479,-4.19077240776744,
2.71393784427457));
#26283=CARTESIAN_POINT('Ctrl Pts',(-31.2683626559462,-3.67410740557199,
3.38067583437288));
#26284=CARTESIAN_POINT('Ctrl Pts',(-31.3079989889446,-3.02956497379938,
3.8834922164745));
#26285=CARTESIAN_POINT('Ctrl Pts',(-31.3476353219429,-2.38502254202674,
4.38630859857615));
#26286=CARTESIAN_POINT('Ctrl Pts',(-31.3872716549412,-1.61260268067694,
4.72520337268107));
#26287=CARTESIAN_POINT('Ctrl Pts',(-31.4269079879395,-0.806155214751121,
4.85900077557536));
#26288=CARTESIAN_POINT('Ctrl Pts',(-31.4665443209379,0.000292251174648372,
4.99279817846964));
#26289=CARTESIAN_POINT('Ctrl Pts',(-31.5061806539362,0.840767321676489,
4.9214982101533));
#26290=CARTESIAN_POINT('Ctrl Pts',(-31.5458169869345,1.61315160673935,4.65376375455655));
#26291=CARTESIAN_POINT('Ctrl Pts',(-31.5854533199328,2.38553589180226,4.38602929895978));
#26292=CARTESIAN_POINT('Ctrl Pts',(-31.6250896529312,3.0898293914262,3.92186035608262));
#26293=CARTESIAN_POINT('Ctrl Pts',(-31.6647259859295,3.64045979429983,3.3176539217641));
#26294=CARTESIAN_POINT('Ctrl Pts',(-31.7043623189278,4.19109019717344,2.71344748744561));
#26295=CARTESIAN_POINT('Ctrl Pts',(-31.7439986519261,4.58805750329668,1.96920356168581));
#26296=CARTESIAN_POINT('Ctrl Pts',(-31.7836349849244,4.78312985406825,1.17534840237615));
#26297=CARTESIAN_POINT('Ctrl Pts',(-31.8232713179227,4.97820220483983,0.381493243066466));
#26298=CARTESIAN_POINT('Ctrl Pts',(-31.8629076509211,4.97137960025971,-0.461973149793131));
#26299=CARTESIAN_POINT('Ctrl Pts',(-31.9025439839194,4.76349098425275,-1.25256885458638));
#26300=CARTESIAN_POINT('Ctrl Pts',(-31.9421803169177,4.55560236824579,-2.0431645593796));
#26301=CARTESIAN_POINT('Ctrl Pts',(-31.981816649916,4.14664774081201,-2.78088957610653));
#26302=CARTESIAN_POINT('Ctrl Pts',(-32.0214529829143,3.58631545184477,-3.37610967658211));
#26303=CARTESIAN_POINT('Ctrl Pts',(-32.0610893159127,3.02598316287755,-3.97132977705768));
#26304=CARTESIAN_POINT('Ctrl Pts',(-32.100725648911,2.31427321237688,-4.42404496128188));
#26305=CARTESIAN_POINT('Ctrl Pts',(-32.1403619819093,1.53765898091128,-4.67924993368397));
#26306=CARTESIAN_POINT('Ctrl Pts',(-32.1799983149076,0.761044749445631,
-4.93445490608606));
#26307=CARTESIAN_POINT('Ctrl Pts',(-32.219634647906,-0.0804737629849417,
-4.992149666666));
#26308=CARTESIAN_POINT('Ctrl Pts',(-32.2592709809043,-0.884651318568558,
-4.8453242534271));
#26309=CARTESIAN_POINT('Ctrl Pts',(-32.2989073139026,-1.68882887415215,
-4.6984988401882));
#26310=CARTESIAN_POINT('Ctrl Pts',(-32.3385436469009,-2.45566547288878,
-4.34715325313046));
#26311=CARTESIAN_POINT('Ctrl Pts',(-32.3781799798992,-3.09198979653732,
-3.83397628799953));
#26312=CARTESIAN_POINT('Ctrl Pts',(-32.4178163128975,-3.72831412018587,
-3.32079932286859));
#26313=CARTESIAN_POINT('Ctrl Pts',(-32.4574526458959,-4.23412616874633,
-2.64579097966446));
#26314=CARTESIAN_POINT('Ctrl Pts',(-32.4970889788942,-4.54796933477179,
-1.8909653641387));
#26315=CARTESIAN_POINT('Ctrl Pts',(-32.5284454772949,-4.79625221033389,
-1.29381909919356));
#26316=CARTESIAN_POINT('Ctrl Pts',(-32.5598019756957,-4.92439193501344,
-0.646719433129764));
#26317=CARTESIAN_POINT('Ctrl Pts',(-32.5911584740964,-4.92505699337764,
0.000124540890476602));
#26318=CARTESIAN_POINT('Ctrl Pts',(-32.8088415259036,-4.92500432546286,
0.000126715614278523));
#26319=CARTESIAN_POINT('Ctrl Pts',(-32.7782934065495,-4.92435948959698,
-0.630060842889056));
#26320=CARTESIAN_POINT('Ctrl Pts',(-32.7477452871955,-4.80290353570356,
-1.26048979348428));
#26321=CARTESIAN_POINT('Ctrl Pts',(-32.7171971678414,-4.56694350005811,
-1.84466853820109));
#26322=CARTESIAN_POINT('Ctrl Pts',(-32.6775608348431,-4.26078420957148,
-2.60264329231841));
#26323=CARTESIAN_POINT('Ctrl Pts',(-32.6379245018448,-3.76185514089583,
-3.28275495376725));
#26324=CARTESIAN_POINT('Ctrl Pts',(-32.5982881688465,-3.13077661311804,
-3.80236935966164));
#26325=CARTESIAN_POINT('Ctrl Pts',(-32.5586518358481,-2.49969808534025,
-4.32198376555603));
#26326=CARTESIAN_POINT('Ctrl Pts',(-32.5190155028498,-1.73647009846033,
-4.68110091589597));
#26327=CARTESIAN_POINT('Ctrl Pts',(-32.4793791698515,-0.933825521759056,
-4.83608776217916));
#26328=CARTESIAN_POINT('Ctrl Pts',(-32.4397428368532,-0.131180945057805,
-4.99107460846236));
#26329=CARTESIAN_POINT('Ctrl Pts',(-32.4001065038549,0.710880221464788,
-4.94193115068882));
#26330=CARTESIAN_POINT('Ctrl Pts',(-32.3604701708565,1.49004680813205,-4.69462836207976));
#26331=CARTESIAN_POINT('Ctrl Pts',(-32.3208338378582,2.26921339479935,-4.44732557347068));
#26332=CARTESIAN_POINT('Ctrl Pts',(-32.2811975048599,2.98548540161131,-4.00186345402606));
#26333=CARTESIAN_POINT('Ctrl Pts',(-32.2415611718616,3.55183515199862,-3.4123660415797));
#26334=CARTESIAN_POINT('Ctrl Pts',(-32.2019248388633,4.11818490238593,-2.82286862913336));
#26335=CARTESIAN_POINT('Ctrl Pts',(-32.1622885058649,4.53461239634859,-2.08933592368529));
#26336=CARTESIAN_POINT('Ctrl Pts',(-32.1226521728666,4.75052132847285,-1.30089279192747));
#26337=CARTESIAN_POINT('Ctrl Pts',(-32.0830158398683,4.96643026059711,-0.512449660169646));
#26338=CARTESIAN_POINT('Ctrl Pts',(-32.04337950687,4.98182063088296,0.330903897897914));
#26339=CARTESIAN_POINT('Ctrl Pts',(-32.0037431738717,4.79482249575999,1.12669968615089));
#26340=CARTESIAN_POINT('Ctrl Pts',(-31.9641068408733,4.60782436063702,1.92249547440389));
#26341=CARTESIAN_POINT('Ctrl Pts',(-31.924470507875,4.21843772010518,2.67073349284236));
#26342=CARTESIAN_POINT('Ctrl Pts',(-31.8848341748767,3.67397339242095,3.28050216595624));
#26343=CARTESIAN_POINT('Ctrl Pts',(-31.8451978418784,3.12950906473676,3.89027083907008));
#26344=CARTESIAN_POINT('Ctrl Pts',(-31.8055615088801,2.42996704990017,4.36157016685941));
#26345=CARTESIAN_POINT('Ctrl Pts',(-31.7659251758817,1.66034231540023,4.63713686903792));
#26346=CARTESIAN_POINT('Ctrl Pts',(-31.7262888428834,0.890717580900255,
4.91270357121643));
#26347=CARTESIAN_POINT('Ctrl Pts',(-31.6866525098851,0.0510101267369292,
4.99253764778412));
#26348=CARTESIAN_POINT('Ctrl Pts',(-31.6470161768868,-0.756754854777219,
4.86693918633553));
#26349=CARTESIAN_POINT('Ctrl Pts',(-31.6073798438884,-1.56451983629139,
4.74134072488694));
#26350=CARTESIAN_POINT('Ctrl Pts',(-31.5677435108901,-2.34034234515637,
4.41030972542208));
#26351=CARTESIAN_POINT('Ctrl Pts',(-31.5281071778918,-2.98995926811177,
3.91406674874667));
#26352=CARTESIAN_POINT('Ctrl Pts',(-31.4884708448935,-3.63957619106713,
3.41782377207128));
#26353=CARTESIAN_POINT('Ctrl Pts',(-31.4488345118952,-4.16298752811293,
2.75636881818537));
#26354=CARTESIAN_POINT('Ctrl Pts',(-31.4091981788969,-4.49659834015827,
2.01006923515549));
#26355=CARTESIAN_POINT('Ctrl Pts',(-31.3757459612324,-4.77815873325062,
1.38020834223579));
#26356=CARTESIAN_POINT('Ctrl Pts',(-31.342293743568,-4.92452422896182,0.689912627386944));
#26357=CARTESIAN_POINT('Ctrl Pts',(-31.3088415259036,-4.9251906134473,-0.000109311167407344));
#26358=CARTESIAN_POINT('Origin',(-55.3478126690739,0.,0.));
#26359=CARTESIAN_POINT('',(-30.5978126690739,-4.07061596824169,-9.62913744964106E-5));
#26360=CARTESIAN_POINT('',(-30.3021873309261,-4.0701702520628,4.41716588962804E-5));
#26361=CARTESIAN_POINT('',(-55.3478126690739,-4.0705,-3.42898509504556E-13));
#26362=CARTESIAN_POINT('',(-30.,3.27123863458584,-2.42269058837956));
#26363=CARTESIAN_POINT('Ctrl Pts',(-30.5978126690739,-4.07061596824169,
-9.62913744964253E-5));
#26364=CARTESIAN_POINT('Ctrl Pts',(-30.5908201746933,-4.07073558370832,
-0.119309532774532));
#26365=CARTESIAN_POINT('Ctrl Pts',(-30.5441913473144,-4.03650708564677,
-0.914204073344773));
#26366=CARTESIAN_POINT('Ctrl Pts',(-30.4579261869372,-3.53493172767287,
-2.34618303071339));
#26367=CARTESIAN_POINT('Ctrl Pts',(-30.3390171879422,-1.98456278272466,
-3.74990799775467));
#26368=CARTESIAN_POINT('Ctrl Pts',(-30.2201081889473,0.0480654627907762,
-4.24241178043034));
#26369=CARTESIAN_POINT('Ctrl Pts',(-30.1071024596332,1.96866978992971,-3.73070684879719));
#26370=CARTESIAN_POINT('Ctrl Pts',(-30.0337330633174,2.92852673884923,-2.88450283314551));
#26371=CARTESIAN_POINT('Ctrl Pts',(-30.,3.27123863458584,-2.42269058837956));
#26372=CARTESIAN_POINT('',(-30.,-1.22233170237264,-3.88263769354994));
#26373=CARTESIAN_POINT('Origin',(-30.,0.,0.));
#26374=CARTESIAN_POINT('Ctrl Pts',(-30.3021873309261,-4.0701702520628,4.41716588963498E-5));
#26375=CARTESIAN_POINT('Ctrl Pts',(-30.280730886614,-4.07009405811129,-0.365864875771756));
#26376=CARTESIAN_POINT('Ctrl Pts',(-30.2196381093036,-3.93089507694675,
-1.40778857362903));
#26377=CARTESIAN_POINT('Ctrl Pts',(-30.118908998995,-3.05253333388674,-2.94673281729211));
#26378=CARTESIAN_POINT('Ctrl Pts',(-30.0396363329983,-1.86695937376294,
-3.67969605923881));
#26379=CARTESIAN_POINT('Ctrl Pts',(-30.,-1.22233170237264,-3.88263769354994));
#26380=CARTESIAN_POINT('Origin',(-55.3478126690739,0.,0.));
#26381=CARTESIAN_POINT('',(-32.0978126690739,-4.07054710488196,0.0001029327297676));
#26382=CARTESIAN_POINT('',(-31.8021873309261,-4.07065754153041,-9.03454027129102E-5));
#26383=CARTESIAN_POINT('',(-55.3478126690739,-4.0705,-3.42898509504556E-13));
#26384=CARTESIAN_POINT('Ctrl Pts',(-32.0978126690739,-4.07054710488196,
0.000102932729767729));
#26385=CARTESIAN_POINT('Ctrl Pts',(-32.0664561706731,-4.0699974358319,-0.534511970061966));
#26386=CARTESIAN_POINT('Ctrl Pts',(-31.9954633392741,-3.83021782586463,
-1.74538787858084));
#26387=CARTESIAN_POINT('Ctrl Pts',(-31.8848341748767,-2.66338978325909,
-3.30252489436533));
#26388=CARTESIAN_POINT('Ctrl Pts',(-31.7659251758817,-0.762024275548931,
-4.17368360225475));
#26389=CARTESIAN_POINT('Ctrl Pts',(-31.6470161768868,1.32451446852128,-4.03062988269698));
#26390=CARTESIAN_POINT('Ctrl Pts',(-31.5281071778918,3.08919387167645,-2.90812603048288));
#26391=CARTESIAN_POINT('Ctrl Pts',(-31.4091981788968,4.10319375653073,-1.07894246870398));
#26392=CARTESIAN_POINT('Ctrl Pts',(-31.2902891799019,4.12011035263834,1.01242603005823));
#26393=CARTESIAN_POINT('Ctrl Pts',(-31.1713801809069,3.13583293969945,2.85777317714776));
#26394=CARTESIAN_POINT('Ctrl Pts',(-31.0524711819119,1.38954257002262,4.00867653673046));
#26395=CARTESIAN_POINT('Ctrl Pts',(-30.933562182917,-0.694408967730227,
4.18546426527762));
#26396=CARTESIAN_POINT('Ctrl Pts',(-30.8146531839221,-2.6096181325775,3.34517725330154));
#26397=CARTESIAN_POINT('Ctrl Pts',(-30.7027366793076,-3.81535138401945,
1.78922095425846));
#26398=CARTESIAN_POINT('Ctrl Pts',(-30.6304565076916,-4.07005755406551,
0.556440132046678));
#26399=CARTESIAN_POINT('Ctrl Pts',(-30.5978126690739,-4.07061596824169,
-9.62913744964253E-5));
#26400=CARTESIAN_POINT('Ctrl Pts',(-31.8021873309261,-4.07065754153041,
-9.0345402713049E-5));
#26401=CARTESIAN_POINT('Ctrl Pts',(-31.7960032155922,-4.07075935824244,
-0.105518617748798));
#26402=CARTESIAN_POINT('Ctrl Pts',(-31.75018276726,-4.04102178465253,-0.88661924731187));
#26403=CARTESIAN_POINT('Ctrl Pts',(-31.6647259859294,-3.55858318971203,
-2.31015180080996));
#26404=CARTESIAN_POINT('Ctrl Pts',(-31.5458169869345,-2.02255110907419,
-3.72955802299772));
#26405=CARTESIAN_POINT('Ctrl Pts',(-31.4269079879395,0.00496435902457082,
-4.24267488557468));
#26406=CARTESIAN_POINT('Ctrl Pts',(-31.3079989889446,2.03127363286532,-3.72481475967269));
#26407=CARTESIAN_POINT('Ctrl Pts',(-31.1890899899496,3.56397954706214,-2.30181723085673));
#26408=CARTESIAN_POINT('Ctrl Pts',(-31.0701809909547,4.23063279613937,-0.319475851207252));
#26409=CARTESIAN_POINT('Ctrl Pts',(-30.9512719919596,3.86923364069296,1.74050225247754));
#26410=CARTESIAN_POINT('Ctrl Pts',(-30.8323629929648,2.56760636218215,3.37752821215737));
#26411=CARTESIAN_POINT('Ctrl Pts',(-30.7134539939697,0.642041383293453,
4.19382295160038));
#26412=CARTESIAN_POINT('Ctrl Pts',(-30.5945449949749,-1.43953109436157,
3.99098332553759));
#26413=CARTESIAN_POINT('Ctrl Pts',(-30.4756359959798,-3.17131430799793,
2.8183836925229));
#26414=CARTESIAN_POINT('Ctrl Pts',(-30.378183441297,-3.9589973334931,1.29599045009805));
#26415=CARTESIAN_POINT('Ctrl Pts',(-30.3203672196124,-4.07023481064188,
0.310076237309551));
#26416=CARTESIAN_POINT('Ctrl Pts',(-30.3021873309261,-4.0701702520628,4.41716588963498E-5));
#26417=CARTESIAN_POINT('Origin',(-55.3478126690739,0.,0.));
#26418=CARTESIAN_POINT('',(-33.5978126690739,-4.07020326590693,-5.60749306866135E-5));
#26419=CARTESIAN_POINT('',(-33.3021873309261,-4.07050357498408,0.000104730133066722));
#26420=CARTESIAN_POINT('',(-55.3478126690739,-4.0705,-3.42898509504556E-13));
#26421=CARTESIAN_POINT('Ctrl Pts',(-33.5978126690739,-4.07020326590693,
-5.60749306863922E-5));
#26422=CARTESIAN_POINT('Ctrl Pts',(-33.5817284996513,-4.07033713790938,
-0.274350811580848));
#26423=CARTESIAN_POINT('Ctrl Pts',(-33.5260079972304,-3.97569374054994,
-1.22450089022107));
#26424=CARTESIAN_POINT('Ctrl Pts',(-33.4306511618112,-3.24442008373921,
-2.73387163822095));
#26425=CARTESIAN_POINT('Ctrl Pts',(-33.3117421628162,-1.5441295420815,-3.95170593178579));
#26426=CARTESIAN_POINT('Ctrl Pts',(-33.1928331638213,0.531387184754894,
-4.20926875762475));
#26427=CARTESIAN_POINT('Ctrl Pts',(-33.0739241648263,2.47777589431427,-3.44397189762026));
#26428=CARTESIAN_POINT('Ctrl Pts',(-32.9550151658313,3.82206071866471,-1.84178383011512));
#26429=CARTESIAN_POINT('Ctrl Pts',(-32.8361061668364,4.23757808931381,0.207960936267553));
#26430=CARTESIAN_POINT('Ctrl Pts',(-32.7171971678414,3.62335655689582,2.20717083064289));
#26431=CARTESIAN_POINT('Ctrl Pts',(-32.5982881688465,2.12865303036779,3.67003434456881));
#26432=CARTESIAN_POINT('Ctrl Pts',(-32.4793791698515,0.116683086477182,
4.24107308018517));
#26433=CARTESIAN_POINT('Ctrl Pts',(-32.3604701708566,-1.92364105191405,
3.78152362377861));
#26434=CARTESIAN_POINT('Ctrl Pts',(-32.2415611718616,-3.49651704310921,
2.40305729888056));
#26435=CARTESIAN_POINT('Ctrl Pts',(-32.1540086712673,-4.0290199584954,0.95813549201353));
#26436=CARTESIAN_POINT('Ctrl Pts',(-32.1060925036714,-4.07069224764503,
0.141270575619876));
#26437=CARTESIAN_POINT('Ctrl Pts',(-32.0978126690739,-4.07054710488196,
0.000102932729767729));
#26438=CARTESIAN_POINT('Ctrl Pts',(-33.3021873309261,-4.07050357498408,
0.00010473013306686));
#26439=CARTESIAN_POINT('Ctrl Pts',(-33.2716392115721,-4.0699706197775,-0.520743687508975));
#26440=CARTESIAN_POINT('Ctrl Pts',(-33.2014547592197,-3.83934010403903,
-1.71785382786294));
#26441=CARTESIAN_POINT('Ctrl Pts',(-33.091633973869,-2.69680011715167,-3.27529919943904));
#26442=CARTESIAN_POINT('Ctrl Pts',(-32.9727249748741,-0.804382135063499,
-4.16572743931235));
#26443=CARTESIAN_POINT('Ctrl Pts',(-32.853815975879,1.28350211569609,-4.04387660995158));
#26444=CARTESIAN_POINT('Ctrl Pts',(-32.7349069768842,3.05949310273849,-2.93935667663218));
#26445=CARTESIAN_POINT('Ctrl Pts',(-32.6159979778891,4.09202190325118,-1.12056791874808));
#26446=CARTESIAN_POINT('Ctrl Pts',(-32.4970889788942,4.13018220918936,0.970520807006677));
#26447=CARTESIAN_POINT('Ctrl Pts',(-32.3781799798992,3.16470099886364,2.82577127648086));
#26448=CARTESIAN_POINT('Ctrl Pts',(-32.2592709809043,1.43019189953828,3.99435437116099));
#26449=CARTESIAN_POINT('Ctrl Pts',(-32.1403619819093,-0.651856339348117,
4.19230235613684));
#26450=CARTESIAN_POINT('Ctrl Pts',(-32.0214529829143,-2.57550234280079,
3.37151351350433));
#26451=CARTESIAN_POINT('Ctrl Pts',(-31.9087280992533,-3.80580220902221,
1.8167364506488));
#26452=CARTESIAN_POINT('Ctrl Pts',(-31.8356395485905,-4.07010677644452,
0.570211035487816));
#26453=CARTESIAN_POINT('Ctrl Pts',(-31.8021873309261,-4.07065754153041,
-9.0345402713049E-5));
#26454=CARTESIAN_POINT('Origin',(-55.3478126690739,0.,0.));
#26455=CARTESIAN_POINT('',(-35.0978126690738,-4.07084382520696,-1.45670438658383E-5));
#26456=CARTESIAN_POINT('',(-34.8021873309261,-4.07022604729798,-6.65076760328343E-5));
#26457=CARTESIAN_POINT('',(-55.3478126690739,-4.0705,-3.42898509504556E-13));
#26458=CARTESIAN_POINT('Ctrl Pts',(-35.0978126690738,-4.07084382520696,
-1.45670438656941E-5));
#26459=CARTESIAN_POINT('Ctrl Pts',(-35.0970008286294,-4.07084664099177,
-0.0138531808912899));
#26460=CARTESIAN_POINT('Ctrl Pts',(-35.0565526551867,-4.0674041557348,-0.703330423914037));
#26461=CARTESIAN_POINT('Ctrl Pts',(-34.9764681487457,-3.70631687576659,
-2.06483196179423));
#26462=CARTESIAN_POINT('Ctrl Pts',(-34.8575591497507,-2.26953513242235,
-3.58462356416123));
#26463=CARTESIAN_POINT('Ctrl Pts',(-34.7386501507558,-0.281252374001066,
-4.2333453575344));
#26464=CARTESIAN_POINT('Ctrl Pts',(-34.6197411517608,1.77537520426393,-3.8533568090853));
#26465=CARTESIAN_POINT('Ctrl Pts',(-34.5008321527659,3.40058349612684,-2.5369958021071));
#26466=CARTESIAN_POINT('Ctrl Pts',(-34.3819231537709,4.19944403810212,-0.604140368530221));
#26467=CARTESIAN_POINT('Ctrl Pts',(-34.2630141547759,3.97783231829727,1.47552223349874));
#26468=CARTESIAN_POINT('Ctrl Pts',(-34.144105155781,2.78960037305193,3.19663034658495));
#26469=CARTESIAN_POINT('Ctrl Pts',(-34.025196156786,0.92349064771896,4.14095168259845));
#26470=CARTESIAN_POINT('Ctrl Pts',(-33.9062871577911,-1.16702892364603,
4.07901450174094));
#26471=CARTESIAN_POINT('Ctrl Pts',(-33.7873781587961,-2.97395842107017,
3.02586964752038));
#26472=CARTESIAN_POINT('Ctrl Pts',(-33.6845533292237,-3.9115499238755,1.47934517898094));
#26473=CARTESIAN_POINT('Ctrl Pts',(-33.6213648326496,-4.07000723618249,
0.401595657019318));
#26474=CARTESIAN_POINT('Ctrl Pts',(-33.5978126690739,-4.07020326590693,
-5.60749306863922E-5));
#26475=CARTESIAN_POINT('Ctrl Pts',(-34.8021873309261,-4.07022604729797,
-6.65076760328689E-5));
#26476=CARTESIAN_POINT('Ctrl Pts',(-34.7869115405502,-4.07037793767931,
-0.260571206194689));
#26477=CARTESIAN_POINT('Ctrl Pts',(-34.731999417176,-3.98185833732723,-1.19690962121964));
#26478=CARTESIAN_POINT('Ctrl Pts',(-34.6374509608035,-3.27202393444525,
-2.70077305417611));
#26479=CARTESIAN_POINT('Ctrl Pts',(-34.5185419618086,-1.5841921492944,-3.93581642761199));
#26480=CARTESIAN_POINT('Ctrl Pts',(-34.3996329628135,0.488601104807327,
-4.21444951068671));
#26481=CARTESIAN_POINT('Ctrl Pts',(-34.2807239638187,2.44266343405159,-3.46896397584259));
#26482=CARTESIAN_POINT('Ctrl Pts',(-34.1618149648236,3.80315426747452,-1.88051411468693));
#26483=CARTESIAN_POINT('Ctrl Pts',(-34.0429059658287,4.2394719479716,0.164903972384525));
#26484=CARTESIAN_POINT('Ctrl Pts',(-33.9239969668337,3.64559051443191,2.17025010513313));
#26485=CARTESIAN_POINT('Ctrl Pts',(-33.8050879678388,2.1658241961235,3.64822165845675));
#26486=CARTESIAN_POINT('Ctrl Pts',(-33.6861789688438,0.159758802036821,
4.23966895440156));
#26487=CARTESIAN_POINT('Ctrl Pts',(-33.5672699698489,-1.88512826096029,
3.80086926340264));
#26488=CARTESIAN_POINT('Ctrl Pts',(-33.4483609708539,-3.47192585240921,
2.43845167947057));
#26489=CARTESIAN_POINT('Ctrl Pts',(-33.360000091213,-4.02413102782502,0.985723265658703));
#26490=CARTESIAN_POINT('Ctrl Pts',(-33.3112755445704,-4.07066213174249,
0.155059660122451));
#26491=CARTESIAN_POINT('Ctrl Pts',(-33.3021873309261,-4.07050357498408,
0.00010473013306686));
#26492=CARTESIAN_POINT('Origin',(-55.3478126690739,0.,0.));
#26493=CARTESIAN_POINT('',(-36.5978126690739,-4.07025299976624,7.60445323442731E-5));
#26494=CARTESIAN_POINT('',(-36.3021873309261,-4.07084820048865,-6.23604784373507E-8));
#26495=CARTESIAN_POINT('',(-55.3478126690739,-4.0705,-3.42898509504556E-13));
#26496=CARTESIAN_POINT('Ctrl Pts',(-36.5978126690739,-4.07025299976624,
7.60445323443742E-5));
#26497=CARTESIAN_POINT('Ctrl Pts',(-36.5726368246093,-4.06996425256608,
-0.42925044427071));
#26498=CARTESIAN_POINT('Ctrl Pts',(-36.5078246471464,-3.89585403258829,
-1.53472847241628));
#26499=CARTESIAN_POINT('Ctrl Pts',(-36.4033761366853,-2.91160450999496,
-3.08591558397465));
#26500=CARTESIAN_POINT('Ctrl Pts',(-36.2844671376902,-1.08356448404466,
-4.10197559999513));
#26501=CARTESIAN_POINT('Ctrl Pts',(-36.1655581386953,1.00778361073219,-4.1212483555325));
#26502=CARTESIAN_POINT('Ctrl Pts',(-36.0466491397003,2.85423852172137,-3.1390505372104));
#26503=CARTESIAN_POINT('Ctrl Pts',(-35.9277401407054,4.00710846920256,-1.394057936416));
#26504=CARTESIAN_POINT('Ctrl Pts',(-35.8088311417104,4.18624403525991,0.689693186344611));
#26505=CARTESIAN_POINT('Ctrl Pts',(-35.6899221427155,3.34811496336391,2.60584765597262));
#26506=CARTESIAN_POINT('Ctrl Pts',(-35.5710131437205,1.69638808700519,3.88877657783347));
#26507=CARTESIAN_POINT('Ctrl Pts',(-35.4521041447256,-0.36756406781807,
4.22672597527783));
#26508=CARTESIAN_POINT('Ctrl Pts',(-35.3331951457305,-2.34219750991838,
3.53757355239032));
#26509=CARTESIAN_POINT('Ctrl Pts',(-35.2150979871801,-3.73807709597292,
1.99935877273991));
#26510=CARTESIAN_POINT('Ctrl Pts',(-35.1366371616278,-4.07070916646062,
0.661786854627458));
#26511=CARTESIAN_POINT('Ctrl Pts',(-35.0978126690738,-4.07084382520696,
-1.45670438656941E-5));
#26512=CARTESIAN_POINT('Ctrl Pts',(-36.3021873309261,-4.07084820044996,
-6.23604713442248E-8));
#26513=CARTESIAN_POINT('Ctrl Pts',(-36.3021838695284,-4.07084820050436,
-5.90650820220945E-5));
#26514=CARTESIAN_POINT('Ctrl Pts',(-36.2625440751324,-4.07083381658627,
-0.675755978339213));
#26515=CARTESIAN_POINT('Ctrl Pts',(-36.183267947738,-3.72710064368882,-2.02707585195046));
#26516=CARTESIAN_POINT('Ctrl Pts',(-36.064358948743,-2.30583140769797,-3.56138417430919));
#26517=CARTESIAN_POINT('Ctrl Pts',(-35.9454499497481,-0.324241098120267,
-4.23026990014066));
#26518=CARTESIAN_POINT('Ctrl Pts',(-35.8265409507531,1.73614036661006,-3.87119262568701));
#26519=CARTESIAN_POINT('Ctrl Pts',(-35.7076319517581,3.37463667925653,-2.5714087580085));
#26520=CARTESIAN_POINT('Ctrl Pts',(-35.5887229527632,4.19309036399278,-0.646768055130456));
#26521=CARTESIAN_POINT('Ctrl Pts',(-35.4698139537682,3.99261574089381,1.43503841875865));
#26522=CARTESIAN_POINT('Ctrl Pts',(-35.3509049547733,2.82192849475196,3.16812804164435));
#26523=CARTESIAN_POINT('Ctrl Pts',(-35.2319959557783,0.96550767828667,4.13135699751496));
#26524=CARTESIAN_POINT('Ctrl Pts',(-35.1130869567833,-1.12553319628343,
4.09065896180682));
#26525=CARTESIAN_POINT('Ctrl Pts',(-34.9941779577884,-2.94306753139286,
3.05592362852992));
#26526=CARTESIAN_POINT('Ctrl Pts',(-34.8905447491693,-3.90381478483326,
1.5069203921675));
#26527=CARTESIAN_POINT('Ctrl Pts',(-34.8265478735485,-4.06998382532337,
0.415364422931012));
#26528=CARTESIAN_POINT('Ctrl Pts',(-34.8021873309261,-4.07022604729797,
-6.65076760328689E-5));
#26529=CARTESIAN_POINT('Origin',(-55.3478126690739,0.,0.));
#26530=CARTESIAN_POINT('',(-38.0978126690739,-4.07046019877506,-0.000104814226016249));
#26531=CARTESIAN_POINT('',(-37.8021873309261,-4.07022625973033,6.65930553865601E-5));
#26532=CARTESIAN_POINT('',(-55.3478126690739,-4.0705,-3.42898509504556E-13));
#26533=CARTESIAN_POINT('Ctrl Pts',(-38.0978126690739,-4.07046019877506,
-0.000104814226015906));
#26534=CARTESIAN_POINT('Ctrl Pts',(-38.0879091535875,-4.07062966286641,
-0.168965898851486));
#26535=CARTESIAN_POINT('Ctrl Pts',(-38.0383693051028,-4.01905313428485,
-1.01354823242553));
#26536=CARTESIAN_POINT('Ctrl Pts',(-37.9491931236197,-3.44676120350641,
-2.47389430094654));
#26537=CARTESIAN_POINT('Ctrl Pts',(-37.8302841246248,-1.8460886395937,-3.81998331873136));
#26538=CARTESIAN_POINT('Ctrl Pts',(-37.7113751256298,0.203186699106992,
-4.23780969080775));
#26539=CARTESIAN_POINT('Ctrl Pts',(-37.5924661266349,2.20308731396286,-3.6258408821712));
#26540=CARTESIAN_POINT('Ctrl Pts',(-37.4735571276399,3.6676338500072,-2.13278638305928));
#26541=CARTESIAN_POINT('Ctrl Pts',(-37.3546481286449,4.24093893214488,-0.121461055132279));
#26542=CARTESIAN_POINT('Ctrl Pts',(-37.23573912965,3.78368842049889,1.91937952232278));
#26543=CARTESIAN_POINT('Ctrl Pts',(-37.116830130655,2.40699499087144,3.49380751156464));
#26544=CARTESIAN_POINT('Ctrl Pts',(-36.9979211316601,0.445397559627416,
4.219234151831));
#26545=CARTESIAN_POINT('Ctrl Pts',(-36.8790121326651,-1.62443225926818,
3.91937949796381));
#26546=CARTESIAN_POINT('Ctrl Pts',(-36.7601031336701,-3.2995221919603,2.66710875646485));
#26547=CARTESIAN_POINT('Ctrl Pts',(-36.6663699791397,-3.98792415159873,
1.16908185946355));
#26548=CARTESIAN_POINT('Ctrl Pts',(-36.6122731576076,-4.07041885023385,
0.246672371313648));
#26549=CARTESIAN_POINT('Ctrl Pts',(-36.5978126690739,-4.07025299976624,
7.60445323443742E-5));
#26550=CARTESIAN_POINT('Ctrl Pts',(-37.8021873309261,-4.07022625973033,
6.65930553865948E-5));
#26551=CARTESIAN_POINT('Ctrl Pts',(-37.7778198655082,-4.06998364140991,
-0.415482332889415));
#26552=CARTESIAN_POINT('Ctrl Pts',(-37.7138160670921,-3.90374786422602,
-1.5071565272805));
#26553=CARTESIAN_POINT('Ctrl Pts',(-37.6101759356775,-2.94280167197283,
-3.05617964738425));
#26554=CARTESIAN_POINT('Ctrl Pts',(-37.4912669366826,-1.12517732754963,
-4.09075686143469));
#26555=CARTESIAN_POINT('Ctrl Pts',(-37.3723579376876,0.965867079610468,
-4.13127298810448));
#26556=CARTESIAN_POINT('Ctrl Pts',(-37.2534489386927,2.82220409351303,-3.1678825376449));
#26557=CARTESIAN_POINT('Ctrl Pts',(-37.1345399396977,3.99274056611069,-1.43469107806466));
#26558=CARTESIAN_POINT('Ctrl Pts',(-37.0156309407027,4.19303408291871,0.647132828117663));
#26559=CARTESIAN_POINT('Ctrl Pts',(-36.8967219417077,3.37441296829128,2.57170232281563));
#26560=CARTESIAN_POINT('Ctrl Pts',(-36.7778129427128,1.73580358791025,3.87134364555039));
#26561=CARTESIAN_POINT('Ctrl Pts',(-36.6589039437178,-0.324609106740258,
4.23024167696931));
#26562=CARTESIAN_POINT('Ctrl Pts',(-36.5399949447229,-2.3061412194985,3.56118356638298));
#26563=CARTESIAN_POINT('Ctrl Pts',(-36.4210894071256,-3.7272356051144,2.02679627410343));
#26564=CARTESIAN_POINT('Ctrl Pts',(-36.3418202025267,-4.07084757762592,
0.675578845480269));
#26565=CARTESIAN_POINT('Ctrl Pts',(-36.3021873309261,-4.07084820044996,
-6.23604713442248E-8));
#26566=CARTESIAN_POINT('Origin',(-55.3478126690739,0.,0.));
#26567=CARTESIAN_POINT('',(-39.5978126690739,-4.07069839459796,9.13927329241537E-5));
#26568=CARTESIAN_POINT('',(-39.3021873309261,-4.07050320376008,-0.000104740849479479));
#26569=CARTESIAN_POINT('',(-55.3478126690739,-4.0705,-3.42898509504556E-13));
#26570=CARTESIAN_POINT('Ctrl Pts',(-39.5978126690739,-4.07069839459796,
9.13927329241997E-5));
#26571=CARTESIAN_POINT('Ctrl Pts',(-39.5635451495673,-4.07016736041225,
-0.584091196748413));
#26572=CARTESIAN_POINT('Ctrl Pts',(-39.4896412970624,-3.79600154444092,
-1.84449221170457));
#26573=CARTESIAN_POINT('Ctrl Pts',(-39.3761011115593,-2.54082596720782,
-3.39771596970325));
#26574=CARTESIAN_POINT('Ctrl Pts',(-39.2571921125643,-0.608870808304631,
-4.19876432921494));
#26575=CARTESIAN_POINT('Ctrl Pts',(-39.1382831135694,1.47103966436091,-3.97949033645411));
#26576=CARTESIAN_POINT('Ctrl Pts',(-39.0193741145744,3.19348560173252,-2.79320086500867));
#26577=CARTESIAN_POINT('Ctrl Pts',(-38.9004651155794,4.13990859901063,-0.928154854760866));
#26578=CARTESIAN_POINT('Ctrl Pts',(-38.7815561165844,4.08032672171768,1.16243249115508));
#26579=CARTESIAN_POINT('Ctrl Pts',(-38.6626471175895,3.02921821353002,2.97054766692245));
#26580=CARTESIAN_POINT('Ctrl Pts',(-38.5437381185945,1.24200441301907,4.05681407060795));
#26581=CARTESIAN_POINT('Ctrl Pts',(-38.4248291195996,-0.84701865830611,
4.15726778637903));
#26582=CARTESIAN_POINT('Ctrl Pts',(-38.3059201206046,-2.73021470026535,
3.2474980222978));
#26583=CARTESIAN_POINT('Ctrl Pts',(-38.196914637096,-3.84837514583954,1.69007750908748));
#26584=CARTESIAN_POINT('Ctrl Pts',(-38.1275454865858,-4.06995142540971,
0.506858174919875));
#26585=CARTESIAN_POINT('Ctrl Pts',(-38.0978126690739,-4.07046019877506,
-0.000104814226015906));
#26586=CARTESIAN_POINT('Ctrl Pts',(-39.3021873309261,-4.07050320376008,
-0.000104740849479045));
#26587=CARTESIAN_POINT('Ctrl Pts',(-39.2930921944864,-4.07066186300007,
-0.155177721080473));
#26588=CARTESIAN_POINT('Ctrl Pts',(-39.2443607250484,-4.02408852320218,
-0.985959385916872));
#26589=CARTESIAN_POINT('Ctrl Pts',(-39.155992922612,-3.47171371609164,-2.43875382264022));
#26590=CARTESIAN_POINT('Ctrl Pts',(-39.0370839236171,-1.88479759517879,
-3.80103318737441));
#26591=CARTESIAN_POINT('Ctrl Pts',(-38.9181749246221,0.160127626810078,
-4.23965506894654));
#26592=CARTESIAN_POINT('Ctrl Pts',(-38.7992659256272,2.16614156389975,-3.64803321565397));
#26593=CARTESIAN_POINT('Ctrl Pts',(-38.6803569266322,3.6457792997346,-2.16993295812935));
#26594=CARTESIAN_POINT('Ctrl Pts',(-38.5614479276372,4.23948627792256,-0.164535157769628));
#26595=CARTESIAN_POINT('Ctrl Pts',(-38.4425389286423,3.80299065872691,1.88084495893092));
#26596=CARTESIAN_POINT('Ctrl Pts',(-38.3236299296473,2.44236164439116,3.46917646169672));
#26597=CARTESIAN_POINT('Ctrl Pts',(-38.2047209306524,0.488234469363121,
4.21449199984978));
#26598=CARTESIAN_POINT('Ctrl Pts',(-38.0858119316573,-1.58453453732273,
3.93567859708109));
#26599=CARTESIAN_POINT('Ctrl Pts',(-37.9669029326625,-3.27225887423897,
2.70048839604023));
#26600=CARTESIAN_POINT('Ctrl Pts',(-37.8723613990853,-3.98191048253192,
1.19667333400869));
#26601=CARTESIAN_POINT('Ctrl Pts',(-37.8174561985065,-4.07037828649813,
0.260453195216987));
#26602=CARTESIAN_POINT('Ctrl Pts',(-37.8021873309261,-4.07022625973033,
6.65930553865948E-5));
#26603=CARTESIAN_POINT('Origin',(-55.3478126690739,0.,0.));
#26604=CARTESIAN_POINT('',(-41.0978126690738,-4.06894916332632,0.00540720055342753));
#26605=CARTESIAN_POINT('',(-40.8021873309261,-4.07070024200598,-0.000481747532086602));
#26606=CARTESIAN_POINT('',(-55.3478126690739,-4.0705,-3.42898509504556E-13));
#26607=CARTESIAN_POINT('Ctrl Pts',(-41.0978126690739,-4.06894916332632,
0.00540720055342749));
#26608=CARTESIAN_POINT('Ctrl Pts',(-41.0391811455472,-4.05939879775064,
-0.995808352670484));
#26609=CARTESIAN_POINT('Ctrl Pts',(-40.9012769560238,-3.18277581994412,
-3.36894444071793));
#26610=CARTESIAN_POINT('Ctrl Pts',(-40.7237364335021,0.0468138156189731,
-4.48441463662212));
#26611=CARTESIAN_POINT('Ctrl Pts',(-40.5651911015089,2.60148923263442,-3.34401588370882));
#26612=CARTESIAN_POINT('Ctrl Pts',(-40.4462821025139,3.88717861421759,-1.70434784922236));
#26613=CARTESIAN_POINT('Ctrl Pts',(-40.327373103519,4.22697739474136,0.364600408636661));
#26614=CARTESIAN_POINT('Ctrl Pts',(-40.208464104524,3.54029037696192,2.33730890925922));
#26615=CARTESIAN_POINT('Ctrl Pts',(-40.0895551055291,1.99296520133986,3.74588177308733));
#26616=CARTESIAN_POINT('Ctrl Pts',(-39.9706461065341,-0.0384827646914282,
4.24227672531885));
#26617=CARTESIAN_POINT('Ctrl Pts',(-39.8517371075391,-2.06066518446267,
3.70875428242689));
#26618=CARTESIAN_POINT('Ctrl Pts',(-39.7328281085442,-3.58205933615999,
2.27351529266644));
#26619=CARTESIAN_POINT('Ctrl Pts',(-39.6481866290558,-4.04543032394026,
0.858803192571973));
#26620=CARTESIAN_POINT('Ctrl Pts',(-39.6031814825656,-4.0707815936022,0.0916173453910432));
#26621=CARTESIAN_POINT('Ctrl Pts',(-39.5978126690739,-4.07069839459796,
9.13927329241997E-5));
#26622=CARTESIAN_POINT('Ctrl Pts',(-40.8021873309261,-4.07070024200598,
-0.000481747532086515));
#26623=CARTESIAN_POINT('Ctrl Pts',(-40.7687281904663,-4.07015465516028,
-0.570964956116361));
#26624=CARTESIAN_POINT('Ctrl Pts',(-40.695632717008,-3.80565769799185,-1.81613807110307));
#26625=CARTESIAN_POINT('Ctrl Pts',(-40.5829009105516,-2.57524274258496,
-3.37219103126866));
#26626=CARTESIAN_POINT('Ctrl Pts',(-40.4639919115566,-0.651474730133847,
-4.1921317137068));
#26627=CARTESIAN_POINT('Ctrl Pts',(-40.3450829125617,1.43053090860402,-3.99434390257198));
#26628=CARTESIAN_POINT('Ctrl Pts',(-40.2261739135667,3.1649510603171,-2.82543882253934));
#26629=CARTESIAN_POINT('Ctrl Pts',(-40.1072649145718,4.13026449432683,-0.970190141382548));
#26630=CARTESIAN_POINT('Ctrl Pts',(-39.9883559155767,4.09192547196896,1.12093825548876));
#26631=CARTESIAN_POINT('Ctrl Pts',(-39.8694469165819,3.0592368484789,2.93961562653621));
#26632=CARTESIAN_POINT('Ctrl Pts',(-39.7505379175868,1.28315058440506,4.04399186048308));
#26633=CARTESIAN_POINT('Ctrl Pts',(-39.6316289185919,-0.804744661503545,
4.16565563790974));
#26634=CARTESIAN_POINT('Ctrl Pts',(-39.5127199195969,-2.69708497226697,
3.27506548731581));
#26635=CARTESIAN_POINT('Ctrl Pts',(-39.4029060570417,-3.83941754526237,
1.7176176530298));
#26636=CARTESIAN_POINT('Ctrl Pts',(-39.3327285274847,-4.0699704307702,0.520625695858415));
#26637=CARTESIAN_POINT('Ctrl Pts',(-39.3021873309261,-4.07050320376008,
-0.000104740849479045));
#26638=CARTESIAN_POINT('Origin',(-55.3478126690739,0.,0.));
#26639=CARTESIAN_POINT('',(-42.5978126690739,-4.07077051219227,-5.79810753342639E-5));
#26640=CARTESIAN_POINT('',(-42.3021873309261,-4.0702562437931,0.000377661753542397));
#26641=CARTESIAN_POINT('',(-55.3478126690739,-4.0705,-3.42898509504556E-13));
#26642=CARTESIAN_POINT('Ctrl Pts',(-42.5978126690739,-4.07077051219227,
-5.79810753340362E-5));
#26643=CARTESIAN_POINT('Ctrl Pts',(-42.5940898075237,-4.07081705779188,
-0.0635213374655559));
#26644=CARTESIAN_POINT('Ctrl Pts',(-42.5507306129751,-4.05388726315202,
-0.802638451157566));
#26645=CARTESIAN_POINT('Ctrl Pts',(-42.4677350854283,-3.62830976367934,
-2.19902748573468));
#26646=CARTESIAN_POINT('Ctrl Pts',(-42.3488260864333,-2.13693866142688,
-3.66517585267858));
#26647=CARTESIAN_POINT('Ctrl Pts',(-42.2299170874383,-0.126195704091931,
-4.24090485322945));
#26648=CARTESIAN_POINT('Ctrl Pts',(-42.1110080884434,1.91502942438633,-3.78563799657268));
#26649=CARTESIAN_POINT('Ctrl Pts',(-41.9920990894484,3.49126541284734,-2.41134949120931));
#26650=CARTESIAN_POINT('Ctrl Pts',(-41.8731900904535,4.21838674592901,-0.449312978092323));
#26651=CARTESIAN_POINT('Ctrl Pts',(-41.7542810914585,3.92189134396604,1.61834472216421));
#26652=CARTESIAN_POINT('Ctrl Pts',(-41.6353720924635,2.66945995165433,3.29983980467131));
#26653=CARTESIAN_POINT('Ctrl Pts',(-41.5164630934686,0.77413855912781,4.16544090694865));
#26654=CARTESIAN_POINT('Ctrl Pts',(-41.3579177614753,-2.01888556396995,
4.00453083969612));
#26655=CARTESIAN_POINT('Ctrl Pts',(-41.2183676200104,-3.8707199036833,2.05940273537045));
#26656=CARTESIAN_POINT('Ctrl Pts',(-41.1184538115438,-4.07231135561863,
0.35788367795225));
#26657=CARTESIAN_POINT('Ctrl Pts',(-41.0978126690739,-4.06894916332632,
0.00540720055342749));
#26658=CARTESIAN_POINT('Ctrl Pts',(-42.3021873309261,-4.0702562437931,0.000377661753542743));
#26659=CARTESIAN_POINT('Ctrl Pts',(-42.2840005194444,-4.070361788608,-0.309619941943036));
#26660=CARTESIAN_POINT('Ctrl Pts',(-42.2261773749644,-3.95913933202493,
-1.29545265190419));
#26661=CARTESIAN_POINT('Ctrl Pts',(-42.1287178974861,-3.17025358567157,
-2.82214018180611));
#26662=CARTESIAN_POINT('Ctrl Pts',(-42.0098088984911,-1.44080606975949,
-3.98424622002752));
#26663=CARTESIAN_POINT('Ctrl Pts',(-41.8512635664978,1.34123824569469,-4.27940453375867));
#26664=CARTESIAN_POINT('Ctrl Pts',(-41.6530819015062,4.38508519896316,-1.98115288915087));
#26665=CARTESIAN_POINT('Ctrl Pts',(-41.4152639035164,4.03738586191726,2.61791030678041));
#26666=CARTESIAN_POINT('Ctrl Pts',(-41.2170822385246,0.682605700869055,
4.43241160683543));
#26667=CARTESIAN_POINT('Ctrl Pts',(-41.0585369065315,-2.02344112387514,
3.7223414795892));
#26668=CARTESIAN_POINT('Ctrl Pts',(-40.9396279075364,-3.55851407251,2.3134304828493));
#26669=CARTESIAN_POINT('Ctrl Pts',(-40.8541780490014,-4.04108036770983,
0.886096610966636));
#26670=CARTESIAN_POINT('Ctrl Pts',(-40.8083645234646,-4.07080096769546,
0.1048402831881));
#26671=CARTESIAN_POINT('Ctrl Pts',(-40.8021873309261,-4.07070024200598,
-0.000481747532086515));
#26672=CARTESIAN_POINT('Origin',(-55.3478126690739,0.,0.));
#26673=CARTESIAN_POINT('',(-44.0978126690739,-4.0703765947929,9.98552879098336E-5));
#26674=CARTESIAN_POINT('',(-43.8021873309261,-4.07079741683127,-5.00544118864354E-5));
#26675=CARTESIAN_POINT('',(-55.3478126690739,-4.0705,-3.42898509504556E-13));
#26676=CARTESIAN_POINT('Ctrl Pts',(-44.0978126690739,-4.0703765947929,9.98552879100285E-5));
#26677=CARTESIAN_POINT('Ctrl Pts',(-44.0697258035035,-4.06993441861034,
-0.478826892483599));
#26678=CARTESIAN_POINT('Ctrl Pts',(-44.0020026049348,-3.86611252863601,
-1.63398403157745));
#26679=CARTESIAN_POINT('Ctrl Pts',(-43.8946430733678,-2.79679600676983,
-3.19033664959511));
#26680=CARTESIAN_POINT('Ctrl Pts',(-43.7757340743728,-0.932818792342456,
-4.1388603280403));
#26681=CARTESIAN_POINT('Ctrl Pts',(-43.6568250753779,1.15783504670461,-4.0816337488567));
#26682=CARTESIAN_POINT('Ctrl Pts',(-43.5379160763829,2.96713289393957,-3.03256290209179));
#26683=CARTESIAN_POINT('Ctrl Pts',(-43.4190070773879,4.05541233929616,-1.24657417947145));
#26684=CARTESIAN_POINT('Ctrl Pts',(-43.300098078393,4.15821929464979,0.842334701919917));
#26685=CARTESIAN_POINT('Ctrl Pts',(-43.181189079398,3.25057203925852,2.72655387993142));
#26686=CARTESIAN_POINT('Ctrl Pts',(-43.0622800804031,1.55302935037421,3.94821747091449));
#26687=CARTESIAN_POINT('Ctrl Pts',(-42.9433710814082,-0.521900734955894,
4.21045373503939));
#26688=CARTESIAN_POINT('Ctrl Pts',(-42.824462082413,-2.47001093572135,3.44954946781609));
#26689=CARTESIAN_POINT('Ctrl Pts',(-42.7092759449685,-3.7756980222501,1.90045190076457));
#26690=CARTESIAN_POINT('Ctrl Pts',(-42.633726140522,-4.07032149896954,0.612156415560098));
#26691=CARTESIAN_POINT('Ctrl Pts',(-42.5978126690739,-4.07077051219227,
-5.79810753340362E-5));
#26692=CARTESIAN_POINT('Ctrl Pts',(-43.8021873309261,-4.07079741683127,
-5.00544118866002E-5));
#26693=CARTESIAN_POINT('Ctrl Pts',(-43.7992728484226,-4.07082805237793,
-0.0497319009987912));
#26694=CARTESIAN_POINT('Ctrl Pts',(-43.7567220329207,-4.057824297978,-0.775060067942204));
#26695=CARTESIAN_POINT('Ctrl Pts',(-43.6745348844206,-3.65047141713449,
-2.16202982679776));
#26696=CARTESIAN_POINT('Ctrl Pts',(-43.5556258854256,-2.17403874853064,
-3.64333320102936));
#26697=CARTESIAN_POINT('Ctrl Pts',(-43.4367168864307,-0.169311716792706,
-4.23929645182126));
#26698=CARTESIAN_POINT('Ctrl Pts',(-43.3178078874356,1.87656008092686,-3.80511075431245));
#26699=CARTESIAN_POINT('Ctrl Pts',(-43.1988988884407,3.46642105478168,-2.44626147372541));
#26700=CARTESIAN_POINT('Ctrl Pts',(-43.0799898894457,4.21394248881074,-0.492996289805673));
#26701=CARTESIAN_POINT('Ctrl Pts',(-42.9610808904508,3.9374548435202,1.58012754509629));
#26702=CARTESIAN_POINT('Ctrl Pts',(-42.8421718914559,2.70418603569597,3.26915855205306));
#26703=CARTESIAN_POINT('Ctrl Pts',(-42.7232628924609,0.813740892457039,
4.16401580837881));
#26704=CARTESIAN_POINT('Ctrl Pts',(-42.6043538934659,-1.2743362201606,4.04653615170507));
#26705=CARTESIAN_POINT('Ctrl Pts',(-42.485444894471,-3.05296381848078,2.94668618241789));
#26706=CARTESIAN_POINT('Ctrl Pts',(-42.3847227069577,-3.93078173750272,
1.40692650742191));
#26707=CARTESIAN_POINT('Ctrl Pts',(-42.3236368524427,-4.07013176426131,
0.365988768312008));
#26708=CARTESIAN_POINT('Ctrl Pts',(-42.3021873309261,-4.0702562437931,0.000377661753542743));
#26709=CARTESIAN_POINT('Origin',(-55.3478126690739,0.,0.));
#26710=CARTESIAN_POINT('',(-45.5978126690739,-4.07031822057863,-9.16775258372991E-5));
#26711=CARTESIAN_POINT('',(-45.3021873309261,-4.07033855687931,9.50420136142105E-5));
#26712=CARTESIAN_POINT('',(-55.3478126690739,-4.0705,-3.42898509504556E-13));
#26713=CARTESIAN_POINT('Ctrl Pts',(-45.5978126690739,-4.07031822057863,
-9.16775258373928E-5));
#26714=CARTESIAN_POINT('Ctrl Pts',(-45.5849981324817,-4.07049943661512,
-0.218609364827659));
#26715=CARTESIAN_POINT('Ctrl Pts',(-45.5325472628912,-3.99970860043998,
-1.11290258178099));
#26716=CARTESIAN_POINT('Ctrl Pts',(-45.4404600603022,-3.35397801744653,
-2.59829699467222));
#26717=CARTESIAN_POINT('Ctrl Pts',(-45.3215510613074,-1.70514605769533,
-3.88494436716616));
#26718=CARTESIAN_POINT('Ctrl Pts',(-45.2026420623123,0.358039382745663,
-4.22754344914553));
#26719=CARTESIAN_POINT('Ctrl Pts',(-45.0837330633174,2.33422062563635,-3.54284206322451));
#26720=CARTESIAN_POINT('Ctrl Pts',(-44.9648240643225,3.74318216521078,-1.997223846241));
#26721=CARTESIAN_POINT('Ctrl Pts',(-44.8459150653275,4.24254387784786,0.0337232659310005));
#26722=CARTESIAN_POINT('Ctrl Pts',(-44.7270060663325,3.71095999205786,2.05647556548625));
#26723=CARTESIAN_POINT('Ctrl Pts',(-44.6080970673375,2.27760632395248,3.57950069794286));
#26724=CARTESIAN_POINT('Ctrl Pts',(-44.4891880683426,0.290790326898236,
4.23270088732366));
#26725=CARTESIAN_POINT('Ctrl Pts',(-44.3702790693477,-1.76668822890541,
3.85734734137919));
#26726=CARTESIAN_POINT('Ctrl Pts',(-44.2513700703527,-3.39485844927514,
2.54465163234734));
#26727=CARTESIAN_POINT('Ctrl Pts',(-44.1605479369281,-4.00834926416774,
1.06972434003999));
#26728=CARTESIAN_POINT('Ctrl Pts',(-44.1093621365018,-4.07055841997397,
0.197037062820157));
#26729=CARTESIAN_POINT('Ctrl Pts',(-44.0978126690739,-4.0703765947929,9.98552879100285E-5));
#26730=CARTESIAN_POINT('Ctrl Pts',(-45.3021873309261,-4.07033855687931,
9.5042013614384E-5));
#26731=CARTESIAN_POINT('Ctrl Pts',(-45.2749088444024,-4.06993566613643,
-0.465059999241131));
#26732=CARTESIAN_POINT('Ctrl Pts',(-45.2079940248804,-3.87457928875426,
-1.6064268825154));
#26733=CARTESIAN_POINT('Ctrl Pts',(-45.1014428723601,-2.82905982713036,
-3.16176156781322));
#26734=CARTESIAN_POINT('Ctrl Pts',(-44.9825338733652,-0.974814091813329,
-4.12917100710215));
#26735=CARTESIAN_POINT('Ctrl Pts',(-44.8636248743702,1.11631317618967,-4.09318465336435));
#26736=CARTESIAN_POINT('Ctrl Pts',(-44.7447158753752,2.93617438620888,-3.06254725647695));
#26737=CARTESIAN_POINT('Ctrl Pts',(-44.6258068763803,4.04254007317222,-1.28770550464645));
#26738=CARTESIAN_POINT('Ctrl Pts',(-44.5068978773853,4.16656143857104,0.800050934283993));
#26739=CARTESIAN_POINT('Ctrl Pts',(-44.3879888783903,3.27810106806685,2.69339360894175));
#26740=CARTESIAN_POINT('Ctrl Pts',(-44.2690798793954,1.59305639924211,3.93223688581989));
#26741=CARTESIAN_POINT('Ctrl Pts',(-44.1501708804004,-0.479103780509667,
4.21553976710139));
#26742=CARTESIAN_POINT('Ctrl Pts',(-44.0312618814054,-2.4348408745219,3.47445897688703));
#26743=CARTESIAN_POINT('Ctrl Pts',(-43.915267364914,-3.76547388867547,1.92793677744289));
#26744=CARTESIAN_POINT('Ctrl Pts',(-43.8389091814209,-4.07041141555569,
0.625930489462706));
#26745=CARTESIAN_POINT('Ctrl Pts',(-43.8021873309261,-4.07079741683127,
-5.00544118866002E-5));
#26746=CARTESIAN_POINT('Origin',(-55.3478126690739,0.,0.));
#26747=CARTESIAN_POINT('',(-47.0978126690739,-4.07081123287269,4.27420414081398E-5));
#26748=CARTESIAN_POINT('',(-46.8021873309261,-4.07035480316255,-9.73195009795758E-5));
#26749=CARTESIAN_POINT('',(-55.3478126690739,-4.0705,-3.42898509504556E-13));
#26750=CARTESIAN_POINT('Ctrl Pts',(-47.0978126690739,-4.07081123287269,
4.27420414080091E-5));
#26751=CARTESIAN_POINT('Ctrl Pts',(-47.0606341284615,-4.07046881201322,
-0.633716584336426));
#26752=CARTESIAN_POINT('Ctrl Pts',(-46.9838192548509,-3.7596214042551,-1.94345587087894));
#26753=CARTESIAN_POINT('Ctrl Pts',(-46.8673680482418,-2.41486120468549,
-3.4883751484243));
#26754=CARTESIAN_POINT('Ctrl Pts',(-46.748459049247,-0.454903300248022,
-4.21821986167895));
#26755=CARTESIAN_POINT('Ctrl Pts',(-46.6295500502518,1.61559690347559,-3.92302975511522));
#26756=CARTESIAN_POINT('Ctrl Pts',(-46.510641051257,3.29350422793804,-2.67453654201874));
#26757=CARTESIAN_POINT('Ctrl Pts',(-46.391732052262,4.17108425236453,-0.776126261452312));
#26758=CARTESIAN_POINT('Ctrl Pts',(-46.2728230532671,4.03508349265237,1.3108840609923));
#26759=CARTESIAN_POINT('Ctrl Pts',(-46.153914054272,2.91855037178518,3.0793472589807));
#26760=CARTESIAN_POINT('Ctrl Pts',(-46.0350050552771,1.09280439512275,4.09952367575057));
#26761=CARTESIAN_POINT('Ctrl Pts',(-45.9160960562821,-0.998494964953347,
4.123508653926));
#26762=CARTESIAN_POINT('Ctrl Pts',(-45.7971870572872,-2.84715829844654,
3.14547380177063));
#26763=CARTESIAN_POINT('Ctrl Pts',(-45.6910925948844,-3.87929174472671,
1.59085653253142));
#26764=CARTESIAN_POINT('Ctrl Pts',(-45.62463446548,-4.06993892167843,0.457282405241305));
#26765=CARTESIAN_POINT('Ctrl Pts',(-45.5978126690739,-4.07031822057863,
-9.16775258373928E-5));
#26766=CARTESIAN_POINT('Ctrl Pts',(-46.8021873309261,-4.07035480316255,
-9.73195009796278E-5));
#26767=CARTESIAN_POINT('Ctrl Pts',(-46.7901811733806,-4.07053748381602,
-0.204824980679389));
#26768=CARTESIAN_POINT('Ctrl Pts',(-46.7385386828367,-4.00527158843597,
-1.08531156100483));
#26769=CARTESIAN_POINT('Ctrl Pts',(-46.6472598592946,-3.38019901859953,
-2.5640924929505));
#26770=CARTESIAN_POINT('Ctrl Pts',(-46.5283508602997,-1.74452217827771,
-3.8674226672609));
#26771=CARTESIAN_POINT('Ctrl Pts',(-46.4094418613047,0.315076609054344,
-4.23096235485186));
#26772=CARTESIAN_POINT('Ctrl Pts',(-46.2905328623097,2.29811122813968,-3.56637077444897));
#26773=CARTESIAN_POINT('Ctrl Pts',(-46.1716238633148,3.72270079080243,-2.03514484494512));
#26774=CARTESIAN_POINT('Ctrl Pts',(-46.0527148643198,4.2426675363842,-0.00937515104479359));
#26775=CARTESIAN_POINT('Ctrl Pts',(-45.9338058653248,3.7316586343443,2.01867272098968));
#26776=CARTESIAN_POINT('Ctrl Pts',(-45.8148968663299,2.31385014354139,3.5561795836249));
#26777=CARTESIAN_POINT('Ctrl Pts',(-45.6959878673349,0.333772012288686,
4.22952857438387));
#26778=CARTESIAN_POINT('Ctrl Pts',(-45.57707886834,-1.7274133029682,3.87509470833104));
#26779=CARTESIAN_POINT('Ctrl Pts',(-45.458169869345,-3.36883415789558,2.57900603610148));
#26780=CARTESIAN_POINT('Ctrl Pts',(-45.3665393568737,-4.00286950955251,
1.09731510772082));
#26781=CARTESIAN_POINT('Ctrl Pts',(-45.3145451774007,-4.07052107660754,
0.21082207709823));
#26782=CARTESIAN_POINT('Ctrl Pts',(-45.3021873309261,-4.07033855687931,
9.5042013614384E-5));
#26783=CARTESIAN_POINT('Origin',(-55.3478126690739,0.,0.));
#26784=CARTESIAN_POINT('',(-48.5978126690739,-4.07016989220343,3.24954791586653E-5));
#26785=CARTESIAN_POINT('',(-48.3021873309261,-4.07078561771882,5.53476569591441E-5));
#26786=CARTESIAN_POINT('',(-55.3478126690739,-4.0705,-3.42898509504556E-13));
#26787=CARTESIAN_POINT('Ctrl Pts',(-48.5978126690739,-4.07016989220343,
3.24954791586923E-5));
#26788=CARTESIAN_POINT('Ctrl Pts',(-48.5759064574397,-4.0700653077914,-0.373558418857458));
#26789=CARTESIAN_POINT('Ctrl Pts',(-48.5143639128072,-3.92681617951824,
-1.42319027041692));
#26790=CARTESIAN_POINT('Ctrl Pts',(-48.4131850351763,-3.03590383707744,
-2.96371451156447));
#26791=CARTESIAN_POINT('Ctrl Pts',(-48.2942760361814,-1.2511421580073,-4.05400531752194));
#26792=CARTESIAN_POINT('Ctrl Pts',(-48.1753670371864,0.837649258381883,
-4.15916572571611));
#26793=CARTESIAN_POINT('Ctrl Pts',(-48.0564580381915,2.72289043680534,-3.25364157263724));
#26794=CARTESIAN_POINT('Ctrl Pts',(-47.9375490391965,3.94646446657405,-1.55747681462926));
#26795=CARTESIAN_POINT('Ctrl Pts',(-47.8186400402015,4.21104071385062,0.517157539180999));
#26796=CARTESIAN_POINT('Ctrl Pts',(-47.6997310412066,3.45232668681426,2.46612170452907));
#26797=CARTESIAN_POINT('Ctrl Pts',(-47.5808220422116,1.85469122386101,3.81581397321361));
#26798=CARTESIAN_POINT('Ctrl Pts',(-47.4619130432167,-0.193637457276558,
4.23825675828857));
#26799=CARTESIAN_POINT('Ctrl Pts',(-47.3430040442216,-2.19491189690037,
3.6307957225496));
#26800=CARTESIAN_POINT('Ctrl Pts',(-47.2240950452268,-3.66281889847391,
2.14104496240076));
#26801=CARTESIAN_POINT('Ctrl Pts',(-47.1423645868441,-4.05998621113554,
0.759479672593957));
#26802=CARTESIAN_POINT('Ctrl Pts',(-47.1002704614598,-4.0708338695703,0.0419391914783086));
#26803=CARTESIAN_POINT('Ctrl Pts',(-47.0978126690739,-4.07081123287269,
4.27420414080091E-5));
#26804=CARTESIAN_POINT('Ctrl Pts',(-48.3021873309261,-4.07078561771882,
5.53476569592308E-5));
#26805=CARTESIAN_POINT('Ctrl Pts',(-48.2658171693605,-4.07036989113885,
-0.6199353689415));
#26806=CARTESIAN_POINT('Ctrl Pts',(-48.1898106747964,-3.76994384664287,
-1.91598331380283));
#26807=CARTESIAN_POINT('Ctrl Pts',(-48.0741678472342,-2.45017226913454,
-3.46366447123714));
#26808=CARTESIAN_POINT('Ctrl Pts',(-47.9552588482392,-0.497729416154917,
-4.21338120113056));
#26809=CARTESIAN_POINT('Ctrl Pts',(-47.8363498492442,1.57566255733915,-3.93923891419978));
#26810=CARTESIAN_POINT('Ctrl Pts',(-47.7174408502492,3.26616576767762,-2.70785466666829));
#26811=CARTESIAN_POINT('Ctrl Pts',(-47.5985318512543,4.16298497174054,-0.818456988979114));
#26812=CARTESIAN_POINT('Ctrl Pts',(-47.4796228522594,4.04819153105236,1.26982717157192));
#26813=CARTESIAN_POINT('Ctrl Pts',(-47.3607138532644,2.94968045290301,3.04954110375778));
#26814=CARTESIAN_POINT('Ctrl Pts',(-47.2418048542694,1.13439185468392,4.08821120268671));
#26815=CARTESIAN_POINT('Ctrl Pts',(-47.1228958552744,-0.956555952514039,
4.13343881380338));
#26816=CARTESIAN_POINT('Ctrl Pts',(-47.0039868562795,-2.81505898666,3.17423354833433));
#26817=CARTESIAN_POINT('Ctrl Pts',(-46.8970840148301,-3.8709155012229,1.61841633454085));
#26818=CARTESIAN_POINT('Ctrl Pts',(-46.8298175063789,-4.06993439401099,
0.471049354774862));
#26819=CARTESIAN_POINT('Ctrl Pts',(-46.8021873309261,-4.07035480316255,
-9.73195009796278E-5));
#26820=CARTESIAN_POINT('Origin',(-55.3478126690739,0.,0.));
#26821=CARTESIAN_POINT('',(-50.0978126690739,-4.07063454056454,-9.39916809451252E-5));
#26822=CARTESIAN_POINT('',(-49.8021873309261,-4.07016024360026,2.01151063877747E-5));
#26823=CARTESIAN_POINT('',(-55.3478126690739,-4.0705,-3.42898509504556E-13));
#26824=CARTESIAN_POINT('Ctrl Pts',(-50.0978126690739,-4.07063454056454,
-9.39916809453677E-5));
#26825=CARTESIAN_POINT('Ctrl Pts',(-50.0911787864178,-4.07074638038891,
-0.113191851380465));
#26826=CARTESIAN_POINT('Ctrl Pts',(-50.0449085707635,-4.03852758336781,
-0.901966869774806));
#26827=CARTESIAN_POINT('Ctrl Pts',(-49.9590020221109,-3.54546957514818,
-2.33022773676946));
#26828=CARTESIAN_POINT('Ctrl Pts',(-49.8400930231158,-2.00143969166412,
-3.74092969395146));
#26829=CARTESIAN_POINT('Ctrl Pts',(-49.721184024121,0.0289435448964663,
-4.2425791784024));
#26830=CARTESIAN_POINT('Ctrl Pts',(-49.6022750251259,2.05229344931449,-3.71327448649327));
#26831=CARTESIAN_POINT('Ctrl Pts',(-49.4833660261311,3.57693244841941,-2.28163758591345));
#26832=CARTESIAN_POINT('Ctrl Pts',(-49.364457027136,4.23237059313566,-0.295558752875362));
#26833=CARTESIAN_POINT('Ctrl Pts',(-49.2455480281411,3.85933526548734,1.76234137516302));
#26834=CARTESIAN_POINT('Ctrl Pts',(-49.1266390291461,2.54847470392539,3.39198946010828));
#26835=CARTESIAN_POINT('Ctrl Pts',(-49.0077300301511,0.618330322503512,
4.19737816098522));
#26836=CARTESIAN_POINT('Ctrl Pts',(-48.8888210311563,-1.46206941105725,
3.98279661184051));
#26837=CARTESIAN_POINT('Ctrl Pts',(-48.7699120321612,-3.18718371510779,
2.80038850522416));
#26838=CARTESIAN_POINT('Ctrl Pts',(-48.6729092448004,-3.96267664484684,
1.28067835687247));
#26839=CARTESIAN_POINT('Ctrl Pts',(-48.615542790438,-4.0702545391679,0.302403912424053));
#26840=CARTESIAN_POINT('Ctrl Pts',(-48.5978126690739,-4.07016989220343,
3.24954791586923E-5));
#26841=CARTESIAN_POINT('Ctrl Pts',(-49.8021873309261,-4.07016024360026,
2.01151063877747E-5));
#26842=CARTESIAN_POINT('Ctrl Pts',(-49.7810894983386,-4.07009807335129,
-0.359787051715212));
#26843=CARTESIAN_POINT('Ctrl Pts',(-49.7203553327528,-3.93407799572834,
-1.39560723718365));
#26844=CARTESIAN_POINT('Ctrl Pts',(-49.6199848341687,-3.06585324049081,
-2.93272222099405));
#26845=CARTESIAN_POINT('Ctrl Pts',(-49.5010758351736,-1.29225906223574,
-4.04108676395591));
#26846=CARTESIAN_POINT('Ctrl Pts',(-49.3821668361788,0.795356333133346,
-4.167460140312));
#26847=CARTESIAN_POINT('Ctrl Pts',(-49.2632578371837,2.68969874550031,-3.28113339811124));
#26848=CARTESIAN_POINT('Ctrl Pts',(-49.1443488381888,3.93043964837605,-1.59748548920479));
#26849=CARTESIAN_POINT('Ctrl Pts',(-49.0254398391938,4.216076827669,0.474354193550262));
#26850=CARTESIAN_POINT('Ctrl Pts',(-48.9065308401989,3.47719994816421,2.43092497585451));
#26851=CARTESIAN_POINT('Ctrl Pts',(-48.7876218412039,1.89335738663818,3.79677672825371));
#26852=CARTESIAN_POINT('Ctrl Pts',(-48.6687128422089,-0.150574338398622,
4.24000508093589));
#26853=CARTESIAN_POINT('Ctrl Pts',(-48.549803843214,-2.15791623528735,3.65290476733649));
#26854=CARTESIAN_POINT('Ctrl Pts',(-48.430894844219,-3.64088070474142,2.17814219269265));
#26855=CARTESIAN_POINT('Ctrl Pts',(-48.3483560067898,-4.0561286694033,0.787058534453424));
#26856=CARTESIAN_POINT('Ctrl Pts',(-48.3054535023588,-4.07082295146222,
0.0557327458286881));
#26857=CARTESIAN_POINT('Ctrl Pts',(-48.3021873309261,-4.07078561771882,
5.53476569592308E-5));
#26858=CARTESIAN_POINT('Origin',(-55.3478126690739,0.,0.));
#26859=CARTESIAN_POINT('',(-51.5978126690739,-4.07052776695671,0.0001044975750702));
#26860=CARTESIAN_POINT('',(-51.3021873309261,-4.07067545460402,-8.7070919803367E-5));
#26861=CARTESIAN_POINT('',(-55.3478126690739,-4.0705,-3.42898509504556E-13));
#26862=CARTESIAN_POINT('Ctrl Pts',(-51.5978126690739,-4.07052776695671,
0.00010449757507032));
#26863=CARTESIAN_POINT('Ctrl Pts',(-51.5668147823977,-4.0699845460846,-0.528403488877145));
#26864=CARTESIAN_POINT('Ctrl Pts',(-51.4961805627232,-3.83428485658603,
-1.73317487318012));
#26865=CARTESIAN_POINT('Ctrl Pts',(-51.3859100100504,-2.67824533662262,
-3.29048853499884));
#26866=CARTESIAN_POINT('Ctrl Pts',(-51.2670010110555,-0.78082496558402,
-4.17020743213141));
#26867=CARTESIAN_POINT('Ctrl Pts',(-51.1480920120604,1.30633725885353,-4.03655767907646));
#26868=CARTESIAN_POINT('Ctrl Pts',(-51.0291830130655,3.07605723061235,-2.9220178035111));
#26869=CARTESIAN_POINT('Ctrl Pts',(-50.9102740140706,4.09828990837908,-1.0974222453584));
#26870=CARTESIAN_POINT('Ctrl Pts',(-50.7913650150755,4.12463095289654,0.993848724235651));
#26871=CARTESIAN_POINT('Ctrl Pts',(-50.6724560160807,3.14867944761336,2.84361277085736));
#26872=CARTESIAN_POINT('Ctrl Pts',(-50.5535470170857,1.40759331717813,4.00237390050092));
#26873=CARTESIAN_POINT('Ctrl Pts',(-50.4346380180907,-0.675540456184353,
4.18855117202478));
#26874=CARTESIAN_POINT('Ctrl Pts',(-50.3157290190957,-2.59451671479358,
3.35690315989496));
#26875=CARTESIAN_POINT('Ctrl Pts',(-50.2034539027568,-3.81113576375281,
1.80142850771877));
#26876=CARTESIAN_POINT('Ctrl Pts',(-50.1308151194162,-4.07007815625064,
0.56254883637138));
#26877=CARTESIAN_POINT('Ctrl Pts',(-50.0978126690739,-4.07063454056454,
-9.39916809453677E-5));
#26878=CARTESIAN_POINT('Ctrl Pts',(-51.3021873309261,-4.07067545460402,
-8.70709198036793E-5));
#26879=CARTESIAN_POINT('Ctrl Pts',(-51.2963618273168,-4.07076913219396,
-0.0994003816391395));
#26880=CARTESIAN_POINT('Ctrl Pts',(-51.2508999907091,-4.04297867155526,
-0.874382431947933));
#26881=CARTESIAN_POINT('Ctrl Pts',(-51.1658018211031,-3.56895759144185,
-2.29409186145612));
#26882=CARTESIAN_POINT('Ctrl Pts',(-51.0468928221082,-2.03933759109846,
-3.72040560679174));
#26883=CARTESIAN_POINT('Ctrl Pts',(-50.9279838231133,-0.0141549843878351,
-4.24265428344519));
#26884=CARTESIAN_POINT('Ctrl Pts',(-50.8090748241182,2.01446730968869,-3.73393052561418));
#26885=CARTESIAN_POINT('Ctrl Pts',(-50.6901658251233,3.55357051600268,-2.31785510914493));
#26886=CARTESIAN_POINT('Ctrl Pts',(-50.5712568261283,4.22914985879238,-0.338536836715756));
#26887=CARTESIAN_POINT('Ctrl Pts',(-50.4523478271334,3.87703837313768,1.72304647947545));
#26888=CARTESIAN_POINT('Ctrl Pts',(-50.3334388281384,2.58279976746683,3.36592648157085));
#26889=CARTESIAN_POINT('Ctrl Pts',(-50.2145298291435,0.660936291289855,
4.19088044882765));
#26890=CARTESIAN_POINT('Ctrl Pts',(-50.0956208301485,-1.42153586209668,
3.99744312162439));
#26891=CARTESIAN_POINT('Ctrl Pts',(-49.9767118311536,-3.15857230942583,
2.83262010934112));
#26892=CARTESIAN_POINT('Ctrl Pts',(-49.8789006647461,-3.9560537057885,1.30826769936161));
#26893=CARTESIAN_POINT('Ctrl Pts',(-49.8207258313369,-4.07021487211157,
0.316179857216054));
#26894=CARTESIAN_POINT('Ctrl Pts',(-49.8021873309261,-4.07016024360026,
2.01151063877747E-5));
#26895=CARTESIAN_POINT('Origin',(41.25,0.,0.));
#26896=CARTESIAN_POINT('',(30.4838415259036,-4.92503358063389,0.00012643715616531));
#26897=CARTESIAN_POINT('',(30.2661584740964,-4.92498881568011,8.60120194096941E-5));
#26898=CARTESIAN_POINT('',(41.25,-4.925,-6.03138548580071E-16));
#26899=CARTESIAN_POINT('',(30.,2.16839587231054,4.42195480991683));
#26900=CARTESIAN_POINT('Ctrl Pts',(30.4838415259036,-4.92503358063389,0.00012643715616531));
#26901=CARTESIAN_POINT('Ctrl Pts',(30.4752030795814,-4.92521674395344,0.178328850711965));
#26902=CARTESIAN_POINT('Ctrl Pts',(30.4665646332593,-4.91573150459355,0.356511818192306));
#26903=CARTESIAN_POINT('Ctrl Pts',(30.4579261869371,-4.89642930393968,0.533624834627407));
#26904=CARTESIAN_POINT('Ctrl Pts',(30.4182898539388,-4.80786378831494,1.34628375915699));
#26905=CARTESIAN_POINT('Ctrl Pts',(30.3786535209405,-4.51262099257391,2.1364169177937));
#26906=CARTESIAN_POINT('Ctrl Pts',(30.3390171879422,-4.04657309347359,2.80802694357323));
#26907=CARTESIAN_POINT('Ctrl Pts',(30.2993808549439,-3.58052519437327,3.47963696935275));
#26908=CARTESIAN_POINT('Ctrl Pts',(30.2597445219455,-2.94367219191368,4.0327238622751));
#26909=CARTESIAN_POINT('Ctrl Pts',(30.2201081889472,-2.21339244687115,4.40007809567974));
#26910=CARTESIAN_POINT('Ctrl Pts',(30.1804718559489,-1.48311270182864,4.76743232908437));
#26911=CARTESIAN_POINT('Ctrl Pts',(30.1408355229506,-0.659406214203193,
4.94905390297128));
#26912=CARTESIAN_POINT('Ctrl Pts',(30.1011991899523,0.157646280266308,4.92289355924806));
#26913=CARTESIAN_POINT('Ctrl Pts',(30.0674661266348,0.853010393055609,4.90062942771858));
#26914=CARTESIAN_POINT('Ctrl Pts',(30.0337330633174,1.54355495045357,4.72786672521511));
#26915=CARTESIAN_POINT('Ctrl Pts',(30.,2.16858287139683,4.42210505377544));
#26916=CARTESIAN_POINT('',(30.,-2.1683958723106,4.4219548099168));
#26917=CARTESIAN_POINT('Origin',(30.,0.,0.));
#26918=CARTESIAN_POINT('Ctrl Pts',(30.,-2.16839587231058,4.42195480991681));
#26919=CARTESIAN_POINT('Ctrl Pts',(30.0396363329983,-2.90256543874867,4.06193976546855));
#26920=CARTESIAN_POINT('Ctrl Pts',(30.0792726659967,-3.54497553128948,3.51573257344795));
#26921=CARTESIAN_POINT('Ctrl Pts',(30.118908998995,-4.01781928837785,2.8490123239199));
#26922=CARTESIAN_POINT('Ctrl Pts',(30.1585453319933,-4.49066304546624,2.18229207439182));
#26923=CARTESIAN_POINT('Ctrl Pts',(30.1981816649916,-4.79394046710217,1.39505876735627));
#26924=CARTESIAN_POINT('Ctrl Pts',(30.2378179979899,-4.89076229523027,0.583305050522158));
#26925=CARTESIAN_POINT('Ctrl Pts',(30.2472648233587,-4.91383856977503,0.38983368157004));
#26926=CARTESIAN_POINT('Ctrl Pts',(30.2567116487276,-4.92518718095595,0.194969436276938));
#26927=CARTESIAN_POINT('Ctrl Pts',(30.2661584740964,-4.92498881568011,8.60120194096941E-5));
#26928=CARTESIAN_POINT('Origin',(41.25,0.,0.));
#26929=CARTESIAN_POINT('',(31.9838415259036,-4.92516276786698,-0.000113722890940915));
#26930=CARTESIAN_POINT('',(31.7661584740964,-4.9252122991162,-0.000105349299657425));
#26931=CARTESIAN_POINT('',(41.25,-4.925,-6.03138548580071E-16));
#26932=CARTESIAN_POINT('Ctrl Pts',(31.9838415259036,-4.92516276786698,-0.000113722890940915));
#26933=CARTESIAN_POINT('Ctrl Pts',(31.9508390755613,-4.92448958453899,0.680641938350505));
#26934=CARTESIAN_POINT('Ctrl Pts',(31.917836625219,-4.78214555510203,1.36167034280227));
#26935=CARTESIAN_POINT('Ctrl Pts',(31.8848341748767,-4.50788725221071,1.9846227453206));
#26936=CARTESIAN_POINT('Ctrl Pts',(31.8451978418784,-4.17849978830403,2.73279594495346));
#26937=CARTESIAN_POINT('Ctrl Pts',(31.80556150888,-3.65883529870816,3.39719861223649));
#26938=CARTESIAN_POINT('Ctrl Pts',(31.7659251758817,-3.012033474306,3.8971052419689));
#26939=CARTESIAN_POINT('Ctrl Pts',(31.7262888428834,-2.36523164990384,4.39701187170132));
#26940=CARTESIAN_POINT('Ctrl Pts',(31.6866525098851,-1.59129249069541,4.73242246388312));
#26941=CARTESIAN_POINT('Ctrl Pts',(31.6470161768868,-0.784250282821528,
4.86258433535561));
#26942=CARTESIAN_POINT('Ctrl Pts',(31.6073798438885,0.0227919250523556,
4.99274620682809));
#26943=CARTESIAN_POINT('Ctrl Pts',(31.5677435108901,0.862937181591687,4.91765935759125));
#26944=CARTESIAN_POINT('Ctrl Pts',(31.5281071778918,1.63410710193199,4.64644691014962));
#26945=CARTESIAN_POINT('Ctrl Pts',(31.4884708448935,2.40527702227229,4.37523446270799));
#26946=CARTESIAN_POINT('Ctrl Pts',(31.4488345118952,3.10747160641356,3.90789641706156));
#26947=CARTESIAN_POINT('Ctrl Pts',(31.4091981788969,3.65537359683798,3.301214746304));
#26948=CARTESIAN_POINT('Ctrl Pts',(31.3695618458985,4.2032755872624,2.69453307554644));
#26949=CARTESIAN_POINT('Ctrl Pts',(31.3299255129002,4.59688498396996,1.94850777967776));
#26950=CARTESIAN_POINT('Ctrl Pts',(31.2902891799019,4.78837790063976,1.15378160391619));
#26951=CARTESIAN_POINT('Ctrl Pts',(31.2506528469036,4.97987081730956,0.35905542815461));
#26952=CARTESIAN_POINT('Ctrl Pts',(31.2110165139052,4.9692472539416,-0.484371627499863));
#26953=CARTESIAN_POINT('Ctrl Pts',(31.1713801809069,4.75779798214507,-1.27402247248995));
#26954=CARTESIAN_POINT('Ctrl Pts',(31.1317438479086,4.54634871034855,-2.06367331748002));
#26955=CARTESIAN_POINT('Ctrl Pts',(31.0921075149103,4.13407373012347,-2.79954795180571));
#26956=CARTESIAN_POINT('Ctrl Pts',(31.052471181912,3.57106481416884,-3.39223689097617));
#26957=CARTESIAN_POINT('Ctrl Pts',(31.0128348489136,3.00805589821421,-3.98492583014663));
#26958=CARTESIAN_POINT('Ctrl Pts',(30.9731985159153,2.29431304653003,-4.43442907416186));
#26959=CARTESIAN_POINT('Ctrl Pts',(30.933562182917,1.516556638511,-4.68613172760538));
#26960=CARTESIAN_POINT('Ctrl Pts',(30.8939258499187,0.738800230491954,-4.9378343810489));
#26961=CARTESIAN_POINT('Ctrl Pts',(30.8542895169203,-0.102969733861949,
-4.99173644392069));
#26962=CARTESIAN_POINT('Ctrl Pts',(30.814653183922,-0.906477461021434,-4.84128848378581));
#26963=CARTESIAN_POINT('Ctrl Pts',(30.7750168509237,-1.70998518818092,-4.69084052365093));
#26964=CARTESIAN_POINT('Ctrl Pts',(30.7353805179254,-2.47523067814598,-4.33604254050938));
#26965=CARTESIAN_POINT('Ctrl Pts',(30.6957441849271,-3.10923594354023,-3.82000336783515));
#26966=CARTESIAN_POINT('Ctrl Pts',(30.6561078519288,-3.74324120893447,-3.30396419516092));
#26967=CARTESIAN_POINT('Ctrl Pts',(30.6164715189305,-4.24600624975789,-2.62668383295402));
#26968=CARTESIAN_POINT('Ctrl Pts',(30.5768351859321,-4.55644465241538,-1.87045130663933));
#26969=CARTESIAN_POINT('Ctrl Pts',(30.5458372992559,-4.799225295769,-1.27903407960837));
#26970=CARTESIAN_POINT('Ctrl Pts',(30.5148394125798,-4.92437632403811,-0.639328623954206));
#26971=CARTESIAN_POINT('Ctrl Pts',(30.4838415259036,-4.92503358063389,0.00012643715616531));
#26972=CARTESIAN_POINT('Ctrl Pts',(30.2661584740964,-4.92498881568011,8.60120194096941E-5));
#26973=CARTESIAN_POINT('Ctrl Pts',(30.2963479817259,-4.92435489372491,-0.622708884020471));
#26974=CARTESIAN_POINT('Ctrl Pts',(30.3265374893554,-4.80579524376599,-1.24569964894004));
#26975=CARTESIAN_POINT('Ctrl Pts',(30.3567269969849,-4.57520694706496,-1.82405290111985));
#26976=CARTESIAN_POINT('Ctrl Pts',(30.3963633299832,-4.27246353615129,-2.58338300929506));
#26977=CARTESIAN_POINT('Ctrl Pts',(30.4359996629815,-3.77661047970369,-3.26576909901281));
#26978=CARTESIAN_POINT('Ctrl Pts',(30.4756359959799,-3.14788147849495,-3.78823036846191));
#26979=CARTESIAN_POINT('Ctrl Pts',(30.5152723289782,-2.51915247728621,-4.31069163791102));
#26980=CARTESIAN_POINT('Ctrl Pts',(30.5549086619765,-1.75754753131633,-4.6732280870915));
#26981=CARTESIAN_POINT('Ctrl Pts',(30.5945449949748,-0.955608781264278,
-4.83182630983855));
#26982=CARTESIAN_POINT('Ctrl Pts',(30.6341813279731,-0.153670031212227,
-4.99042453258561));
#26983=CARTESIAN_POINT('Ctrl Pts',(30.6738176609715,0.688602522921993,-4.94508452889924));
#26984=CARTESIAN_POINT('Ctrl Pts',(30.7134539939698,1.46887527262288,-4.70129757355756));
#26985=CARTESIAN_POINT('Ctrl Pts',(30.7530903269681,2.24914802232376,-4.45751061821589));
#26986=CARTESIAN_POINT('Ctrl Pts',(30.7927266599664,2.96742096759131,-4.01527671121891));
#26987=CARTESIAN_POINT('Ctrl Pts',(30.8323629929647,3.53642168974787,-3.4283364671891));
#26988=CARTESIAN_POINT('Ctrl Pts',(30.871999325963,4.10542241190442,-2.84139622315928));
#26989=CARTESIAN_POINT('Ctrl Pts',(30.9116356589614,4.52515091094998,-2.10974964209663));
#26990=CARTESIAN_POINT('Ctrl Pts',(30.9512719919597,4.74461062149402,-1.32228801091272));
#26991=CARTESIAN_POINT('Ctrl Pts',(30.990908324958,4.96407033203805,-0.534826379728812));
#26992=CARTESIAN_POINT('Ctrl Pts',(31.0305446579563,4.98326125408056,0.308450301576346));
#26993=CARTESIAN_POINT('Ctrl Pts',(31.0701809909546,4.79985126528465,1.10508096512556));
#26994=CARTESIAN_POINT('Ctrl Pts',(31.109817323953,4.61644127648874,1.90171162867477));
#26995=CARTESIAN_POINT('Ctrl Pts',(31.1494536569513,4.23043037685442,2.65169627446803));
#26996=CARTESIAN_POINT('Ctrl Pts',(31.1890899899496,3.68871943369624,3.26391221939412));
#26997=CARTESIAN_POINT('Ctrl Pts',(31.2287263229479,3.14700849053805,3.87612816432021));
#26998=CARTESIAN_POINT('Ctrl Pts',(31.2683626559463,2.44959750385601,4.35057540837914));
#26999=CARTESIAN_POINT('Ctrl Pts',(31.3079989889446,1.68122241712191,4.62960764002769));
#27000=CARTESIAN_POINT('Ctrl Pts',(31.3476353219429,0.912847330387817,4.90863987167623));
#27001=CARTESIAN_POINT('Ctrl Pts',(31.3872716549412,0.0735081436016706,
4.99225709091441));
#27002=CARTESIAN_POINT('Ctrl Pts',(31.4269079879395,-0.734814645052458,
4.87030001077229));
#27003=CARTESIAN_POINT('Ctrl Pts',(31.4665443209378,-1.54313743370658,4.74834293063017));
#27004=CARTESIAN_POINT('Ctrl Pts',(31.5061806539362,-2.32044382422869,4.42081155110776));
#27005=CARTESIAN_POINT('Ctrl Pts',(31.5458169869345,-2.97229043473293,3.9275010823073));
#27006=CARTESIAN_POINT('Ctrl Pts',(31.5854533199328,-3.62413704523717,3.43419061350684));
#27007=CARTESIAN_POINT('Ctrl Pts',(31.6250896529311,-4.15052387572353,2.77510105542834));
#27008=CARTESIAN_POINT('Ctrl Pts',(31.6647259859294,-4.48749445206432,2.03031243692023));
#27009=CARTESIAN_POINT('Ctrl Pts',(31.6985368153184,-4.774939172701,1.39498825311397));
#27010=CARTESIAN_POINT('Ctrl Pts',(31.7323476447074,-4.92455446478589,0.697304835250864));
#27011=CARTESIAN_POINT('Ctrl Pts',(31.7661584740964,-4.9252122991162,-0.000105349299657425));
#27012=CARTESIAN_POINT('Origin',(41.25,0.,0.));
#27013=CARTESIAN_POINT('',(33.4838415259036,-4.9246005781677,3.93170949294919E-5));
#27014=CARTESIAN_POINT('',(33.2661584740964,-4.9245889324042,2.43377721320041E-5));
#27015=CARTESIAN_POINT('',(41.25,-4.925,-6.03138548580071E-16));
#27016=CARTESIAN_POINT('Ctrl Pts',(33.4838415259036,-4.9246005781677,3.93170949294919E-5));
#27017=CARTESIAN_POINT('Ctrl Pts',(33.4661114045395,-4.92470299465183,0.365886073899998));
#27018=CARTESIAN_POINT('Ctrl Pts',(33.4483812831753,-4.88447436734275,0.731710654126898));
#27019=CARTESIAN_POINT('Ctrl Pts',(33.4306511618112,-4.80367402952791,1.08834311566542));
#27020=CARTESIAN_POINT('Ctrl Pts',(33.3910148288129,-4.62304192722966,1.88560799125441));
#27021=CARTESIAN_POINT('Ctrl Pts',(33.3513784958145,-4.23964769810467,2.63693412006481));
#27022=CARTESIAN_POINT('Ctrl Pts',(33.3117421628162,-3.70007407698625,3.25103471900744));
#27023=CARTESIAN_POINT('Ctrl Pts',(33.2721058298179,-3.16050045586783,3.86513531795008));
#27024=CARTESIAN_POINT('Ctrl Pts',(33.2324694968196,-2.46474744275599,4.34201038702495));
#27025=CARTESIAN_POINT('Ctrl Pts',(33.1928331638213,-1.69734963847986,4.62371918742141));
#27026=CARTESIAN_POINT('Ctrl Pts',(33.153196830823,-0.92995183420373,4.90542798781788));
#27027=CARTESIAN_POINT('Ctrl Pts',(33.1135604978246,-0.0909092387633235,
4.99197051953595));
#27028=CARTESIAN_POINT('Ctrl Pts',(33.0739241648263,0.717833737184807,4.87283178912815));
#27029=CARTESIAN_POINT('Ctrl Pts',(33.034287831828,1.52657671313293,4.75369305872036));
#27030=CARTESIAN_POINT('Ctrl Pts',(32.9946514988297,2.30502006958878,4.4288730661867));
#27031=CARTESIAN_POINT('Ctrl Pts',(32.9550151658313,2.95858225653972,3.93783772528318));
#27032=CARTESIAN_POINT('Ctrl Pts',(32.915378832833,3.61214444349066,3.44680238437967));
#27033=CARTESIAN_POINT('Ctrl Pts',(32.8757424998347,4.14082546093669,2.78955169510629));
#27034=CARTESIAN_POINT('Ctrl Pts',(32.8361061668364,4.48039010193867,2.04594219220132));
#27035=CARTESIAN_POINT('Ctrl Pts',(32.7964698338381,4.81995474294064,1.30233268929635));
#27036=CARTESIAN_POINT('Ctrl Pts',(32.7568335008397,4.97040300749856,0.472364372759784));
#27037=CARTESIAN_POINT('Ctrl Pts',(32.7171971678414,4.91345529962058,-0.34312087958652));
#27038=CARTESIAN_POINT('Ctrl Pts',(32.6775608348431,4.8565075917426,-1.15860613193281));
#27039=CARTESIAN_POINT('Ctrl Pts',(32.6379245018448,4.59216391142874,-1.95960832008884));
#27040=CARTESIAN_POINT('Ctrl Pts',(32.5982881688465,4.15254224749944,-2.64880497622958));
#27041=CARTESIAN_POINT('Ctrl Pts',(32.5586518358482,3.71292058357014,-3.33800163237032));
#27042=CARTESIAN_POINT('Ctrl Pts',(32.5190155028498,3.09802093602541,-3.91539275649576));
#27043=CARTESIAN_POINT('Ctrl Pts',(32.4793791698515,2.38255415092096,-4.3108248209992));
#27044=CARTESIAN_POINT('Ctrl Pts',(32.4397428368532,1.66708736581652,-4.70625688550265));
#27045=CARTESIAN_POINT('Ctrl Pts',(32.4001065038549,0.851053443152359,-4.9197298903841));
#27046=CARTESIAN_POINT('Ctrl Pts',(32.3604701708566,0.0336012196779929,
-4.9253066785054));
#27047=CARTESIAN_POINT('Ctrl Pts',(32.3208338378582,-0.783851003796368,
-4.93088346662671));
#27048=CARTESIAN_POINT('Ctrl Pts',(32.2811975048599,-1.60272152808094,-4.72856403798788));
#27049=CARTESIAN_POINT('Ctrl Pts',(32.2415611718616,-2.32351686684147,-4.34293038040315));
#27050=CARTESIAN_POINT('Ctrl Pts',(32.2019248388633,-3.04431220560201,-3.95729672281842));
#27051=CARTESIAN_POINT('Ctrl Pts',(32.1622885058649,-3.66703235883851,-3.3883488362878));
#27052=CARTESIAN_POINT('Ctrl Pts',(32.1226521728666,-4.11601628220298,-2.7052143877759));
#27053=CARTESIAN_POINT('Ctrl Pts',(32.0830158398683,-4.56500020556745,-2.022079939264));
#27054=CARTESIAN_POINT('Ctrl Pts',(32.04337950687,-4.84024789905989,-1.22475892877083));
#27055=CARTESIAN_POINT('Ctrl Pts',(32.0037431738716,-4.90831652669737,-0.410126557532889));
#27056=CARTESIAN_POINT('Ctrl Pts',(31.9971092912156,-4.91970908635527,-0.273782573370168));
#27057=CARTESIAN_POINT('Ctrl Pts',(31.9904754085596,-4.92529808567392,-0.136953658327863));
#27058=CARTESIAN_POINT('Ctrl Pts',(31.9838415259036,-4.92516276786698,-0.000113722890940915));
#27059=CARTESIAN_POINT('Ctrl Pts',(31.7661584740964,-4.9252122991162,-0.000105349299657425));
#27060=CARTESIAN_POINT('Ctrl Pts',(31.7719839777057,-4.92532564198105,-0.12026701408908));
#27061=CARTESIAN_POINT('Ctrl Pts',(31.7778094813151,-4.92101699689922,-0.24042056760678));
#27062=CARTESIAN_POINT('Ctrl Pts',(31.7836349849244,-4.91222944566371,-0.360245654138465));
#27063=CARTESIAN_POINT('Ctrl Pts',(31.8232713179227,-4.85243954072709,-1.17552744775133));
#27064=CARTESIAN_POINT('Ctrl Pts',(31.862907650921,-4.58530540865863,-1.97560335603935));
#27065=CARTESIAN_POINT('Ctrl Pts',(31.9025439839194,-4.14328407736884,-2.66326343741845));
#27066=CARTESIAN_POINT('Ctrl Pts',(31.9421803169177,-3.70126274607906,-3.35092351879755));
#27067=CARTESIAN_POINT('Ctrl Pts',(31.981816649916,-3.08435421556795,-3.92616777326773));
#27068=CARTESIAN_POINT('Ctrl Pts',(32.0214529829144,-2.36751341455751,-4.31910352858822));
#27069=CARTESIAN_POINT('Ctrl Pts',(32.0610893159127,-1.65067261354707,-4.7120392839087));
#27070=CARTESIAN_POINT('Ctrl Pts',(32.100725648911,-0.833899542037295,-4.9226665400795));
#27071=CARTESIAN_POINT('Ctrl Pts',(32.1403619819093,-0.0164328431961262,
-4.92539389647684));
#27072=CARTESIAN_POINT('Ctrl Pts',(32.1799983149076,0.801033855645048,-4.92812125287418));
#27073=CARTESIAN_POINT('Ctrl Pts',(32.2196346479059,1.61919418181762,-4.72294870949805));
#27074=CARTESIAN_POINT('Ctrl Pts',(32.2592709809043,2.33864093827332,-4.33480491238653));
#27075=CARTESIAN_POINT('Ctrl Pts',(32.2989073139026,3.05808769472903,-3.946661115275));
#27076=CARTESIAN_POINT('Ctrl Pts',(32.3385436469009,3.67882088146788,-3.37554606442807));
#27077=CARTESIAN_POINT('Ctrl Pts',(32.3781799798992,4.1254208725147,-2.69085073792278));
#27078=CARTESIAN_POINT('Ctrl Pts',(32.4178163128976,4.57202086356151,-2.0061554114175));
#27079=CARTESIAN_POINT('Ctrl Pts',(32.4574526458959,4.84448765891629,-1.20787980925385));
#27080=CARTESIAN_POINT('Ctrl Pts',(32.4970889788942,4.90971630405955,-0.39301511723372));
#27081=CARTESIAN_POINT('Ctrl Pts',(32.5367253118925,4.9749449492028,0.421849574786424));
#27082=CARTESIAN_POINT('Ctrl Pts',(32.5763616448908,4.83293544413453,1.25330335666306));
#27083=CARTESIAN_POINT('Ctrl Pts',(32.6159979778891,4.50094206822459,2.00032386551657));
#27084=CARTESIAN_POINT('Ctrl Pts',(32.6556343108875,4.16894869231465,2.74734437437008));
#27085=CARTESIAN_POINT('Ctrl Pts',(32.6952706438858,3.64697144556304,3.40993161020045));
#27086=CARTESIAN_POINT('Ctrl Pts',(32.7349069768841,2.99843102086877,3.90758064304421));
#27087=CARTESIAN_POINT('Ctrl Pts',(32.7745433098824,2.34989059617449,4.40522967588796));
#27088=CARTESIAN_POINT('Ctrl Pts',(32.8141796428808,1.57478699353755,4.73794050574509));
#27089=CARTESIAN_POINT('Ctrl Pts',(32.8538159758791,0.767295979967659,4.86528847528057));
#27090=CARTESIAN_POINT('Ctrl Pts',(32.8934523088774,-0.0401950336022416,
4.99263644481604));
#27091=CARTESIAN_POINT('Ctrl Pts',(32.9330886418757,-0.880073458105095,
4.91462155402985));
#27092=CARTESIAN_POINT('Ctrl Pts',(32.972724974874,-1.65029332892724,4.64072268048729));
#27093=CARTESIAN_POINT('Ctrl Pts',(33.0123613078724,-2.42051319974939,4.36682380694472));
#27094=CARTESIAN_POINT('Ctrl Pts',(33.0519976408707,-3.12107451689084,3.89704095064578));
#27095=CARTESIAN_POINT('Ctrl Pts',(33.091633973869,-3.66685846636575,3.28845314035125));
#27096=CARTESIAN_POINT('Ctrl Pts',(33.1312703068673,-4.21264241584066,2.67986533005673));
#27097=CARTESIAN_POINT('Ctrl Pts',(33.1709066398656,-4.60364899764904,1.93247256576663));
#27098=CARTESIAN_POINT('Ctrl Pts',(33.210542972864,-4.79237056943692,1.13708372332491));
#27099=CARTESIAN_POINT('Ctrl Pts',(33.2290814732748,-4.8806384456874,0.765068572907586));
#27100=CARTESIAN_POINT('Ctrl Pts',(33.2476199736856,-4.92465502880973,0.382553937021347));
#27101=CARTESIAN_POINT('Ctrl Pts',(33.2661584740964,-4.9245889324042,2.43377721320041E-5));
#27102=CARTESIAN_POINT('Origin',(41.25,0.,0.));
#27103=CARTESIAN_POINT('',(34.9838415259036,-4.92537655231972,5.17146673368989E-5));
#27104=CARTESIAN_POINT('',(34.7661584740964,-4.92534558823064,6.69665182562415E-5));
#27105=CARTESIAN_POINT('',(41.25,-4.925,-6.03138548580071E-16));
#27106=CARTESIAN_POINT('Ctrl Pts',(34.9838415259036,-4.92537655231972,5.17146673368989E-5));
#27107=CARTESIAN_POINT('Ctrl Pts',(34.9813837335176,-4.92540394102758,0.0507432790454098));
#27108=CARTESIAN_POINT('Ctrl Pts',(34.9789259411317,-4.9246376068758,0.101434013757565));
#27109=CARTESIAN_POINT('Ctrl Pts',(34.9764681487457,-4.92307226133183,0.15210006272951));
#27110=CARTESIAN_POINT('Ctrl Pts',(34.9368318157474,-4.89782824251546,0.969181440404085));
#27111=CARTESIAN_POINT('Ctrl Pts',(34.8971954827491,-4.66478232121914,1.77984270463634));
#27112=CARTESIAN_POINT('Ctrl Pts',(34.8575591497507,-4.25224978111449,2.48558780138401));
#27113=CARTESIAN_POINT('Ctrl Pts',(34.8179228167524,-3.83971724100984,3.19133289813169));
#27114=CARTESIAN_POINT('Ctrl Pts',(34.7782864837541,-3.24769808209686,3.7921618273948));
#27115=CARTESIAN_POINT('Ctrl Pts',(34.7386501507558,-2.54812315101044,4.21507334772028));
#27116=CARTESIAN_POINT('Ctrl Pts',(34.6990138177575,-1.84854821992401,4.63798486804578));
#27117=CARTESIAN_POINT('Ctrl Pts',(34.6593774847591,-1.04141751666414,4.88297897943365));
#27118=CARTESIAN_POINT('Ctrl Pts',(34.6197411517608,-0.224798129020873,
4.92028868264515));
#27119=CARTESIAN_POINT('Ctrl Pts',(34.5801048187625,0.591821258622399,4.95759838585665));
#27120=CARTESIAN_POINT('Ctrl Pts',(34.5404684857642,1.41792933064908,4.78722368089177));
#27121=CARTESIAN_POINT('Ctrl Pts',(34.5008321527659,2.15315323233279,4.42986524371477));
#27122=CARTESIAN_POINT('Ctrl Pts',(34.4611958197675,2.88837713401649,4.07250680653778));
#27123=CARTESIAN_POINT('Ctrl Pts',(34.4215594867692,3.53271686535722,3.52816463714868));
#27124=CARTESIAN_POINT('Ctrl Pts',(34.3819231537709,4.00788458431802,2.8629767861726));
#27125=CARTESIAN_POINT('Ctrl Pts',(34.3422868207726,4.48305230327882,2.19778893519652));
#27126=CARTESIAN_POINT('Ctrl Pts',(34.3026504877742,4.78904800985969,1.41175540263347));
#27127=CARTESIAN_POINT('Ctrl Pts',(34.2630141547759,4.88869295754603,0.600379951544906));
#27128=CARTESIAN_POINT('Ctrl Pts',(34.2233778217776,4.98833790523238,-0.210995499543657));
#27129=CARTESIAN_POINT('Ctrl Pts',(34.1837414887793,4.8816320940242,-1.04771286915773));
#27130=CARTESIAN_POINT('Ctrl Pts',(34.144105155781,4.58154037349691,-1.80811026361641));
#27131=CARTESIAN_POINT('Ctrl Pts',(34.1044688227826,4.28144865296962,-2.5685076580751));
#27132=CARTESIAN_POINT('Ctrl Pts',(34.0648324897843,3.78797102312322,-3.2525850773784));
#27133=CARTESIAN_POINT('Ctrl Pts',(34.025196156786,3.16106544845231,-3.77722651557704));
#27134=CARTESIAN_POINT('Ctrl Pts',(33.9855598237877,2.5341598737814,-4.30186795377567));
#27135=CARTESIAN_POINT('Ctrl Pts',(33.9459234907894,1.77382635428599,-4.66707341086963));
#27136=CARTESIAN_POINT('Ctrl Pts',(33.906287157791,0.972446078917145,-4.82847010376744));
#27137=CARTESIAN_POINT('Ctrl Pts',(33.8666508247927,0.171065803548301,-4.98986679666524));
#27138=CARTESIAN_POINT('Ctrl Pts',(33.8270144917944,-0.671361227693977,
-4.94745472536688));
#27139=CARTESIAN_POINT('Ctrl Pts',(33.7873781587961,-1.4524793922372,-4.70638699370371));
#27140=CARTESIAN_POINT('Ctrl Pts',(33.7477418257978,-2.23359755678042,-4.46531926204055));
#27141=CARTESIAN_POINT('Ctrl Pts',(33.7081054927994,-2.95340685462458,-4.02559587001259));
#27142=CARTESIAN_POINT('Ctrl Pts',(33.6684691598011,-3.5244498252634,-3.44064359511096));
#27143=CARTESIAN_POINT('Ctrl Pts',(33.6288328268028,-4.09549279590221,-2.85569132020933));
#27144=CARTESIAN_POINT('Ctrl Pts',(33.5891964938045,-4.51776943933568,-2.12551016243403));
#27145=CARTESIAN_POINT('Ctrl Pts',(33.5495601608062,-4.73997277331667,-1.33881777236259));
#27146=CARTESIAN_POINT('Ctrl Pts',(33.527653949172,-4.86278012939111,-0.904028560438227));
#27147=CARTESIAN_POINT('Ctrl Pts',(33.5057477375378,-4.92447403886602,-0.451977694839747));
#27148=CARTESIAN_POINT('Ctrl Pts',(33.4838415259036,-4.9246005781677,3.93170949294919E-5));
#27149=CARTESIAN_POINT('Ctrl Pts',(33.2661584740964,-4.9245889324042,2.43377721320041E-5));
#27150=CARTESIAN_POINT('Ctrl Pts',(33.2872563066839,-4.92451371106118,-0.435315375035468));
#27151=CARTESIAN_POINT('Ctrl Pts',(33.3083541392714,-4.86734396438128,-0.870674467928753));
#27152=CARTESIAN_POINT('Ctrl Pts',(33.3294519718589,-4.7533282243701,-1.29059903148261));
#27153=CARTESIAN_POINT('Ctrl Pts',(33.3690883048572,-4.53912774574801,-2.07950802325508));
#27154=CARTESIAN_POINT('Ctrl Pts',(33.4087246378556,-4.12429022673645,-2.81394108620665));
#27155=CARTESIAN_POINT('Ctrl Pts',(33.4483609708539,-3.55921878944626,-3.40466395955689));
#27156=CARTESIAN_POINT('Ctrl Pts',(33.4879973038522,-2.99414735215609,-3.99538683290712));
#27157=CARTESIAN_POINT('Ctrl Pts',(33.5276336368506,-2.2788419965873,-4.44239951665602));
#27158=CARTESIAN_POINT('Ctrl Pts',(33.5672699698489,-1.50021295031243,-4.69138957797913));
#27159=CARTESIAN_POINT('Ctrl Pts',(33.6069063028472,-0.721583904037545,
-4.94037963930225));
#27160=CARTESIAN_POINT('Ctrl Pts',(33.6465426358455,0.120368832943431,-4.99134707819958));
#27161=CARTESIAN_POINT('Ctrl Pts',(33.6861789688438,0.923347265226319,-4.83809930617939));
#27162=CARTESIAN_POINT('Ctrl Pts',(33.7258153018421,1.72632569750921,-4.6848515341592));
#27163=CARTESIAN_POINT('Ctrl Pts',(33.7654516348405,2.49032982509401,-4.32738855122149));
#27164=CARTESIAN_POINT('Ctrl Pts',(33.8050879678388,3.12253247693004,-3.80914242306223));
#27165=CARTESIAN_POINT('Ctrl Pts',(33.8447243008371,3.75473512876605,-3.29089629490298));
#27166=CARTESIAN_POINT('Ctrl Pts',(33.8843606338354,4.25513630485329,-2.61186702152217));
#27167=CARTESIAN_POINT('Ctrl Pts',(33.9239969668337,4.56293682376128,-1.85455725471561));
#27168=CARTESIAN_POINT('Ctrl Pts',(33.963633299832,4.87073734266926,-1.09724748790906));
#27169=CARTESIAN_POINT('Ctrl Pts',(34.0032696328304,4.985937204398,-0.261657227676774));
#27170=CARTESIAN_POINT('Ctrl Pts',(34.0429059658287,4.89453952478992,0.550688577078092));
#27171=CARTESIAN_POINT('Ctrl Pts',(34.082542298827,4.80314184518184,1.36303438183296));
#27172=CARTESIAN_POINT('Ctrl Pts',(34.1221786318253,4.50514662423694,2.1521357311104));
#27173=CARTESIAN_POINT('Ctrl Pts',(34.1618149648236,4.03676054245367,2.82211611942957));
#27174=CARTESIAN_POINT('Ctrl Pts',(34.201451297822,3.5683744606704,3.49209650774873));
#27175=CARTESIAN_POINT('Ctrl Pts',(34.2410876308203,2.92959751804876,4.04295593510963));
#27176=CARTESIAN_POINT('Ctrl Pts',(34.2807239638186,2.19804167292129,4.40776449833205));
#27177=CARTESIAN_POINT('Ctrl Pts',(34.3203602968169,1.4664858277938,4.77257306155448));
#27178=CARTESIAN_POINT('Ctrl Pts',(34.3599966298152,0.64215108016047,4.95133076063843));
#27179=CARTESIAN_POINT('Ctrl Pts',(34.3996329628136,-0.174805175720185,
4.92231837848757));
#27180=CARTESIAN_POINT('Ctrl Pts',(34.4392692958119,-0.991761431600829,
4.8933059963367));
#27181=CARTESIAN_POINT('Ctrl Pts',(34.4789056288102,-1.80133919572881,4.65652353295103));
#27182=CARTESIAN_POINT('Ctrl Pts',(34.5185419618085,-2.50517406027409,4.24074026514061));
#27183=CARTESIAN_POINT('Ctrl Pts',(34.5581782948069,-3.20900892481938,3.82495699733019));
#27184=CARTESIAN_POINT('Ctrl Pts',(34.5978146278052,-3.80710088978197,3.23017292509503));
#27185=CARTESIAN_POINT('Ctrl Pts',(34.6374509608035,-4.22678125726992,2.52865483446174));
#27186=CARTESIAN_POINT('Ctrl Pts',(34.6770872938018,-4.64646162475788,1.82713674382845));
#27187=CARTESIAN_POINT('Ctrl Pts',(34.7167236268002,-4.88773039477119,1.01888463479704));
#27188=CARTESIAN_POINT('Ctrl Pts',(34.7563599597985,-4.92127320031289,0.202101846941553));
#27189=CARTESIAN_POINT('Ctrl Pts',(34.7596261312311,-4.92403724393003,0.134796109842093));
#27190=CARTESIAN_POINT('Ctrl Pts',(34.7628923026638,-4.92539075926287,0.0674324466003896));
#27191=CARTESIAN_POINT('Ctrl Pts',(34.7661584740964,-4.92534558823064,6.69665182562415E-5));
#27192=CARTESIAN_POINT('Origin',(41.25,0.,0.));
#27193=CARTESIAN_POINT('',(36.4838415259036,-4.92478004438697,-0.000110922936420454));
#27194=CARTESIAN_POINT('',(36.2661584740964,-4.92482433489693,-0.000117749303896287));
#27195=CARTESIAN_POINT('',(41.25,-4.925,-6.03138548580071E-16));
#27196=CARTESIAN_POINT('Ctrl Pts',(36.4838415259036,-4.92478004438697,-0.000110922936420454));
#27197=CARTESIAN_POINT('Ctrl Pts',(36.4570197294975,-4.92432112113983,0.553277444647099));
#27198=CARTESIAN_POINT('Ctrl Pts',(36.4301979330913,-4.83122563981592,1.10681634663209));
#27199=CARTESIAN_POINT('Ctrl Pts',(36.4033761366852,-4.64828496666694,1.62887132335118));
#27200=CARTESIAN_POINT('Ctrl Pts',(36.3637398036869,-4.37794149935855,2.40034630539035));
#27201=CARTESIAN_POINT('Ctrl Pts',(36.3241034706886,-3.91139484670805,3.10306695234755));
#27202=CARTESIAN_POINT('Ctrl Pts',(36.2844671376903,-3.3053308358794,3.65165208977549));
#27203=CARTESIAN_POINT('Ctrl Pts',(36.244830804692,-2.69926682505073,4.20023722720345));
#27204=CARTESIAN_POINT('Ctrl Pts',(36.2051944716936,-1.95368545604391,4.59468685510214));
#27205=CARTESIAN_POINT('Ctrl Pts',(36.1655581386953,-1.15917551859725,4.78707499799849));
#27206=CARTESIAN_POINT('Ctrl Pts',(36.125921805697,-0.364665581150601,4.97946314089483));
#27207=CARTESIAN_POINT('Ctrl Pts',(36.0862854726987,0.478772924735871,4.96978979878885));
#27208=CARTESIAN_POINT('Ctrl Pts',(36.0466491397003,1.26866148143396,4.75923029122388));
#27209=CARTESIAN_POINT('Ctrl Pts',(36.007012806702,2.05855003813205,4.54867078365892));
#27210=CARTESIAN_POINT('Ctrl Pts',(35.9673764737037,2.79488864564176,4.13722511063498));
#27211=CARTESIAN_POINT('Ctrl Pts',(35.9277401407054,3.38821151784667,3.57488428200248));
#27212=CARTESIAN_POINT('Ctrl Pts',(35.8881038077071,3.98153439005161,3.01254345336996));
#27213=CARTESIAN_POINT('Ctrl Pts',(35.8484674747088,4.43184152695175,2.29930746912889));
#27214=CARTESIAN_POINT('Ctrl Pts',(35.8088311417104,4.6844202167787,1.52183512642213));
#27215=CARTESIAN_POINT('Ctrl Pts',(35.7691948087121,4.93699890660564,0.744362783715409));
#27216=CARTESIAN_POINT('Ctrl Pts',(35.7295584757138,4.99184914935941,-0.0973459174569996));
#27217=CARTESIAN_POINT('Ctrl Pts',(35.6899221427155,4.8423065924764,-0.901022632255597));
#27218=CARTESIAN_POINT('Ctrl Pts',(35.6502858097171,4.69276403559339,-1.7046993470542));
#27219=CARTESIAN_POINT('Ctrl Pts',(35.6106494767188,4.33882867907361,-2.470344075479));
#27220=CARTESIAN_POINT('Ctrl Pts',(35.5710131437205,3.82350397891201,-3.10493031203944));
#27221=CARTESIAN_POINT('Ctrl Pts',(35.5313768107222,3.3081792787504,-3.73951654859988));
#27222=CARTESIAN_POINT('Ctrl Pts',(35.4917404777239,2.63146523494698,-4.24304429329594));
#27223=CARTESIAN_POINT('Ctrl Pts',(35.4521041447255,1.87558319687476,-4.55433448387119));
#27224=CARTESIAN_POINT('Ctrl Pts',(35.4124678117272,1.11970115880254,-4.86562467444645));
#27225=CARTESIAN_POINT('Ctrl Pts',(35.3728314787289,0.28465112646151,-4.98467731090088));
#27226=CARTESIAN_POINT('Ctrl Pts',(35.3331951457306,-0.528107589407301,
-4.89702739357129));
#27227=CARTESIAN_POINT('Ctrl Pts',(35.2935588127323,-1.34086630527611,-4.8093774762417));
#27228=CARTESIAN_POINT('Ctrl Pts',(35.2539224797339,-2.13133370467271,-4.5150250051281));
#27229=CARTESIAN_POINT('Ctrl Pts',(35.2142861467356,-2.80346730582963,-4.04973406343202));
#27230=CARTESIAN_POINT('Ctrl Pts',(35.1746498137373,-3.47560090698655,-3.58444312173594));
#27231=CARTESIAN_POINT('Ctrl Pts',(35.135013480739,-4.0294007099038,-2.9482137094574));
#27232=CARTESIAN_POINT('Ctrl Pts',(35.0953771477407,-4.39757955319421,-2.21834825775968));
#27233=CARTESIAN_POINT('Ctrl Pts',(35.0581986071283,-4.74292815238131,-1.53374072005811));
#27234=CARTESIAN_POINT('Ctrl Pts',(35.0210200665159,-4.9249622487385,-0.766749580550754));
#27235=CARTESIAN_POINT('Ctrl Pts',(34.9838415259036,-4.92537655231972,5.17146673368989E-5));
#27236=CARTESIAN_POINT('Ctrl Pts',(34.7661584740964,-4.92534558823064,6.69665182562415E-5));
#27237=CARTESIAN_POINT('Ctrl Pts',(34.8025286356621,-4.92484259021781,-0.750075346909099));
#27238=CARTESIAN_POINT('Ctrl Pts',(34.8388987972277,-4.75090614755571,-1.50044294378959));
#27239=CARTESIAN_POINT('Ctrl Pts',(34.8752689587934,-4.41988712998175,-2.17356224361685));
#27240=CARTESIAN_POINT('Ctrl Pts',(34.9149052917917,-4.05914141303884,-2.90713007964017));
#27241=CARTESIAN_POINT('Ctrl Pts',(34.9545416247901,-3.51183313808295,-3.54895228500724));
#27242=CARTESIAN_POINT('Ctrl Pts',(34.9941779577884,-2.84446074016496,-4.02104689929317));
#27243=CARTESIAN_POINT('Ctrl Pts',(35.0338142907867,-2.17708834224698,-4.4931415135791));
#27244=CARTESIAN_POINT('Ctrl Pts',(35.073450623785,-1.3896518213669,-4.7955085367839));
#27245=CARTESIAN_POINT('Ctrl Pts',(35.1130869567833,-0.577825404896259,
-4.89141011060323));
#27246=CARTESIAN_POINT('Ctrl Pts',(35.1527232897817,0.234001011574379,-4.98731168442256));
#27247=CARTESIAN_POINT('Ctrl Pts',(35.19235962278,1.07021732363557,-4.87674780885642));
#27248=CARTESIAN_POINT('Ctrl Pts',(35.2319959557783,1.82922251653823,-4.57315209168081));
#27249=CARTESIAN_POINT('Ctrl Pts',(35.2716322887766,2.5882277094409,-4.26955637450519));
#27250=CARTESIAN_POINT('Ctrl Pts',(35.3112686217749,3.27002178318504,-3.77292881572008));
#27251=CARTESIAN_POINT('Ctrl Pts',(35.3509049547733,3.79176616030783,-3.14361009894666));
#27252=CARTESIAN_POINT('Ctrl Pts',(35.3905412877716,4.31351053743063,-2.51429138217323));
#27253=CARTESIAN_POINT('Ctrl Pts',(35.4301776207699,4.67520521793209,-1.75228150741147));
#27254=CARTESIAN_POINT('Ctrl Pts',(35.4698139537682,4.83290398115343,-0.950165342246432));
#27255=CARTESIAN_POINT('Ctrl Pts',(35.5094502867666,4.99060274437478,-0.148049177081417));
#27256=CARTESIAN_POINT('Ctrl Pts',(35.5490866197649,4.94430559031603,0.694173278486871));
#27257=CARTESIAN_POINT('Ctrl Pts',(35.5887229527632,4.6996376637687,1.47417125800964));
#27258=CARTESIAN_POINT('Ctrl Pts',(35.6283592857615,4.45496973722136,2.25416923753242));
#27259=CARTESIAN_POINT('Ctrl Pts',(35.6679956187598,4.01193103818541,2.97194274100968));
#27260=CARTESIAN_POINT('Ctrl Pts',(35.7076319517581,3.42435115685893,3.54028165873479));
#27261=CARTESIAN_POINT('Ctrl Pts',(35.7472682847565,2.83677127553244,4.1086205764599));
#27262=CARTESIAN_POINT('Ctrl Pts',(35.7869046177548,2.10465021191539,4.52752490843288));
#27263=CARTESIAN_POINT('Ctrl Pts',(35.8265409507531,1.31694131684514,4.74609741120441));
#27264=CARTESIAN_POINT('Ctrl Pts',(35.8661772837514,0.529232421774926,4.96466991397594));
#27265=CARTESIAN_POINT('Ctrl Pts',(35.9058136167498,-0.314064304748486,
4.98291058754604));
#27266=CARTESIAN_POINT('Ctrl Pts',(35.9454499497481,-1.1104875714138,4.7986031740904));
#27267=CARTESIAN_POINT('Ctrl Pts',(35.9850862827464,-1.90691083807915,4.61429576063476));
#27268=CARTESIAN_POINT('Ctrl Pts',(36.0247226157447,-2.65646064488639,4.22744026015335));
#27269=CARTESIAN_POINT('Ctrl Pts',(36.064358948743,-3.26806603342656,3.68503995498266));
#27270=CARTESIAN_POINT('Ctrl Pts',(36.1039952817413,-3.8796714219667,3.142639649812));
#27271=CARTESIAN_POINT('Ctrl Pts',(36.1436316147397,-4.35333239223978,2.44469453995207));
#27272=CARTESIAN_POINT('Ctrl Pts',(36.183267947738,-4.63149872125605,1.67600556790799));
#27273=CARTESIAN_POINT('Ctrl Pts',(36.2108981231908,-4.82540627764142,1.14015854171839));
#27274=CARTESIAN_POINT('Ctrl Pts',(36.2385282986436,-4.92431567132321,0.569934425257451));
#27275=CARTESIAN_POINT('Ctrl Pts',(36.2661584740964,-4.92482433489693,-0.000117749303896287));
#27276=CARTESIAN_POINT('Origin',(41.25,0.,0.));
#27277=CARTESIAN_POINT('',(37.9838415259036,-4.92485067281264,0.000120817417613023));
#27278=CARTESIAN_POINT('',(37.7661584740964,-4.92480467811149,0.000114993715880741));
#27279=CARTESIAN_POINT('',(41.25,-4.925,-6.03138548580071E-16));
#27280=CARTESIAN_POINT('Ctrl Pts',(37.9838415259036,-4.92485067281264,0.000120817417613023));
#27281=CARTESIAN_POINT('Ctrl Pts',(37.9722920584757,-4.92507066765589,0.238400081367369));
#27282=CARTESIAN_POINT('Ctrl Pts',(37.9607425910477,-4.9080872440668,0.476648253950855));
#27283=CARTESIAN_POINT('Ctrl Pts',(37.9491931236198,-4.87363741638938,0.712343491708345));
#27284=CARTESIAN_POINT('Ctrl Pts',(37.9095567906214,-4.75540990069872,1.52122017698863));
#27285=CARTESIAN_POINT('Ctrl Pts',(37.8699204576231,-4.43146711813237,2.30002898645485));
#27286=CARTESIAN_POINT('Ctrl Pts',(37.8302841246248,-3.94116839977733,2.9541439650625));
#27287=CARTESIAN_POINT('Ctrl Pts',(37.7906477916264,-3.45086968142229,3.60825894367013));
#27288=CARTESIAN_POINT('Ctrl Pts',(37.7510114586281,-2.79421502727857,4.13768009141919));
#27289=CARTESIAN_POINT('Ctrl Pts',(37.7113751256298,-2.05098855374135,4.47808227597847));
#27290=CARTESIAN_POINT('Ctrl Pts',(37.6717387926315,-1.30776208020412,4.81848446053774));
#27291=CARTESIAN_POINT('Ctrl Pts',(37.6321024596332,-0.477963787273387,
4.96986768190722));
#27292=CARTESIAN_POINT('Ctrl Pts',(37.5924661266349,0.337585105473864,4.9138387454774));
#27293=CARTESIAN_POINT('Ctrl Pts',(37.5528297936365,1.15313399822113,4.85780980904757));
#27294=CARTESIAN_POINT('Ctrl Pts',(37.5131934606382,1.95443349078488,4.59436871481845));
#27295=CARTESIAN_POINT('Ctrl Pts',(37.4735571276399,2.6441249924731,4.15552378688388));
#27296=CARTESIAN_POINT('Ctrl Pts',(37.4339207946416,3.33381649416131,3.71667885894933));
#27297=CARTESIAN_POINT('Ctrl Pts',(37.3942844616432,3.91190000497398,3.10243009730932));
#27298=CARTESIAN_POINT('Ctrl Pts',(37.3546481286449,4.30813787178923,2.38740926467432));
#27299=CARTESIAN_POINT('Ctrl Pts',(37.3150117956466,4.7043757386045,1.6723884320393));
#27300=CARTESIAN_POINT('Ctrl Pts',(37.2753754626483,4.91876796142238,0.856595528409254));
#27301=CARTESIAN_POINT('Ctrl Pts',(37.23573912965,4.92526569725575,0.0391501065792324));
#27302=CARTESIAN_POINT('Ctrl Pts',(37.1961027966516,4.93176343308912,-0.778295315250795));
#27303=CARTESIAN_POINT('Ctrl Pts',(37.1564664636533,4.730366681938,-1.59739325528078));
#27304=CARTESIAN_POINT('Ctrl Pts',(37.116830130655,4.34554532557911,-2.31862259599992));
#27305=CARTESIAN_POINT('Ctrl Pts',(37.0771937976567,3.96072396922023,-3.03985193671904));
#27306=CARTESIAN_POINT('Ctrl Pts',(37.0375574646584,3.39247800765361,-3.6632126781273));
#27307=CARTESIAN_POINT('Ctrl Pts',(36.99792113166,2.70984982319539,-4.11296594383257));
#27308=CARTESIAN_POINT('Ctrl Pts',(36.9582847986617,2.02722163873717,-4.56271920953783));
#27309=CARTESIAN_POINT('Ctrl Pts',(36.9186484656634,1.23021123138735,-4.8388649995401));
#27310=CARTESIAN_POINT('Ctrl Pts',(36.8790121326651,0.415656064117347,-4.90785135835727));
#27311=CARTESIAN_POINT('Ctrl Pts',(36.8393757996667,-0.398899103152658,
-4.97683771717445));
#27312=CARTESIAN_POINT('Ctrl Pts',(36.7997394666684,-1.23099903034286,-4.83866464480654));
#27313=CARTESIAN_POINT('Ctrl Pts',(36.7601031336701,-1.97954284707522,-4.51012029063243));
#27314=CARTESIAN_POINT('Ctrl Pts',(36.7204668006718,-2.7280866638076,-4.18157593645832));
#27315=CARTESIAN_POINT('Ctrl Pts',(36.6808304676735,-3.39307437008213,-3.662660300478));
#27316=CARTESIAN_POINT('Ctrl Pts',(36.6411941346751,-3.89370937681127,-3.01642208722661));
#27317=CARTESIAN_POINT('Ctrl Pts',(36.6015578016768,-4.39434438354041,-2.37018387397521));
#27318=CARTESIAN_POINT('Ctrl Pts',(36.5619214686785,-4.73062669072415,-1.59662308345274));
#27319=CARTESIAN_POINT('Ctrl Pts',(36.5222851356802,-4.86169770333288,-0.789728029630932));
#27320=CARTESIAN_POINT('Ctrl Pts',(36.509470599088,-4.90407332590429,-0.528856616685018));
#27321=CARTESIAN_POINT('Ctrl Pts',(36.4966560624958,-4.924999302212,-0.264500950312836));
#27322=CARTESIAN_POINT('Ctrl Pts',(36.4838415259036,-4.92478004438697,-0.000110922936420454));
#27323=CARTESIAN_POINT('Ctrl Pts',(36.2661584740964,-4.92482433489693,-0.000117749303896287));
#27324=CARTESIAN_POINT('Ctrl Pts',(36.2781646316419,-4.92504536480005,-0.247822879828381));
#27325=CARTESIAN_POINT('Ctrl Pts',(36.2901707891874,-4.90668667699816,-0.49549554482184));
#27326=CARTESIAN_POINT('Ctrl Pts',(36.3021769467329,-4.86946910202077,-0.740301109765489));
#27327=CARTESIAN_POINT('Ctrl Pts',(36.3418132797313,-4.74660146600976,-1.54848598116662));
#27328=CARTESIAN_POINT('Ctrl Pts',(36.3814496127296,-4.41819450622829,-2.32542288974066));
#27329=CARTESIAN_POINT('Ctrl Pts',(36.4210859457279,-3.92414995609534,-2.97671332021275));
#27330=CARTESIAN_POINT('Ctrl Pts',(36.4607222787263,-3.43010540596239,-3.62800375068483));
#27331=CARTESIAN_POINT('Ctrl Pts',(36.5003586117246,-2.77042326547796,-4.15364770305498));
#27332=CARTESIAN_POINT('Ctrl Pts',(36.5399949447229,-2.02525549283558,-4.48977897645243));
#27333=CARTESIAN_POINT('Ctrl Pts',(36.5796312777212,-1.28008772019321,-4.82591024984988));
#27334=CARTESIAN_POINT('Ctrl Pts',(36.6192676107195,-0.449434315392872,
-4.97252884427464));
#27335=CARTESIAN_POINT('Ctrl Pts',(36.6589039437178,0.365779604923634,-4.91182047201209));
#27336=CARTESIAN_POINT('Ctrl Pts',(36.6985402767162,1.18099352524016,-4.85111209974954));
#27337=CARTESIAN_POINT('Ctrl Pts',(36.7381766097145,1.98076796107286,-4.5830767607997));
#27338=CARTESIAN_POINT('Ctrl Pts',(36.7778129427128,2.66792961757094,-4.14028098374283));
#27339=CARTESIAN_POINT('Ctrl Pts',(36.8174492757111,3.35509127406902,-3.69748520668596));
#27340=CARTESIAN_POINT('Ctrl Pts',(36.8570856087094,3.92964015123248,-3.0799289915221));
#27341=CARTESIAN_POINT('Ctrl Pts',(36.8967219417078,4.32176805696933,-2.36264595960017));
#27342=CARTESIAN_POINT('Ctrl Pts',(36.9363582747061,4.71389596270618,-1.64536292767826));
#27343=CARTESIAN_POINT('Ctrl Pts',(36.9759946077044,4.92360289701643,-0.828353078998293));
#27344=CARTESIAN_POINT('Ctrl Pts',(37.0156309407027,4.92540928360095,-0.0108838261772031));
#27345=CARTESIAN_POINT('Ctrl Pts',(37.0552672737011,4.92721567018547,0.80658542664391));
#27346=CARTESIAN_POINT('Ctrl Pts',(37.0949036066994,4.72112150904426,1.62451408360616));
#27347=CARTESIAN_POINT('Ctrl Pts',(37.1345399396977,4.33216742137014,2.34352309608281));
#27348=CARTESIAN_POINT('Ctrl Pts',(37.174176272696,3.94321333369602,3.06253210855944));
#27349=CARTESIAN_POINT('Ctrl Pts',(37.2138126056943,3.37139931948902,3.68262147655047));
#27350=CARTESIAN_POINT('Ctrl Pts',(37.2534489386926,2.68620128259561,4.12844979841592));
#27351=CARTESIAN_POINT('Ctrl Pts',(37.293085271691,2.0010032457022,4.57427812028138));
#27352=CARTESIAN_POINT('Ctrl Pts',(37.3327216046893,1.20242118612239,4.84584539602124));
#27353=CARTESIAN_POINT('Ctrl Pts',(37.3723579376876,0.387483523946268,4.91015596364463));
#27354=CARTESIAN_POINT('Ctrl Pts',(37.4119942706859,-0.427454138229844,
4.97446653126802));
#27355=CARTESIAN_POINT('Ctrl Pts',(37.4516306036843,-1.25874740300227,4.83152039077494));
#27356=CARTESIAN_POINT('Ctrl Pts',(37.4912669366826,-2.0053934101798,4.49868562349977));
#27357=CARTESIAN_POINT('Ctrl Pts',(37.5309032696809,-2.75203941735733,4.1658508562246));
#27358=CARTESIAN_POINT('Ctrl Pts',(37.5705396026792,-3.41403816693998,3.64312746216736));
#27359=CARTESIAN_POINT('Ctrl Pts',(37.6101759356775,-3.9109562307027,2.99402679182231));
#27360=CARTESIAN_POINT('Ctrl Pts',(37.6498122686759,-4.40787429446542,2.34492612147726));
#27361=CARTESIAN_POINT('Ctrl Pts',(37.6894486016742,-4.73971167240821,1.56944817484441));
#27362=CARTESIAN_POINT('Ctrl Pts',(37.7290849346725,-4.86614983229095,0.761814202008249));
#27363=CARTESIAN_POINT('Ctrl Pts',(37.7414427811471,-4.90557081930387,0.510009459010666));
#27364=CARTESIAN_POINT('Ctrl Pts',(37.7538006276218,-4.92502551330707,0.255078917155293));
#27365=CARTESIAN_POINT('Ctrl Pts',(37.7661584740964,-4.92480467811149,0.000114993715880741));
#27366=CARTESIAN_POINT('Origin',(41.25,0.,0.));
#27367=CARTESIAN_POINT('',(39.4838415259036,-4.92532729210881,-7.01284572532379E-5));
#27368=CARTESIAN_POINT('',(39.2661584740964,-4.92535986435928,-6.05616521270463E-5));
#27369=CARTESIAN_POINT('',(41.25,-4.925,-6.03138548580071E-16));
#27370=CARTESIAN_POINT('Ctrl Pts',(39.4838415259036,-4.92532729210881,-7.01284572532379E-5));
#27371=CARTESIAN_POINT('Ctrl Pts',(39.4479280544555,-4.92478402189283,0.740663422453838));
#27372=CARTESIAN_POINT('Ctrl Pts',(39.4120145830074,-4.75533077391977,1.48162891276357));
#27373=CARTESIAN_POINT('Ctrl Pts',(39.3761011115593,-4.43228737044207,2.14815909981045));
#27374=CARTESIAN_POINT('Ctrl Pts',(39.3364647785609,-4.07575664821281,2.88378312561361));
#27375=CARTESIAN_POINT('Ctrl Pts',(39.2968284455626,-3.53214240127592,3.52873975902211));
#27376=CARTESIAN_POINT('Ctrl Pts',(39.2571921125643,-2.86749071492952,4.00465759431309));
#27377=CARTESIAN_POINT('Ctrl Pts',(39.217555779566,-2.20283902858313,4.48057542960406));
#27378=CARTESIAN_POINT('Ctrl Pts',(39.1779194465677,-1.41714990282724,4.7874544667775));
#27379=CARTESIAN_POINT('Ctrl Pts',(39.1382831135693,-0.605887020789073,
4.8880129502341));
#27380=CARTESIAN_POINT('Ctrl Pts',(39.098646780571,0.205375861249093,4.98857143369071));
#27381=CARTESIAN_POINT('Ctrl Pts',(39.0590104475727,1.04221249956953,4.88280936343047));
#27382=CARTESIAN_POINT('Ctrl Pts',(39.0193741145744,1.80294739451225,4.5835747596906));
#27383=CARTESIAN_POINT('Ctrl Pts',(38.9797377815761,2.56368228945497,4.28434015595073));
#27384=CARTESIAN_POINT('Ctrl Pts',(38.9401014485778,3.24831544101998,3.79163301873121));
#27385=CARTESIAN_POINT('Ctrl Pts',(38.9004651155794,3.77366287747338,3.16531878190195));
#27386=CARTESIAN_POINT('Ctrl Pts',(38.8608287825811,4.29901031392678,2.53900454507269));
#27387=CARTESIAN_POINT('Ctrl Pts',(38.8211924495828,4.66507203526857,1.77908320863369));
#27388=CARTESIAN_POINT('Ctrl Pts',(38.7815561165845,4.82737144406183,0.97788533702132));
#27389=CARTESIAN_POINT('Ctrl Pts',(38.7419197835861,4.98967085285509,0.176687465408939));
#27390=CARTESIAN_POINT('Ctrl Pts',(38.7022834505878,4.94820794909981,-0.665786941376808));
#27391=CARTESIAN_POINT('Ctrl Pts',(38.6626471175895,4.70802040038411,-1.44717623190548));
#27392=CARTESIAN_POINT('Ctrl Pts',(38.6230107845912,4.46783285166841,-2.22856552243415));
#27393=CARTESIAN_POINT('Ctrl Pts',(38.5833744515928,4.02892065799228,-2.94886969670574));
#27394=CARTESIAN_POINT('Ctrl Pts',(38.5437381185945,3.44461209146379,-3.52057130300519));
#27395=CARTESIAN_POINT('Ctrl Pts',(38.5041017855962,2.86030352493532,-4.09227290930463));
#27396=CARTESIAN_POINT('Ctrl Pts',(38.4644654525979,2.13059858555448,-4.51537194763194));
#27397=CARTESIAN_POINT('Ctrl Pts',(38.4248291195996,1.34415703490748,-4.73846144550029));
#27398=CARTESIAN_POINT('Ctrl Pts',(38.3851927866013,0.557715484260454,-4.96155094336865));
#27399=CARTESIAN_POINT('Ctrl Pts',(38.3455564536029,-0.285462677652743,
-4.98463090077803));
#27400=CARTESIAN_POINT('Ctrl Pts',(38.3059201206046,-1.0829305511676,-4.80489711703856));
#27401=CARTESIAN_POINT('Ctrl Pts',(38.2662837876063,-1.88039842468243,-4.6251633332991));
#27402=CARTESIAN_POINT('Ctrl Pts',(38.226647454608,-2.63215600979892,-4.2426158084108));
#27403=CARTESIAN_POINT('Ctrl Pts',(38.1870111216097,-3.24686410815625,-3.70373438467301));
#27404=CARTESIAN_POINT('Ctrl Pts',(38.1473747886113,-3.8615722065136,-3.16485296093521));
#27405=CARTESIAN_POINT('Ctrl Pts',(38.107738455613,-4.33923081811179,-2.46963763834791));
#27406=CARTESIAN_POINT('Ctrl Pts',(38.0681021226147,-4.62180399950339,-1.70255769650709));
#27407=CARTESIAN_POINT('Ctrl Pts',(38.0400152570443,-4.82203934821423,-1.15899401191694));
#27408=CARTESIAN_POINT('Ctrl Pts',(38.011928391474,-4.92431567276809,-0.579344659801372));
#27409=CARTESIAN_POINT('Ctrl Pts',(37.9838415259036,-4.92485067281264,0.000120817417613023));
#27410=CARTESIAN_POINT('Ctrl Pts',(37.7661584740964,-4.92480467811149,0.000114993715880741));
#27411=CARTESIAN_POINT('Ctrl Pts',(37.7934369606201,-4.92431721049982,-0.5626877538214));
#27412=CARTESIAN_POINT('Ctrl Pts',(37.8207154471438,-4.82796004188169,-1.12565315428906));
#27413=CARTESIAN_POINT('Ctrl Pts',(37.8479939336675,-4.63886049554297,-1.65552057418984));
#27414=CARTESIAN_POINT('Ctrl Pts',(37.8876302666658,-4.36409405708955,-2.4254313785122));
#27415=CARTESIAN_POINT('Ctrl Pts',(37.9272665996641,-3.89352223836002,-3.12546298811743));
#27416=CARTESIAN_POINT('Ctrl Pts',(37.9669029326624,-3.28431992769162,-3.6705609490957));
#27417=CARTESIAN_POINT('Ctrl Pts',(38.0065392656607,-2.67511761702323,-4.21565891007397));
#27418=CARTESIAN_POINT('Ctrl Pts',(38.0461755986591,-1.92728481441597,-4.6058232224253));
#27419=CARTESIAN_POINT('Ctrl Pts',(38.0858119316574,-1.13168386082912,-4.79364857998611));
#27420=CARTESIAN_POINT('Ctrl Pts',(38.1254482646557,-0.336082907242237,
-4.98147393754693));
#27421=CARTESIAN_POINT('Ctrl Pts',(38.165084597654,0.507286197324216,-4.96696034031723));
#27422=CARTESIAN_POINT('Ctrl Pts',(38.2047209306523,1.29595336769371,-4.75187120364867));
#27423=CARTESIAN_POINT('Ctrl Pts',(38.2443572636507,2.08462053806321,-4.53678206698012));
#27424=CARTESIAN_POINT('Ctrl Pts',(38.283993596649,2.81858577423572,-4.1211173908727));
#27425=CARTESIAN_POINT('Ctrl Pts',(38.3236299296473,3.40867165653206,-3.55538079661358));
#27426=CARTESIAN_POINT('Ctrl Pts',(38.3632662626456,3.99875753882839,-2.98964420235446));
#27427=CARTESIAN_POINT('Ctrl Pts',(38.402902595644,4.44496406724855,-2.27383568994364));
#27428=CARTESIAN_POINT('Ctrl Pts',(38.4425389286423,4.69307675806728,-1.49492662321651));
#27429=CARTESIAN_POINT('Ctrl Pts',(38.4821752616406,4.94118944888601,-0.716017556489387));
#27430=CARTESIAN_POINT('Ctrl Pts',(38.5218115946389,4.9912083021033,0.125992064554042));
#27431=CARTESIAN_POINT('Ctrl Pts',(38.5614479276372,4.83705598218242,0.928797337566571));
#27432=CARTESIAN_POINT('Ctrl Pts',(38.6010842606355,4.68290366226154,1.73160261057911));
#27433=CARTESIAN_POINT('Ctrl Pts',(38.6407205936339,4.32458016920247,2.49520353556076));
#27434=CARTESIAN_POINT('Ctrl Pts',(38.6803569266322,3.80562212350232,3.12682192191077));
#27435=CARTESIAN_POINT('Ctrl Pts',(38.7199932596305,3.28666407780217,3.75844030826078));
#27436=CARTESIAN_POINT('Ctrl Pts',(38.7596295926288,2.60707147946093,4.25807615597916));
#27437=CARTESIAN_POINT('Ctrl Pts',(38.7992659256271,1.8494154206263,4.56502328970031));
#27438=CARTESIAN_POINT('Ctrl Pts',(38.8389022586255,1.09175936179166,4.87197042342147));
#27439=CARTESIAN_POINT('Ctrl Pts',(38.8785385916238,0.256039842463638,4.9862288431454));
#27440=CARTESIAN_POINT('Ctrl Pts',(38.9181749246221,-0.556202475131627,
4.8939160148322));
#27441=CARTESIAN_POINT('Ctrl Pts',(38.9578112576204,-1.36844479272689,4.80160318651899));
#27442=CARTESIAN_POINT('Ctrl Pts',(38.9974475906187,-2.15720990858938,4.50271911016864));
#27443=CARTESIAN_POINT('Ctrl Pts',(39.0370839236171,-2.82666218631365,4.03357853464529));
#27444=CARTESIAN_POINT('Ctrl Pts',(39.0767202566154,-3.49611446403792,3.56443795912194));
#27445=CARTESIAN_POINT('Ctrl Pts',(39.1163565896137,-4.04625390362397,2.92504088442559));
#27446=CARTESIAN_POINT('Ctrl Pts',(39.1559929226121,-4.41023804827196,2.19307447250255));
#27447=CARTESIAN_POINT('Ctrl Pts',(39.1927147731068,-4.74745822812066,1.51492997444862));
#27448=CARTESIAN_POINT('Ctrl Pts',(39.2294366236016,-4.92489283176939,0.757328994148836));
#27449=CARTESIAN_POINT('Ctrl Pts',(39.2661584740964,-4.92535986435928,-6.05616521270463E-5));
#27450=CARTESIAN_POINT('Origin',(41.25,0.,0.));
#27451=CARTESIAN_POINT('',(40.9838415259036,-4.92312335471689,0.00654147285873569));
#27452=CARTESIAN_POINT('',(40.7661584740964,-4.92470501206087,0.000456272822055327));
#27453=CARTESIAN_POINT('',(41.25,-4.925,-6.03138548580071E-16));
#27454=CARTESIAN_POINT('Ctrl Pts',(40.9838415259036,-4.92312335471689,0.00654147285873569));
#27455=CARTESIAN_POINT('Ctrl Pts',(40.9632003834336,-4.92719130640019,0.433011391936502));
#27456=CARTESIAN_POINT('Ctrl Pts',(40.9425592409637,-4.87680194143325,0.858319305362528));
#27457=CARTESIAN_POINT('Ctrl Pts',(40.9219180984937,-4.76835699241177,1.26767821358287));
#27458=CARTESIAN_POINT('Ctrl Pts',(40.8426454324971,-4.35187228303479,2.83982820728391));
#27459=CARTESIAN_POINT('Ctrl Pts',(40.7633727665005,-3.07909246396308,4.17673717491474));
#27460=CARTESIAN_POINT('Ctrl Pts',(40.6841001005039,-1.5283810325561,4.68726372815487));
#27461=CARTESIAN_POINT('Ctrl Pts',(40.6444637675055,-0.753025316852604,
4.94252700477493));
#27462=CARTESIAN_POINT('Ctrl Pts',(40.6048274345072,0.0918133019347075,
4.9911946777973));
#27463=CARTESIAN_POINT('Ctrl Pts',(40.5651911015089,0.89643139271475,4.84097909079969));
#27464=CARTESIAN_POINT('Ctrl Pts',(40.5255547685106,1.70104948349479,4.69076350380207));
#27465=CARTESIAN_POINT('Ctrl Pts',(40.4859184355122,2.46544704626757,4.34166465678447));
#27466=CARTESIAN_POINT('Ctrl Pts',(40.4462821025139,3.10020438041818,3.82803285295568));
#27467=CARTESIAN_POINT('Ctrl Pts',(40.4066457695156,3.73496171456878,3.3144010491269));
#27468=CARTESIAN_POINT('Ctrl Pts',(40.3670094365173,4.24007882009722,2.63623628848694));
#27469=CARTESIAN_POINT('Ctrl Pts',(40.327373103519,4.55242656245004,1.88020324123194));
#27470=CARTESIAN_POINT('Ctrl Pts',(40.2877367705206,4.86477430480286,1.12417019397695));
#27471=CARTESIAN_POINT('Ctrl Pts',(40.2481004375223,4.98435268398005,0.290268860106923));
#27472=CARTESIAN_POINT('Ctrl Pts',(40.208464104524,4.8975150328889,-0.522335340103032));
#27473=CARTESIAN_POINT('Ctrl Pts',(40.1688277715257,4.81067738179775,-1.33493954031299));
#27474=CARTESIAN_POINT('Ctrl Pts',(40.1291914385274,4.51742370043825,-2.12624660686287));
#27475=CARTESIAN_POINT('Ctrl Pts',(40.089555105529,4.05294216033234,-2.7990307722324));
#27476=CARTESIAN_POINT('Ctrl Pts',(40.0499187725307,3.58846062022643,-3.47181493760193));
#27477=CARTESIAN_POINT('Ctrl Pts',(40.0102824395324,2.9527512213741,-4.0260762017911));
#27478=CARTESIAN_POINT('Ctrl Pts',(39.9706461065341,2.22327502076688,-4.39501351572401));
#27479=CARTESIAN_POINT('Ctrl Pts',(39.9310097735357,1.49379882015967,-4.76395082965692));
#27480=CARTESIAN_POINT('Ctrl Pts',(39.8913734405374,0.670555817797568,-4.94756419333357));
#27481=CARTESIAN_POINT('Ctrl Pts',(39.8517371075391,-0.146540443155989,
-4.92327259531741));
#27482=CARTESIAN_POINT('Ctrl Pts',(39.8121007745408,-0.963636704109558,
-4.89898099730126));
#27483=CARTESIAN_POINT('Ctrl Pts',(39.7724644415425,-1.77458622365459,-4.6667844375923));
#27484=CARTESIAN_POINT('Ctrl Pts',(39.7328281085442,-2.48080217325227,-4.25503128141026));
#27485=CARTESIAN_POINT('Ctrl Pts',(39.6931917755458,-3.18701812284995,-3.84327812522822));
#27486=CARTESIAN_POINT('Ctrl Pts',(39.6535554425475,-3.78850050250029,-3.2519683725731));
#27487=CARTESIAN_POINT('Ctrl Pts',(39.6139191095492,-4.21219662658612,-2.55287835332392));
#27488=CARTESIAN_POINT('Ctrl Pts',(39.5742827765509,-4.63589275067194,-1.85378833407475));
#27489=CARTESIAN_POINT('Ctrl Pts',(39.5346464435525,-4.88180261919324,-1.04691804823153));
#27490=CARTESIAN_POINT('Ctrl Pts',(39.4950101105542,-4.92003395469309,-0.230337196211024));
#27491=CARTESIAN_POINT('Ctrl Pts',(39.491287249004,-4.92362485118071,-0.15363944879941));
#27492=CARTESIAN_POINT('Ctrl Pts',(39.4875643874538,-4.92538360857494,-0.0768560348162278));
#27493=CARTESIAN_POINT('Ctrl Pts',(39.4838415259036,-4.92532729210881,-7.01284572532379E-5));
#27494=CARTESIAN_POINT('Ctrl Pts',(39.2661584740964,-4.92535986435928,-6.05616521270463E-5));
#27495=CARTESIAN_POINT('Ctrl Pts',(39.2690729565999,-4.92539693107279,-0.0601718735549025));
#27496=CARTESIAN_POINT('Ctrl Pts',(39.2719874391034,-4.92431927345987,-0.120281853688074));
#27497=CARTESIAN_POINT('Ctrl Pts',(39.274901921607,-4.9221183016965,-0.180350673538913));
#27498=CARTESIAN_POINT('Ctrl Pts',(39.3145382546053,-4.89218556076315,-0.997273658507651));
#27499=CARTESIAN_POINT('Ctrl Pts',(39.3541745876036,-4.65449122918653,-1.80658387929538));
#27500=CARTESIAN_POINT('Ctrl Pts',(39.393810920602,-4.23791524610868,-2.50995000407357));
#27501=CARTESIAN_POINT('Ctrl Pts',(39.4334472536003,-3.82133926303084,-3.21331612885174));
#27502=CARTESIAN_POINT('Ctrl Pts',(39.4730835865986,-3.22588162845177,-3.81073815762037));
#27503=CARTESIAN_POINT('Ctrl Pts',(39.5127199195969,-2.52389122711134,-4.22962765446655));
#27504=CARTESIAN_POINT('Ctrl Pts',(39.5523562525952,-1.8219008257709,-4.64851715131273));
#27505=CARTESIAN_POINT('Ctrl Pts',(39.5919925855935,-1.01337765766909,-4.88887411623647));
#27506=CARTESIAN_POINT('Ctrl Pts',(39.6316289185919,-0.1965574769085,-4.92149723378835));
#27507=CARTESIAN_POINT('Ctrl Pts',(39.6712652515902,0.620262703852086,-4.95412035134023));
#27508=CARTESIAN_POINT('Ctrl Pts',(39.7109015845885,1.44537989727145,-4.77900962152026));
#27509=CARTESIAN_POINT('Ctrl Pts',(39.7505379175869,2.17854060488518,-4.41743662914066));
#27510=CARTESIAN_POINT('Ctrl Pts',(39.7901742505852,2.91170131249894,-4.05586363676105));
#27511=CARTESIAN_POINT('Ctrl Pts',(39.8298105835835,3.55290553430707,-3.50782838182181));
#27512=CARTESIAN_POINT('Ctrl Pts',(39.8694469165818,4.02424846332451,-2.83992665169721));
#27513=CARTESIAN_POINT('Ctrl Pts',(39.9090832495801,4.49559139234193,-2.17202492157262));
#27514=CARTESIAN_POINT('Ctrl Pts',(39.9487195825785,4.79707302856867,-1.38425671626268));
#27515=CARTESIAN_POINT('Ctrl Pts',(39.9883559155768,4.89205896281718,-0.572318557806623));
#27516=CARTESIAN_POINT('Ctrl Pts',(40.0279922485751,4.98704489706568,0.23961960064943));
#27517=CARTESIAN_POINT('Ctrl Pts',(40.0676285815734,4.87553512933595,1.07572771225159));
#27518=CARTESIAN_POINT('Ctrl Pts',(40.1072649145717,4.57108642730011,1.83438198185512));
#27519=CARTESIAN_POINT('Ctrl Pts',(40.14690124757,4.26663772526427,2.59303625145865));
#27520=CARTESIAN_POINT('Ctrl Pts',(40.1865375805684,3.76925008892232,3.27423667906355));
#27521=CARTESIAN_POINT('Ctrl Pts',(40.2261739135667,3.13934012392578,3.79528850237715));
#27522=CARTESIAN_POINT('Ctrl Pts',(40.265810246565,2.50943015892925,4.31634032569076));
#27523=CARTESIAN_POINT('Ctrl Pts',(40.3054465795633,1.74699786527812,4.67724354471308));
#27524=CARTESIAN_POINT('Ctrl Pts',(40.3450829125616,0.944712214563968,4.83400506215193));
#27525=CARTESIAN_POINT('Ctrl Pts',(40.3847192455599,0.142426563849815,4.99076657959077));
#27526=CARTESIAN_POINT('Ctrl Pts',(40.4243555785583,-0.699712443927367,
4.94338639544614));
#27527=CARTESIAN_POINT('Ctrl Pts',(40.4639919115566,-1.47944958844674,4.69790665725705));
#27528=CARTESIAN_POINT('Ctrl Pts',(40.5036282445549,-2.25918673296613,4.45242691906795));
#27529=CARTESIAN_POINT('Ctrl Pts',(40.5432645775532,-2.9765220142277,4.00884762683438));
#27530=CARTESIAN_POINT('Ctrl Pts',(40.5829009105516,-3.54416805574804,3.42049456712443));
#27531=CARTESIAN_POINT('Ctrl Pts',(40.6225372435499,-4.11181409726837,2.8321415074145));
#27532=CARTESIAN_POINT('Ctrl Pts',(40.6621735765482,-4.52977089904747,2.0990146802282));
#27533=CARTESIAN_POINT('Ctrl Pts',(40.7018099095466,-4.74751677154496,1.31132578004485));
#27534=CARTESIAN_POINT('Ctrl Pts',(40.7232594310632,-4.86535170792741,0.885061574079994));
#27535=CARTESIAN_POINT('Ctrl Pts',(40.7447089525798,-4.92455446162076,0.442818752745147));
#27536=CARTESIAN_POINT('Ctrl Pts',(40.7661584740964,-4.92470501206087,0.000456272822055327));
#27537=CARTESIAN_POINT('Origin',(41.25,0.,0.));
#27538=CARTESIAN_POINT('',(42.4838415259036,-4.92524003303928,0.000110626574143721));
#27539=CARTESIAN_POINT('',(42.2661584740964,-4.92524231653586,-0.000581745865239311));
#27540=CARTESIAN_POINT('',(41.25,-4.925,-6.03138548580071E-16));
#27541=CARTESIAN_POINT('Ctrl Pts',(42.4838415259036,-4.92524003303928,0.000110626574143721));
#27542=CARTESIAN_POINT('Ctrl Pts',(42.4784727124118,-4.92534069746969,0.110850170218861));
#27543=CARTESIAN_POINT('Ctrl Pts',(42.4731038989201,-4.92168159671247,0.221582690680517));
#27544=CARTESIAN_POINT('Ctrl Pts',(42.4677350854283,-4.91421672981629,0.332057585799473));
#27545=CARTESIAN_POINT('Ctrl Pts',(42.42809875243,-4.85910586583519,1.14766046297098));
#27546=CARTESIAN_POINT('Ctrl Pts',(42.3884624194316,-4.59656460406497,1.94922166617571));
#27547=CARTESIAN_POINT('Ctrl Pts',(42.3488260864333,-4.158498505033,2.63942433349232));
#27548=CARTESIAN_POINT('Ctrl Pts',(42.309189753435,-3.72043240600104,3.32962700080891));
#27549=CARTESIAN_POINT('Ctrl Pts',(42.2695534204367,-3.10684146970732,3.90847113223737));
#27550=CARTESIAN_POINT('Ctrl Pts',(42.2299170874384,-2.39226443364707,4.30547999981316));
#27551=CARTESIAN_POINT('Ctrl Pts',(42.19028075444,-1.67768739758682,4.70248886738895));
#27552=CARTESIAN_POINT('Ctrl Pts',(42.1506444214417,-0.862124261760032,
4.91766247111206));
#27553=CARTESIAN_POINT('Ctrl Pts',(42.1110080884434,-0.044692789168467,
4.92514955874023));
#27554=CARTESIAN_POINT('Ctrl Pts',(42.0713717554451,0.77273868342311,4.93263664636839));
#27555=CARTESIAN_POINT('Ctrl Pts',(42.0317354224467,1.59203849277947,4.7324372179016));
#27556=CARTESIAN_POINT('Ctrl Pts',(41.9920990894484,2.31371310296222,4.34829220454241));
#27557=CARTESIAN_POINT('Ctrl Pts',(41.9524627564501,3.03538771314496,3.96414719118321));
#27558=CARTESIAN_POINT('Ctrl Pts',(41.9128264234518,3.6594371241541,3.39605659293162));
#27559=CARTESIAN_POINT('Ctrl Pts',(41.8731900904534,4.10993491693973,2.71420756085693));
#27560=CARTESIAN_POINT('Ctrl Pts',(41.8335537574551,4.56043270972535,2.03235852878226));
#27561=CARTESIAN_POINT('Ctrl Pts',(41.7939174244568,4.83737888428748,1.2367510628845));
#27562=CARTESIAN_POINT('Ctrl Pts',(41.7542810914585,4.90733051716129,0.421733363841795));
#27563=CARTESIAN_POINT('Ctrl Pts',(41.7146447584602,4.9772821500351,-0.393284335200907));
#27564=CARTESIAN_POINT('Ctrl Pts',(41.6750084254618,4.8402392412206,-1.22771226738855));
#27565=CARTESIAN_POINT('Ctrl Pts',(41.6353720924635,4.51245254963717,-1.97556946497589));
#27566=CARTESIAN_POINT('Ctrl Pts',(41.5957357594652,4.18466585805374,-2.72342666256322));
#27567=CARTESIAN_POINT('Ctrl Pts',(41.5560994264669,3.66613538370139,-3.38471312555024));
#27568=CARTESIAN_POINT('Ctrl Pts',(41.5164630934686,3.02049996896988,-3.88783329591911));
#27569=CARTESIAN_POINT('Ctrl Pts',(41.4768267604703,2.37486455423836,-4.39095346628799));
#27570=CARTESIAN_POINT('Ctrl Pts',(41.4371904274719,1.60212419912768,-4.73590734403872));
#27571=CARTESIAN_POINT('Ctrl Pts',(41.3975540944736,0.796173003049936,-4.86543917721391));
#27572=CARTESIAN_POINT('Ctrl Pts',(41.318281428477,-0.815729389105595,-5.12450284356429));
#27573=CARTESIAN_POINT('Ctrl Pts',(41.2390087624804,-2.56047514512941,-4.52187833161248));
#27574=CARTESIAN_POINT('Ctrl Pts',(41.1597360964837,-3.6527532233002,-3.31687056575093));
#27575=CARTESIAN_POINT('Ctrl Pts',(41.101104572957,-4.46062220351945,-2.42562463267031));
#27576=CARTESIAN_POINT('Ctrl Pts',(41.0424730494303,-4.91156826733875,-1.20485373601841));
#27577=CARTESIAN_POINT('Ctrl Pts',(40.9838415259036,-4.92312335471689,0.00654147285873569));
#27578=CARTESIAN_POINT('Ctrl Pts',(40.7661584740964,-4.92470501206087,0.000456272822055327));
#27579=CARTESIAN_POINT('Ctrl Pts',(40.7843452855781,-4.92483266210987,-0.374617969403003));
#27580=CARTESIAN_POINT('Ctrl Pts',(40.8025320970598,-4.88250676151333,-0.749778236054864));
#27581=CARTESIAN_POINT('Ctrl Pts',(40.8207189085415,-4.79747128229509,-1.11535753233566));
#27582=CARTESIAN_POINT('Ctrl Pts',(40.8603552415398,-4.61214497733185,-1.91210097135244));
#27583=CARTESIAN_POINT('Ctrl Pts',(40.8999915745381,-4.22395742418951,-2.66333687620561));
#27584=CARTESIAN_POINT('Ctrl Pts',(40.9396279075364,-3.68111313624165,-3.2733004318091));
#27585=CARTESIAN_POINT('Ctrl Pts',(40.9792642405348,-3.13826884829379,-3.88326398741259));
#27586=CARTESIAN_POINT('Ctrl Pts',(41.0189005735331,-2.44076782554041,-4.35195519376641));
#27587=CARTESIAN_POINT('Ctrl Pts',(41.0585369065314,-1.67125931107344,-4.63093894008567));
#27588=CARTESIAN_POINT('Ctrl Pts',(41.0981732395297,-0.901750796606443,
-4.90992268640494));
#27589=CARTESIAN_POINT('Ctrl Pts',(41.1378095725281,-0.0602347904258443,
-4.99919897268965));
#27590=CARTESIAN_POINT('Ctrl Pts',(41.1774459055264,0.746297725178827,-4.87333646147363));
#27591=CARTESIAN_POINT('Ctrl Pts',(41.256718571523,2.35936275638813,-4.62161143904159));
#27592=CARTESIAN_POINT('Ctrl Pts',(41.3359912375197,3.83249382529375,-3.50933122660671));
#27593=CARTESIAN_POINT('Ctrl Pts',(41.4152639035163,4.49894422300268,-2.02576932080728));
#27594=CARTESIAN_POINT('Ctrl Pts',(41.4945365695129,5.16539462071163,-0.542207415007845));
#27595=CARTESIAN_POINT('Ctrl Pts',(41.5738092355096,5.0251643472239,1.31263618415612));
#27596=CARTESIAN_POINT('Ctrl Pts',(41.6530819015062,4.14324285485124,2.6791377546773));
#27597=CARTESIAN_POINT('Ctrl Pts',(41.7323545675028,3.26132136247858,4.0456393251985));
#27598=CARTESIAN_POINT('Ctrl Pts',(41.8116272334995,1.63770865122098,4.92379886707688));
#27599=CARTESIAN_POINT('Ctrl Pts',(41.8908998994961,0.00513277477895049,
4.9301462671972));
#27600=CARTESIAN_POINT('Ctrl Pts',(41.9305362324945,-0.811155163442051,
4.93331996725735));
#27601=CARTESIAN_POINT('Ctrl Pts',(41.9701725654928,-1.62968389295916,4.718540631878));
#27602=CARTESIAN_POINT('Ctrl Pts',(42.0098088984911,-2.34850201279282,4.32703610425884));
#27603=CARTESIAN_POINT('Ctrl Pts',(42.0494452314894,-3.06732013262647,3.93553157663968));
#27604=CARTESIAN_POINT('Ctrl Pts',(42.0890815644878,-3.68642764277668,3.36730185678069));
#27605=CARTESIAN_POINT('Ctrl Pts',(42.1287178974861,-4.13139670740965,2.68265742962034));
#27606=CARTESIAN_POINT('Ctrl Pts',(42.1683542304844,-4.57636577204261,1.99801300245999));
#27607=CARTESIAN_POINT('Ctrl Pts',(42.2079905634827,-4.84719639115833,1.19695386799826));
#27608=CARTESIAN_POINT('Ctrl Pts',(42.247626896481,-4.91062973406511,0.381403650086907));
#27609=CARTESIAN_POINT('Ctrl Pts',(42.2538040890195,-4.92051561257233,0.254302822645805));
#27610=CARTESIAN_POINT('Ctrl Pts',(42.2599812815579,-4.92536418444955,0.126850032864256));
#27611=CARTESIAN_POINT('Ctrl Pts',(42.2661584740964,-4.92524231653586,-0.000581745865239312));
#27612=CARTESIAN_POINT('Origin',(41.25,0.,0.));
#27613=CARTESIAN_POINT('',(43.9838415259036,-4.92495182736585,-0.000126817358605258));
#27614=CARTESIAN_POINT('',(43.7661584740964,-4.92500388850328,-0.000126728605493087));
#27615=CARTESIAN_POINT('',(41.25,-4.925,-6.03138548580071E-16));
#27616=CARTESIAN_POINT('Ctrl Pts',(43.9838415259036,-4.92495182736585,-0.000126817358605258));
#27617=CARTESIAN_POINT('Ctrl Pts',(43.9541087083917,-4.92433624971945,0.613260411095392));
#27618=CARTESIAN_POINT('Ctrl Pts',(43.9243758908798,-4.80942794181503,1.22687181317958));
#27619=CARTESIAN_POINT('Ctrl Pts',(43.8946430733678,-4.58560281726217,1.79778244828448));
#27620=CARTESIAN_POINT('Ctrl Pts',(43.8550067403695,-4.2872252024731,2.558854083565));
#27621=CARTESIAN_POINT('Ctrl Pts',(43.8153704073711,-3.79529020284407,3.24404167227217));
#27622=CARTESIAN_POINT('Ctrl Pts',(43.7757340743728,-3.16956835360222,3.77009434044043));
#27623=CARTESIAN_POINT('Ctrl Pts',(43.7360977413745,-2.54384650436036,4.29614700860869));
#27624=CARTESIAN_POINT('Ctrl Pts',(43.6964614083762,-1.78433780550569,4.66306475623804));
#27625=CARTESIAN_POINT('Ctrl Pts',(43.6568250753779,-0.983323226255741,
4.82626671845745));
#27626=CARTESIAN_POINT('Ctrl Pts',(43.6171887423796,-0.182308647005795,
4.98946868067685));
#27627=CARTESIAN_POINT('Ctrl Pts',(43.5775524093812,0.660211812639427,4.94895485748631));
#27628=CARTESIAN_POINT('Ctrl Pts',(43.5379160763829,1.44187117188668,4.70964778766782));
#27629=CARTESIAN_POINT('Ctrl Pts',(43.4982797433846,2.22353053113393,4.47034071784932));
#27630=CARTESIAN_POINT('Ctrl Pts',(43.4586434103863,2.94432878998322,4.03224040140287));
#27631=CARTESIAN_POINT('Ctrl Pts',(43.4190070773879,3.5166883414399,3.44857626359137));
#27632=CARTESIAN_POINT('Ctrl Pts',(43.3793707443896,4.08904789289657,2.86491212577987));
#27633=CARTESIAN_POINT('Ctrl Pts',(43.3397344113913,4.51296873696065,2.13568416660331));
#27634=CARTESIAN_POINT('Ctrl Pts',(43.300098078393,4.73694409335704,1.34949451562975));
#27635=CARTESIAN_POINT('Ctrl Pts',(43.2604617453947,4.96091944975344,0.563304864656144));
#27636=CARTESIAN_POINT('Ctrl Pts',(43.2208254123963,4.98494931848214,-0.279846478114447));
#27637=CARTESIAN_POINT('Ctrl Pts',(43.181189079398,4.8061141017137,-1.07751647096024));
#27638=CARTESIAN_POINT('Ctrl Pts',(43.1415527463997,4.62727888494526,-1.87518646380601));
#27639=CARTESIAN_POINT('Ctrl Pts',(43.1019164134014,4.24557858267969,-2.62737510672696));
#27640=CARTESIAN_POINT('Ctrl Pts',(43.0622800804031,3.7073900118728,-3.2426896528834));
#27641=CARTESIAN_POINT('Ctrl Pts',(43.0226437474048,3.16920144106591,-3.85800419903984));
#27642=CARTESIAN_POINT('Ctrl Pts',(42.9830074144064,2.4745246017177,-4.33644464843178));
#27643=CARTESIAN_POINT('Ctrl Pts',(42.9433710814081,1.70776354660135,-4.61988239596167));
#27644=CARTESIAN_POINT('Ctrl Pts',(42.9037347484098,0.941002491484994,-4.90332014349156));
#27645=CARTESIAN_POINT('Ctrl Pts',(42.8640984154114,0.102157220600491,-4.9917551891594));
#27646=CARTESIAN_POINT('Ctrl Pts',(42.8244620824131,-0.706852245384476,
-4.87443795232758));
#27647=CARTESIAN_POINT('Ctrl Pts',(42.7848257494148,-1.51586171136944,-4.75712071549575));
#27648=CARTESIAN_POINT('Ctrl Pts',(42.7451894164165,-2.29503537245488,-4.43405119616424));
#27649=CARTESIAN_POINT('Ctrl Pts',(42.7055530834182,-2.94970211843778,-3.94449188930112));
#27650=CARTESIAN_POINT('Ctrl Pts',(42.6659167504199,-3.60436886442068,-3.454932582438));
#27651=CARTESIAN_POINT('Ctrl Pts',(42.6262804174215,-4.13452869530104,-2.79888348804327));
#27652=CARTESIAN_POINT('Ctrl Pts',(42.5866440844232,-4.47576837764522,-2.05603666527677));
#27653=CARTESIAN_POINT('Ctrl Pts',(42.5523765649167,-4.77078652353756,-1.41380979755406));
#27654=CARTESIAN_POINT('Ctrl Pts',(42.5181090454101,-4.92459752229869,-0.706706527309889));
#27655=CARTESIAN_POINT('Ctrl Pts',(42.4838415259036,-4.92524003303928,0.000110626574143721));
#27656=CARTESIAN_POINT('Ctrl Pts',(42.2661584740964,-4.92524231653586,-0.000581745865239312));
#27657=CARTESIAN_POINT('Ctrl Pts',(42.2996176145563,-4.92458221154214,-0.690823754191429));
#27658=CARTESIAN_POINT('Ctrl Pts',(42.3330767550162,-4.77809370979876,-1.38044931645573));
#27659=CARTESIAN_POINT('Ctrl Pts',(42.366535895476,-4.49640310266108,-2.01018654256035));
#27660=CARTESIAN_POINT('Ctrl Pts',(42.4061722284743,-4.16270706165249,-2.75618521593511));
#27661=CARTESIAN_POINT('Ctrl Pts',(42.4458085614727,-3.63927891293753,-3.41814126132365));
#27662=CARTESIAN_POINT('Ctrl Pts',(42.485444894471,-2.9896289807233,-3.91446405638524));
#27663=CARTESIAN_POINT('Ctrl Pts',(42.5250812274693,-2.33997904850905,-4.41078685144686));
#27664=CARTESIAN_POINT('Ctrl Pts',(42.5647175604676,-1.56410733279554,-4.7414763961815));
#27665=CARTESIAN_POINT('Ctrl Pts',(42.6043538934659,-0.756326335255354,
-4.86693625596787));
#27666=CARTESIAN_POINT('Ctrl Pts',(42.6439902264642,0.0514546622848183,
-4.99239611575423));
#27667=CARTESIAN_POINT('Ctrl Pts',(42.6836265594626,0.891144941651684,-4.91262629059232));
#27668=CARTESIAN_POINT('Ctrl Pts',(42.7232628924609,1.66074315118674,-4.63702688099208));
#27669=CARTESIAN_POINT('Ctrl Pts',(42.7628992254592,2.43034136072179,-4.36142747139185));
#27670=CARTESIAN_POINT('Ctrl Pts',(42.8025355584575,3.12984750042507,-3.88999847735328));
#27671=CARTESIAN_POINT('Ctrl Pts',(42.8421718914558,3.67426005949087,-3.28016527711588));
#27672=CARTESIAN_POINT('Ctrl Pts',(42.8818082244541,4.21867261855668,-2.67033207687847));
#27673=CARTESIAN_POINT('Ctrl Pts',(42.9214445574525,4.60799159698502,-1.92209467044223));
#27674=CARTESIAN_POINT('Ctrl Pts',(42.9610808904508,4.79491986130557,-1.12629121671947));
#27675=CARTESIAN_POINT('Ctrl Pts',(43.0007172234491,4.98184812562611,-0.330487762996699));
#27676=CARTESIAN_POINT('Ctrl Pts',(43.0403535564475,4.96638567583886,0.512881738012616));
#27677=CARTESIAN_POINT('Ctrl Pts',(43.0799898894458,4.7504084749811,1.30131039653013));
#27678=CARTESIAN_POINT('Ctrl Pts',(43.1196262224441,4.53443127412335,2.08973905504764));
#27679=CARTESIAN_POINT('Ctrl Pts',(43.1592625554424,4.11793932219513,2.82322687107334));
#27680=CARTESIAN_POINT('Ctrl Pts',(43.1988988884407,3.55153812862758,3.41267285313056));
#27681=CARTESIAN_POINT('Ctrl Pts',(43.2385352214391,2.98513693506004,4.00211883518778));
#27682=CARTESIAN_POINT('Ctrl Pts',(43.2781715544374,2.26882649985319,4.44752298327648));
#27683=CARTESIAN_POINT('Ctrl Pts',(43.3178078874357,1.48963848090206,4.69475907111567));
#27684=CARTESIAN_POINT('Ctrl Pts',(43.357444220434,0.710450461950941,4.94199515895486));
#27685=CARTESIAN_POINT('Ctrl Pts',(43.3970805534323,-0.131615140744488,
4.99106318654455));
#27686=CARTESIAN_POINT('Ctrl Pts',(43.4367168864306,-0.934246273828332,
4.83600597226192));
#27687=CARTESIAN_POINT('Ctrl Pts',(43.476353219429,-1.73687740691221,4.68094875797928));
#27688=CARTESIAN_POINT('Ctrl Pts',(43.5159895524273,-2.50007407038453,4.32176630182432));
#27689=CARTESIAN_POINT('Ctrl Pts',(43.5556258854256,-3.13110737352768,3.80209726824003));
#27690=CARTESIAN_POINT('Ctrl Pts',(43.5952622184239,-3.76214067667083,3.28242823465576));
#27691=CARTESIAN_POINT('Ctrl Pts',(43.6348985514223,-4.26101061948481,2.60227262364216));
#27692=CARTESIAN_POINT('Ctrl Pts',(43.6745348844206,-4.56710398015465,1.84427110008394));
#27693=CARTESIAN_POINT('Ctrl Pts',(43.7050760809792,-4.80295974143054,1.26020411478287));
#27694=CARTESIAN_POINT('Ctrl Pts',(43.7356172775378,-4.92435927308213,0.62991808387772));
#27695=CARTESIAN_POINT('Ctrl Pts',(43.7661584740964,-4.92500388850328,-0.000126728605493087));
#27696=CARTESIAN_POINT('Origin',(41.25,0.,0.));
#27697=CARTESIAN_POINT('',(45.4838415259036,-4.92470113209118,9.20081859334676E-5));
#27698=CARTESIAN_POINT('',(45.2661584740964,-4.92466880697525,8.05726078428837E-5));
#27699=CARTESIAN_POINT('',(41.25,-4.925,-6.03138548580071E-16));
#27700=CARTESIAN_POINT('Ctrl Pts',(45.4838415259036,-4.92470113209118,9.20081859334676E-5));
#27701=CARTESIAN_POINT('Ctrl Pts',(45.4693810373698,-4.92490179872926,0.298455085306509));
#27702=CARTESIAN_POINT('Ctrl Pts',(45.4549205488361,-4.89822119016455,0.59678269783049));
#27703=CARTESIAN_POINT('Ctrl Pts',(45.4404600603023,-4.84432450427108,0.890109553198539));
#27704=CARTESIAN_POINT('Ctrl Pts',(45.400823727304,-4.69659318906749,1.69412118043862));
#27705=CARTESIAN_POINT('Ctrl Pts',(45.3611873943056,-4.34438389857107,2.46056146020548));
#27706=CARTESIAN_POINT('Ctrl Pts',(45.3215510613073,-3.83049037024208,3.09630722682097));
#27707=CARTESIAN_POINT('Ctrl Pts',(45.281914728309,-3.3165968419131,3.73205299343644));
#27708=CARTESIAN_POINT('Ctrl Pts',(45.2422783953107,-2.64101907575149,4.23710424690058));
#27709=CARTESIAN_POINT('Ctrl Pts',(45.2026420623124,-1.88584036240152,4.55009681731105));
#27710=CARTESIAN_POINT('Ctrl Pts',(45.1630057293141,-1.1306616490515,4.86308938772155));
#27711=CARTESIAN_POINT('Ctrl Pts',(45.1233693963157,-0.29588198851312,4.9840232750784));
#27712=CARTESIAN_POINT('Ctrl Pts',(45.0837330633174,0.517072158884537,4.8982049060758));
#27713=CARTESIAN_POINT('Ctrl Pts',(45.0440967303191,1.33002630628219,4.8123865370732));
#27714=CARTESIAN_POINT('Ctrl Pts',(45.0044603973208,2.12115494053905,4.51981591171113));
#27715=CARTESIAN_POINT('Ctrl Pts',(44.9648240643225,2.79433523927099,4.05604061738936));
#27716=CARTESIAN_POINT('Ctrl Pts',(44.9251877313242,3.46751553800291,3.59226532306761));
#27717=CARTESIAN_POINT('Ctrl Pts',(44.8855513983258,4.02274750120992,2.95728535978618));
#27718=CARTESIAN_POINT('Ctrl Pts',(44.8459150653275,4.39256995877785,2.22825134952313));
#27719=CARTESIAN_POINT('Ctrl Pts',(44.8062787323291,4.76239241634577,1.49921733926011));
#27720=CARTESIAN_POINT('Ctrl Pts',(44.7666423993308,4.94680536827464,0.67612928201546));
#27721=CARTESIAN_POINT('Ctrl Pts',(44.7270060663325,4.92340247928476,-0.141006901853086));
#27722=CARTESIAN_POINT('Ctrl Pts',(44.6873697333342,4.89999959029487,-0.958143085721712));
#27723=CARTESIAN_POINT('Ctrl Pts',(44.6477334003359,4.66878086038622,-1.76932739621425));
#27724=CARTESIAN_POINT('Ctrl Pts',(44.6080970673376,4.25783956788869,-2.47600022885704));
#27725=CARTESIAN_POINT('Ctrl Pts',(44.5684607343393,3.84689827539119,-3.18267306149978));
#27726=CARTESIAN_POINT('Ctrl Pts',(44.5288244013409,3.25623442030485,-3.78483441629277));
#27727=CARTESIAN_POINT('Ctrl Pts',(44.4891880683426,2.55761417863557,-4.20932116061901));
#27728=CARTESIAN_POINT('Ctrl Pts',(44.4495517353443,1.85899393696629,-4.63380790494526));
#27729=CARTESIAN_POINT('Ctrl Pts',(44.409915402346,1.05241730871404,-4.88062003880476));
#27730=CARTESIAN_POINT('Ctrl Pts',(44.3702790693477,0.235884061122376,-4.91976967222236));
#27731=CARTESIAN_POINT('Ctrl Pts',(44.3306427363493,-0.580649186469257,
-4.95891930563996));
#27732=CARTESIAN_POINT('Ctrl Pts',(44.291006403351,-1.40713905340033,-4.79040643861569));
#27733=CARTESIAN_POINT('Ctrl Pts',(44.2513700703527,-2.14316629663364,-4.43470553100115));
#27734=CARTESIAN_POINT('Ctrl Pts',(44.2117337373544,-2.87919353986696,-4.0790046233866));
#27735=CARTESIAN_POINT('Ctrl Pts',(44.172097404356,-3.52475815940249,-3.53611567518177));
#27736=CARTESIAN_POINT('Ctrl Pts',(44.1324610713577,-4.00142348800549,-2.8720001717005));
#27737=CARTESIAN_POINT('Ctrl Pts',(44.0928247383594,-4.47808881660849,-2.20788466821924));
#27738=CARTESIAN_POINT('Ctrl Pts',(44.0531884053611,-4.78585485427895,-1.42254260946154));
#27739=CARTESIAN_POINT('Ctrl Pts',(44.0135520723628,-4.88732775813964,-0.61139373915575));
#27740=CARTESIAN_POINT('Ctrl Pts',(44.0036485568764,-4.91268173008443,-0.408720464633004));
#27741=CARTESIAN_POINT('Ctrl Pts',(43.99374504139,-4.92515686621733,-0.204436076436149));
#27742=CARTESIAN_POINT('Ctrl Pts',(43.9838415259036,-4.92495182736585,-0.000126817358605258));
#27743=CARTESIAN_POINT('Ctrl Pts',(43.7661584740964,-4.92500388850328,-0.000126728605493087));
#27744=CARTESIAN_POINT('Ctrl Pts',(43.7752536105361,-4.9251958543025,-0.18775341578092));
#27745=CARTESIAN_POINT('Ctrl Pts',(43.7843487469758,-4.91467876478723,-0.375358710689233));
#27746=CARTESIAN_POINT('Ctrl Pts',(43.7934438834155,-4.89328627121904,-0.561715594621382));
#27747=CARTESIAN_POINT('Ctrl Pts',(43.8330802164138,-4.8000584230879,-1.37385332966565));
#27748=CARTESIAN_POINT('Ctrl Pts',(43.8727165494122,-4.50028594829992,-2.16228136365135));
#27749=CARTESIAN_POINT('Ctrl Pts',(43.9123528824105,-4.03039144350975,-2.8312047076203));
#27750=CARTESIAN_POINT('Ctrl Pts',(43.9519892154088,-3.56049693871958,-3.50012805158925));
#27751=CARTESIAN_POINT('Ctrl Pts',(43.9916255484071,-2.92048040392721,-4.04954670554145));
#27752=CARTESIAN_POINT('Ctrl Pts',(44.0312618814054,-2.18810441989724,-4.41270596780624));
#27753=CARTESIAN_POINT('Ctrl Pts',(44.0708982144038,-1.45572843586724,-4.77586523007105));
#27754=CARTESIAN_POINT('Ctrl Pts',(44.1105345474021,-0.630993002599663,
-4.95276510064842));
#27755=CARTESIAN_POINT('Ctrl Pts',(44.1501708804004,0.185895807452519,-4.92191201692444));
#27756=CARTESIAN_POINT('Ctrl Pts',(44.1898072133987,1.00278461750467,-4.89105893320045));
#27757=CARTESIAN_POINT('Ctrl Pts',(44.2294435463971,1.8118268043414,-4.65245289517512));
#27758=CARTESIAN_POINT('Ctrl Pts',(44.2690798793954,2.51472303050596,-4.23508478231541));
#27759=CARTESIAN_POINT('Ctrl Pts',(44.3087162123937,3.21761925667052,-3.8177166694557));
#27760=CARTESIAN_POINT('Ctrl Pts',(44.348352545392,3.81436952216293,-3.2215864817616));
#27761=CARTESIAN_POINT('Ctrl Pts',(44.3879888783903,4.23246814812435,-2.51912454105487));
#27762=CARTESIAN_POINT('Ctrl Pts',(44.4276252113887,4.65056677408577,-1.81666260034813));
#27763=CARTESIAN_POINT('Ctrl Pts',(44.467261544387,4.89001376051621,-1.00786890662875));
#27764=CARTESIAN_POINT('Ctrl Pts',(44.5068978773853,4.92171608803313,-0.19101261171286));
#27765=CARTESIAN_POINT('Ctrl Pts',(44.5465342103836,4.95341841555005,0.625843683203033));
#27766=CARTESIAN_POINT('Ctrl Pts',(44.5861705433819,4.77737608415345,1.45076257931545));
#27767=CARTESIAN_POINT('Ctrl Pts',(44.6258068763803,4.4149783917305,2.18351571243843));
#27768=CARTESIAN_POINT('Ctrl Pts',(44.6654432093786,4.05258069930754,2.91626884556144));
#27769=CARTESIAN_POINT('Ctrl Pts',(44.7050795423769,3.50382764585821,3.55685621569501));
#27770=CARTESIAN_POINT('Ctrl Pts',(44.7447158753752,2.83539320811387,4.02744589365957));
#27771=CARTESIAN_POINT('Ctrl Pts',(44.7843522083735,2.16695877036953,4.49803557162413));
#27772=CARTESIAN_POINT('Ctrl Pts',(44.8239885413719,1.37884294833018,4.79862755741967));
#27773=CARTESIAN_POINT('Ctrl Pts',(44.8636248743702,0.566802505140043,4.89269966250424));
#27774=CARTESIAN_POINT('Ctrl Pts',(44.9032612073685,-0.245237938050057,
4.98677176758881));
#27775=CARTESIAN_POINT('Ctrl Pts',(44.9428975403668,-1.08120300239091,4.87432399196243));
#27776=CARTESIAN_POINT('Ctrl Pts',(44.9825338733651,-1.83952219999503,4.56901883832726));
#27777=CARTESIAN_POINT('Ctrl Pts',(45.0221702063635,-2.59784139759917,4.26371368469208));
#27778=CARTESIAN_POINT('Ctrl Pts',(45.0618065393618,-3.27851472846656,3.76555115304811));
#27779=CARTESIAN_POINT('Ctrl Pts',(45.1014428723601,-3.79883978635438,3.1350584278558));
#27780=CARTESIAN_POINT('Ctrl Pts',(45.1410792053584,-4.31916484424219,2.50456570266349));
#27781=CARTESIAN_POINT('Ctrl Pts',(45.1807155383568,-4.67914162915044,1.74174278392284));
#27782=CARTESIAN_POINT('Ctrl Pts',(45.2203518713551,-4.83503264625132,0.93927332462865));
#27783=CARTESIAN_POINT('Ctrl Pts',(45.2356207389355,-4.89508561071691,0.63014281268565));
#27784=CARTESIAN_POINT('Ctrl Pts',(45.250889606516,-4.92485274797344,0.315128851399062));
#27785=CARTESIAN_POINT('Ctrl Pts',(45.2661584740964,-4.92466880697525,8.05726078428837E-5));
#27786=CARTESIAN_POINT('Origin',(41.25,0.,0.));
#27787=CARTESIAN_POINT('',(46.9838415259036,-4.92541598660193,-1.76250313788096E-5));
#27788=CARTESIAN_POINT('',(46.7661584740964,-4.92542130869464,-7.54510152246871E-8));
#27789=CARTESIAN_POINT('',(41.25,-4.925,-6.03138548580071E-16));
#27790=CARTESIAN_POINT('Ctrl Pts',(46.9838415259036,-4.92541598660193,-1.76250313788096E-5));
#27791=CARTESIAN_POINT('Ctrl Pts',(46.9450170333497,-4.92525305960927,0.8007125042042));
#27792=CARTESIAN_POINT('Ctrl Pts',(46.9061925407958,-4.72610526188126,1.60152074077725));
#27793=CARTESIAN_POINT('Ctrl Pts',(46.8673680482419,-4.35075866585062,2.30882523177979));
#27794=CARTESIAN_POINT('Ctrl Pts',(46.8277317152435,-3.96756337619178,3.03091982960743));
#27795=CARTESIAN_POINT('Ctrl Pts',(46.7880953822452,-3.40072342726273,3.65555937291029));
#27796=CARTESIAN_POINT('Ctrl Pts',(46.7484590492469,-2.71911036961906,4.10684960976261));
#27797=CARTESIAN_POINT('Ctrl Pts',(46.7088227162486,-2.03749731197539,4.55813984661494));
#27798=CARTESIAN_POINT('Ctrl Pts',(46.6691863832502,-1.24111114561709,4.83608077701674));
#27799=CARTESIAN_POINT('Ctrl Pts',(46.6295500502519,-0.426713487684489,
4.90690233434551));
#27800=CARTESIAN_POINT('Ctrl Pts',(46.5899137172536,0.387684170248116,4.97772389167427));
#27801=CARTESIAN_POINT('Ctrl Pts',(46.5502773842553,1.22009331975503,4.84142607593));
#27802=CARTESIAN_POINT('Ctrl Pts',(46.510641051257,1.96937551967397,4.51456919117275));
#27803=CARTESIAN_POINT('Ctrl Pts',(46.4710047182587,2.71865771959291,4.18771230641549));
#27804=CARTESIAN_POINT('Ctrl Pts',(46.4313683852603,3.38481296992387,3.67029635264524));
#27805=CARTESIAN_POINT('Ctrl Pts',(46.391732052262,3.88690282395414,3.02518782169216));
#27806=CARTESIAN_POINT('Ctrl Pts',(46.3520957192637,4.38899267798441,2.38007929073908));
#27807=CARTESIAN_POINT('Ctrl Pts',(46.3124593862653,4.72701713571399,1.60727818260316));
#27808=CARTESIAN_POINT('Ctrl Pts',(46.272823053267,4.85990592929473,0.800680509181498));
#27809=CARTESIAN_POINT('Ctrl Pts',(46.2331867202687,4.99279472287548,-0.00591716424018909));
#27810=CARTESIAN_POINT('Ctrl Pts',(46.1935503872704,4.92054785230737,-0.846311402947627));
#27811=CARTESIAN_POINT('Ctrl Pts',(46.1539140542721,4.65194337567933,-1.61839357044276));
#27812=CARTESIAN_POINT('Ctrl Pts',(46.1142777212738,4.38333889905129,-2.39047573793788));
#27813=CARTESIAN_POINT('Ctrl Pts',(46.0746413882754,3.91837681636332,-3.0942458342207));
#27814=CARTESIAN_POINT('Ctrl Pts',(46.0350050552771,3.31355042814016,-3.64419517583092));
#27815=CARTESIAN_POINT('Ctrl Pts',(45.9953687222788,2.708724039917,-4.19414451744114));
#27816=CARTESIAN_POINT('Ctrl Pts',(45.9557323892805,1.96403334615864,-4.59027310437877));
#27817=CARTESIAN_POINT('Ctrl Pts',(45.9160960562822,1.16995891878022,-4.78445096617617));
#27818=CARTESIAN_POINT('Ctrl Pts',(45.8764597232838,0.375884491401773,-4.97862882797357));
#27819=CARTESIAN_POINT('Ctrl Pts',(45.8368233902855,-0.467573669596737,
-4.97085596463074));
#27820=CARTESIAN_POINT('Ctrl Pts',(45.7971870572872,-1.25793465847378,-4.76207678585587));
#27821=CARTESIAN_POINT('Ctrl Pts',(45.7575507242889,-2.0482956473508,-4.55329760708101));
#27822=CARTESIAN_POINT('Ctrl Pts',(45.7179143912906,-2.78555946410635,-4.14351211287411));
#27823=CARTESIAN_POINT('Ctrl Pts',(45.6782780582922,-3.38014790888984,-3.58250959990415));
#27824=CARTESIAN_POINT('Ctrl Pts',(45.6386417252939,-3.97473635367333,-3.02150708693418));
#27825=CARTESIAN_POINT('Ctrl Pts',(45.5990053922956,-4.42664942648476,-2.30928755520114));
#27826=CARTESIAN_POINT('Ctrl Pts',(45.5593690592973,-4.6809792929351,-1.53238630197798));
#27827=CARTESIAN_POINT('Ctrl Pts',(45.5341932148327,-4.84252221772373,-1.03892125019597));
#27828=CARTESIAN_POINT('Ctrl Pts',(45.5090173703681,-4.92435176961579,-0.519360872400719));
#27829=CARTESIAN_POINT('Ctrl Pts',(45.4838415259036,-4.92470113209118,9.20081859334676E-5));
#27830=CARTESIAN_POINT('Ctrl Pts',(45.2661584740964,-4.92466880697525,8.05726078428837E-5));
#27831=CARTESIAN_POINT('Ctrl Pts',(45.2905259395143,-4.9243752569861,-0.50270249221085));
#27832=CARTESIAN_POINT('Ctrl Pts',(45.3148934049322,-4.84780015486276,-1.00557295930924));
#27833=CARTESIAN_POINT('Ctrl Pts',(45.33926087035,-4.69630409857361,-1.48475684285591));
#27834=CARTESIAN_POINT('Ctrl Pts',(45.3788972033484,-4.44987928450151,-2.26420155119845));
#27835=CARTESIAN_POINT('Ctrl Pts',(45.4185335363467,-4.00522440706378,-2.98097496803579));
#27836=CARTESIAN_POINT('Ctrl Pts',(45.458169869345,-3.41636542355341,-3.54798849510125));
#27837=CARTESIAN_POINT('Ctrl Pts',(45.4978062023433,-2.82750644004303,-4.11500202216671));
#27838=CARTESIAN_POINT('Ctrl Pts',(45.5374425353416,-2.09444335046,-4.53225565946027));
#27839=CARTESIAN_POINT('Ctrl Pts',(45.5770788683399,-1.30624396262072,-4.74905272436441));
#27840=CARTESIAN_POINT('Ctrl Pts',(45.6167152013383,-0.518044574781435,
-4.96584978926855));
#27841=CARTESIAN_POINT('Ctrl Pts',(45.6563515343366,0.325291111314094,-4.98219028178326));
#27842=CARTESIAN_POINT('Ctrl Pts',(45.6959878673349,1.12129707073172,-4.79608881775695));
#27843=CARTESIAN_POINT('Ctrl Pts',(45.7356242003332,1.91730303014935,-4.60998735373063));
#27844=CARTESIAN_POINT('Ctrl Pts',(45.7752605333315,2.66597926288907,-4.22144393316328));
#27845=CARTESIAN_POINT('Ctrl Pts',(45.8148968663299,3.27636095055706,-3.67766692215644));
#27846=CARTESIAN_POINT('Ctrl Pts',(45.8545331993282,3.88674263822504,-3.1338899111496));
#27847=CARTESIAN_POINT('Ctrl Pts',(45.8941695323265,4.35882978082128,-2.43487930970328));
#27848=CARTESIAN_POINT('Ctrl Pts',(45.9338058653249,4.63526337679785,-1.6655655184864));
#27849=CARTESIAN_POINT('Ctrl Pts',(45.9734421983232,4.91169697277443,-0.896251727269502));
#27850=CARTESIAN_POINT('Ctrl Pts',(46.0130785313215,4.99247702213132,-0.0566347462819967));
#27851=CARTESIAN_POINT('Ctrl Pts',(46.0527148643198,4.86778867807864,0.751271225473264));
#27852=CARTESIAN_POINT('Ctrl Pts',(46.0923511973181,4.74310033402597,1.5591771972285));
#27853=CARTESIAN_POINT('Ctrl Pts',(46.1319875303164,4.41294359656375,2.33537215975155));
#27854=CARTESIAN_POINT('Ctrl Pts',(46.1716238633147,3.91743279863258,2.98554774486244));
#27855=CARTESIAN_POINT('Ctrl Pts',(46.2112601963131,3.42192200070141,3.63572332997333));
#27856=CARTESIAN_POINT('Ctrl Pts',(46.2508965293114,2.76105714230129,4.15987953767205));
#27857=CARTESIAN_POINT('Ctrl Pts',(46.2905328623097,2.01513388288903,4.4943309293695));
#27858=CARTESIAN_POINT('Ctrl Pts',(46.3301691953081,1.26921062347679,4.82878232106693));
#27859=CARTESIAN_POINT('Ctrl Pts',(46.3698055283064,0.438228963052423,4.9735288967631));
#27860=CARTESIAN_POINT('Ctrl Pts',(46.4094418613047,-0.376846098396358,
4.91098382065942));
#27861=CARTESIAN_POINT('Ctrl Pts',(46.449078194303,-1.19192115984518,4.84843874455575));
#27862=CARTESIAN_POINT('Ctrl Pts',(46.4887145273013,-1.99108962231841,4.5786020166522));
#27863=CARTESIAN_POINT('Ctrl Pts',(46.5283508602997,-2.67725181725943,4.13425903586556));
#27864=CARTESIAN_POINT('Ctrl Pts',(46.567987193298,-3.36341401220043,3.68991605507894));
#27865=CARTESIAN_POINT('Ctrl Pts',(46.6076235262963,-3.93656993960923,3.07106682140923));
#27866=CARTESIAN_POINT('Ctrl Pts',(46.6472598592946,-4.32708065200984,2.35290205908728));
#27867=CARTESIAN_POINT('Ctrl Pts',(46.6868927308952,-4.71755726153596,1.63480001331054));
#27868=CARTESIAN_POINT('Ctrl Pts',(46.7265256024958,-4.92542055507572,0.817399784357684));
#27869=CARTESIAN_POINT('Ctrl Pts',(46.7661584740964,-4.92542130864622,-7.54510065536516E-8));
#27870=CARTESIAN_POINT('Origin',(41.25,0.,0.));
#27871=CARTESIAN_POINT('',(48.4838415259036,-4.92464095784815,-6.78464642470123E-5));
#27872=CARTESIAN_POINT('',(48.2661584740964,-4.924668549948,-8.0469304329367E-5));
#27873=CARTESIAN_POINT('',(41.25,-4.925,-6.03138548580071E-16));
#27874=CARTESIAN_POINT('Ctrl Pts',(48.4838415259036,-4.92464095784815,-6.78464642470123E-5));
#27875=CARTESIAN_POINT('Ctrl Pts',(48.4602893623278,-4.92440377657073,0.485900652092098));
#27876=CARTESIAN_POINT('Ctrl Pts',(48.4367371987521,-4.85294368865689,0.971937392632399));
#27877=CARTESIAN_POINT('Ctrl Pts',(48.4131850351763,-4.71126924513192,1.43656431086514));
#27878=CARTESIAN_POINT('Ctrl Pts',(48.373548702178,-4.47284293653205,2.21849278176001));
#27879=CARTESIAN_POINT('Ctrl Pts',(48.3339123691797,-4.03555488870416,2.93978415837996));
#27880=CARTESIAN_POINT('Ctrl Pts',(48.2942760361814,-3.45253598268484,3.51280090634862));
#27881=CARTESIAN_POINT('Ctrl Pts',(48.2546397031831,-2.86951707666548,4.08581765431731));
#27882=CARTESIAN_POINT('Ctrl Pts',(48.2150033701847,-2.14076731245468,4.51055977363469));
#27883=CARTESIAN_POINT('Ctrl Pts',(48.1753670371864,-1.3548304250574,4.73542072457306));
#27884=CARTESIAN_POINT('Ctrl Pts',(48.1357307041881,-0.568893537660152,
4.96028167551142));
#27885=CARTESIAN_POINT('Ctrl Pts',(48.0960943711898,0.274230472923564,4.98526145807077));
#27886=CARTESIAN_POINT('Ctrl Pts',(48.0564580381915,1.07210130052046,4.80732500677867));
#27887=CARTESIAN_POINT('Ctrl Pts',(48.0168217051931,1.86997212811736,4.62938855548657));
#27888=CARTESIAN_POINT('Ctrl Pts',(47.9771853721948,2.62258977272744,4.24853587034301));
#27889=CARTESIAN_POINT('Ctrl Pts',(47.9375490391965,3.23851053096014,3.71104088636025));
#27890=CARTESIAN_POINT('Ctrl Pts',(47.8979127061982,3.85443128919285,3.17354590237749));
#27891=CARTESIAN_POINT('Ctrl Pts',(47.8582763731999,4.33365516104819,2.47940861955552));
#27892=CARTESIAN_POINT('Ctrl Pts',(47.8186400402016,4.617956026119,1.7129673260773));
#27893=CARTESIAN_POINT('Ctrl Pts',(47.7790037072032,4.90225689118982,0.946526032599082));
#27894=CARTESIAN_POINT('Ctrl Pts',(47.7393673742049,4.99163474947611,0.107780728464605));
#27895=CARTESIAN_POINT('Ctrl Pts',(47.6997310412066,4.87523011286816,-0.701360296823789));
#27896=CARTESIAN_POINT('Ctrl Pts',(47.6600947082082,4.7588254762602,-1.51050132211221));
#27897=CARTESIAN_POINT('Ctrl Pts',(47.6204583752099,4.43663834475798,-2.29003806855454));
#27898=CARTESIAN_POINT('Ctrl Pts',(47.5808220422116,3.94781473719369,-2.94525613829656));
#27899=CARTESIAN_POINT('Ctrl Pts',(47.5411857092133,3.45899112962941,-3.60047420803855));
#27900=CARTESIAN_POINT('Ctrl Pts',(47.501549376215,2.80353104600308,-4.13137360108024));
#27901=CARTESIAN_POINT('Ctrl Pts',(47.4619130432166,2.06107346089987,-4.47344957590353));
#27902=CARTESIAN_POINT('Ctrl Pts',(47.4222767102183,1.31861587579667,-4.81552555072681));
#27903=CARTESIAN_POINT('Ctrl Pts',(47.38264037722,0.489160789216602,-4.9687781073317));
#27904=CARTESIAN_POINT('Ctrl Pts',(47.3430040442217,-0.326512278912506,
-4.91458692578498));
#27905=CARTESIAN_POINT('Ctrl Pts',(47.3033677112234,-1.14218534704164,-4.86039574423825));
#27906=CARTESIAN_POINT('Ctrl Pts',(47.263731378225,-1.94407639671981,-4.59876082453989));
#27907=CARTESIAN_POINT('Ctrl Pts',(47.2240950452267,-2.63475496265902,-4.16147103872187));
#27908=CARTESIAN_POINT('Ctrl Pts',(47.1844587122284,-3.3254335285982,-3.72418125290388));
#27909=CARTESIAN_POINT('Ctrl Pts',(47.1448223792301,-3.90489961079844,-3.11123660096624));
#27910=CARTESIAN_POINT('Ctrl Pts',(47.1051860462318,-4.30274757244656,-2.3971103952848));
#27911=CARTESIAN_POINT('Ctrl Pts',(47.0655497132335,-4.7005955340947,-1.68298418960333));
#27912=CARTESIAN_POINT('Ctrl Pts',(47.0259133802351,-4.91682537519071,-0.867676430178051));
#27913=CARTESIAN_POINT('Ctrl Pts',(46.9862770472368,-4.92516498054441,-0.0502477242891959));
#27914=CARTESIAN_POINT('Ctrl Pts',(46.9854652067924,-4.92533579425003,-0.0335049624427779));
#27915=CARTESIAN_POINT('Ctrl Pts',(46.984653366348,-4.92541939349056,-0.0167613108132938));
#27916=CARTESIAN_POINT('Ctrl Pts',(46.9838415259036,-4.92541598660193,-1.76250313788096E-5));
#27917=CARTESIAN_POINT('Ctrl Pts',(46.7661584740964,-4.92542130864622,-7.54510065536516E-8));
#27918=CARTESIAN_POINT('Ctrl Pts',(46.8057982684924,-4.92542206234836,-0.817542713004385));
#27919=CARTESIAN_POINT('Ctrl Pts',(46.8454380628885,-4.71748324187784,-1.63508498109272));
#27920=CARTESIAN_POINT('Ctrl Pts',(46.8850778572845,-4.32687594630263,-2.35327848202517));
#27921=CARTESIAN_POINT('Ctrl Pts',(46.9247141902829,-3.9363027590578,-3.07140926937937));
#27922=CARTESIAN_POINT('Ctrl Pts',(46.9643505232812,-3.36309299739203,-3.69020863934389));
#27923=CARTESIAN_POINT('Ctrl Pts',(47.0039868562795,-2.67689214969072,-4.13449192617173));
#27924=CARTESIAN_POINT('Ctrl Pts',(47.0436231892778,-1.99069130198939,-4.57877521299958));
#27925=CARTESIAN_POINT('Ctrl Pts',(47.0832595222761,-1.19149936825251,-4.84854241669076));
#27926=CARTESIAN_POINT('Ctrl Pts',(47.1228958552744,-0.376418868815787,
-4.91101658558128));
#27927=CARTESIAN_POINT('Ctrl Pts',(47.1625321882728,0.438661630620939,-4.97349075447181));
#27928=CARTESIAN_POINT('Ctrl Pts',(47.2021685212711,1.26963069575751,-4.82867188856169));
#27929=CARTESIAN_POINT('Ctrl Pts',(47.2418048542694,2.01552485694469,-4.49415560697369));
#27930=CARTESIAN_POINT('Ctrl Pts',(47.2814411872677,2.7614190181319,-4.15963932538569));
#27931=CARTESIAN_POINT('Ctrl Pts',(47.3210775202661,3.4222382753697,-3.6354256281198));
#27932=CARTESIAN_POINT('Ctrl Pts',(47.3607138532644,3.9176925097825,-2.98520693879824));
#27933=CARTESIAN_POINT('Ctrl Pts',(47.4003501862627,4.41314674419528,-2.33498824947669));
#27934=CARTESIAN_POINT('Ctrl Pts',(47.439986519261,4.74323595578306,-1.55876456809948));
#27935=CARTESIAN_POINT('Ctrl Pts',(47.4796228522593,4.86785401605814,-0.750847752211934));
#27936=CARTESIAN_POINT('Ctrl Pts',(47.5192591852577,4.99247207633321,0.0570690636756077));
#27937=CARTESIAN_POINT('Ctrl Pts',(47.558895518256,4.91161898529556,0.896679014073474));
#27938=CARTESIAN_POINT('Ctrl Pts',(47.5985318512543,4.63511846436338,1.66596875420057));
#27939=CARTESIAN_POINT('Ctrl Pts',(47.6381681842526,4.35861794343121,2.43525849432767));
#27940=CARTESIAN_POINT('Ctrl Pts',(47.6778045172509,3.8864699926045,3.13422802418401));
#27941=CARTESIAN_POINT('Ctrl Pts',(47.7174408502492,3.27604100168431,3.67795193333712));
#27942=CARTESIAN_POINT('Ctrl Pts',(47.7570771832476,2.66561201076412,4.22167584249024));
#27943=CARTESIAN_POINT('Ctrl Pts',(47.7967135162459,1.91690197975045,4.61015413094014));
#27944=CARTESIAN_POINT('Ctrl Pts',(47.8363498492442,1.12087983355739,4.79618634619));
#27945=CARTESIAN_POINT('Ctrl Pts',(47.8759861822425,0.324857687364301,4.98221856143987));
#27946=CARTESIAN_POINT('Ctrl Pts',(47.9156225152409,-0.518476574008187,
4.96580470348969));
#27947=CARTESIAN_POINT('Ctrl Pts',(47.9552588482392,-1.3066570987317,4.74893907046501));
#27948=CARTESIAN_POINT('Ctrl Pts',(47.9948951812375,-2.09483762345518,4.53207343744033));
#27949=CARTESIAN_POINT('Ctrl Pts',(48.0345315142358,-2.8278644115297,4.11475602934116));
#27950=CARTESIAN_POINT('Ctrl Pts',(48.0741678472342,-3.41667406580256,3.54769127697538));
#27951=CARTESIAN_POINT('Ctrl Pts',(48.1138041802325,-4.00548372007542,2.98062652460961));
#27952=CARTESIAN_POINT('Ctrl Pts',(48.1534405132308,-4.45007624054664,2.26381442797724));
#27953=CARTESIAN_POINT('Ctrl Pts',(48.1930768462291,-4.69643324635205,1.48434828501067));
#27954=CARTESIAN_POINT('Ctrl Pts',(48.2174373888515,-4.84784458757054,1.00528736382791));
#27955=CARTESIAN_POINT('Ctrl Pts',(48.241797931474,-4.9243754795075,0.502559829996446));
#27956=CARTESIAN_POINT('Ctrl Pts',(48.2661584740964,-4.924668549948,-8.0469304329367E-5));
#27957=CARTESIAN_POINT('Origin',(41.25,0.,0.));
#27958=CARTESIAN_POINT('',(49.9838415259036,-4.92505697724291,0.000124540890093713));
#27959=CARTESIAN_POINT('',(49.7661584740964,-4.92500433765405,0.000126715614453391));
#27960=CARTESIAN_POINT('',(41.25,-4.925,-6.03138548580071E-16));
#27961=CARTESIAN_POINT('Ctrl Pts',(49.9838415259036,-4.92505697724291,0.000124540890093713));
#27962=CARTESIAN_POINT('Ctrl Pts',(49.975561691306,-4.92523258911014,0.170926810624905));
#27963=CARTESIAN_POINT('Ctrl Pts',(49.9672818567084,-4.91652003640936,0.341711252245115));
#27964=CARTESIAN_POINT('Ctrl Pts',(49.9590020221109,-4.8987843370784,0.511553455647789));
#27965=CARTESIAN_POINT('Ctrl Pts',(49.9193656891125,-4.81388190619586,1.32460377107337));
#27966=CARTESIAN_POINT('Ctrl Pts',(49.8797293561142,-4.52220276134002,2.11606151681266));
#27967=CARTESIAN_POINT('Ctrl Pts',(49.8400930231159,-4.05918617416124,2.78976388302373));
#27968=CARTESIAN_POINT('Ctrl Pts',(49.8004566901176,-3.59616958698247,3.46346624923481));
#27969=CARTESIAN_POINT('Ctrl Pts',(49.7608203571192,-2.96181555748075,4.01941323591768));
#27970=CARTESIAN_POINT('Ctrl Pts',(49.7211840241209,-2.23319865620258,4.39005679703905));
#27971=CARTESIAN_POINT('Ctrl Pts',(49.6815476911226,-1.5045817549244,4.76070035816043));
#27972=CARTESIAN_POINT('Ctrl Pts',(49.6419113581243,-0.68170198186976,4.9460404937203));
#27973=CARTESIAN_POINT('Ctrl Pts',(49.602275025126,0.135460049406341,4.92355821479023));
#27974=CARTESIAN_POINT('Ctrl Pts',(49.5626386921276,0.952622080682418,4.90107593586015));
#27975=CARTESIAN_POINT('Ctrl Pts',(49.5230023591293,1.76406637017997,4.67077124244014));
#27976=CARTESIAN_POINT('Ctrl Pts',(49.483366026131,2.4712017255922,4.26062635662838));
#27977=CARTESIAN_POINT('Ctrl Pts',(49.4437296931327,3.17833708100444,3.85048147081662));
#27978=CARTESIAN_POINT('Ctrl Pts',(49.4040933601344,3.78116350233136,3.2604963926131));
#27979=CARTESIAN_POINT('Ctrl Pts',(49.364457027136,4.20643705108794,2.56235482605598));
#27980=CARTESIAN_POINT('Ctrl Pts',(49.3248206941377,4.63171059984453,1.86421325949884));
#27981=CARTESIAN_POINT('Ctrl Pts',(49.2851843611394,4.87943127603075,1.05791520458814));
#27982=CARTESIAN_POINT('Ctrl Pts',(49.2455480281411,4.91950080039325,0.241426581613654));
#27983=CARTESIAN_POINT('Ctrl Pts',(49.2059116951428,4.95957032475575,-0.575062041360806));
#27984=CARTESIAN_POINT('Ctrl Pts',(49.1662753621445,4.79198869729451,-1.40174123239899));
#27985=CARTESIAN_POINT('Ctrl Pts',(49.1266390291461,4.43711723261043,-2.13816874531611));
#27986=CARTESIAN_POINT('Ctrl Pts',(49.0870026961478,4.08224576792633,-2.87459625823325));
#27987=CARTESIAN_POINT('Ctrl Pts',(49.0473663631494,3.54008446601938,-3.52077209302934));
#27988=CARTESIAN_POINT('Ctrl Pts',(49.0077300301511,2.87650640020383,-3.99818531948745));
#27989=CARTESIAN_POINT('Ctrl Pts',(48.9680936971528,2.2129283343883,-4.47559854594555));
#27990=CARTESIAN_POINT('Ctrl Pts',(48.9284573641545,1.42793350466419,-4.7842491640657));
#27991=CARTESIAN_POINT('Ctrl Pts',(48.8888210311562,0.616899470788016,-4.88663585325509));
#27992=CARTESIAN_POINT('Ctrl Pts',(48.8491846981579,-0.194134563088155,
-4.98902254244449));
#27993=CARTESIAN_POINT('Ctrl Pts',(48.8095483651595,-1.03120780111639,-4.88514530270314));
#27994=CARTESIAN_POINT('Ctrl Pts',(48.7699120321612,-1.79261511129173,-4.58762530969411));
#27995=CARTESIAN_POINT('Ctrl Pts',(48.7302756991629,-2.55402242146707,-4.29010531668508));
#27996=CARTESIAN_POINT('Ctrl Pts',(48.6906393661646,-3.23976380378953,-3.79894257040838));
#27997=CARTESIAN_POINT('Ctrl Pts',(48.6510030331663,-3.76652107934467,-3.17381377497632));
#27998=CARTESIAN_POINT('Ctrl Pts',(48.6113667001679,-4.29327835489981,-2.54868497954427));
#27999=CARTESIAN_POINT('Ctrl Pts',(48.5717303671696,-4.66105152368764,-1.78959013495686));
#28000=CARTESIAN_POINT('Ctrl Pts',(48.5320940341713,-4.82515582339564,-0.98875993007825));
#28001=CARTESIAN_POINT('Ctrl Pts',(48.5160098647487,-4.89174829448995,-0.663788175135068));
#28002=CARTESIAN_POINT('Ctrl Pts',(48.4999256953262,-4.92480293293963,-0.331943923991882));
#28003=CARTESIAN_POINT('Ctrl Pts',(48.4838415259036,-4.92464095784815,-6.78464642470123E-5));
#28004=CARTESIAN_POINT('Ctrl Pts',(48.2661584740964,-4.924668549948,-8.0469304329367E-5));
#28005=CARTESIAN_POINT('Ctrl Pts',(48.2814342644723,-4.92485232592885,-0.315271635839327));
#28006=CARTESIAN_POINT('Ctrl Pts',(48.2967100548482,-4.89505801306927,-0.630428500180749));
#28007=CARTESIAN_POINT('Ctrl Pts',(48.311985845224,-4.83495091642528,-0.939693941883922));
#28008=CARTESIAN_POINT('Ctrl Pts',(48.3516221782224,-4.67899008955348,-1.74214983651119));
#28009=CARTESIAN_POINT('Ctrl Pts',(48.3912585112207,-4.31894694467024,-2.50494143646496));
#28010=CARTESIAN_POINT('Ctrl Pts',(48.430894844219,-3.79856703940939,-3.1353888938643));
#28011=CARTESIAN_POINT('Ctrl Pts',(48.4705311772174,-3.27818713414853,-3.76583635126364));
#28012=CARTESIAN_POINT('Ctrl Pts',(48.5101675102157,-2.59747046851005,-4.26393966610853));
#28013=CARTESIAN_POINT('Ctrl Pts',(48.549803843214,-1.83912471392769,-4.56917884912326));
#28014=CARTESIAN_POINT('Ctrl Pts',(48.5894401762123,-1.08077895934533,-4.87441803213799));
#28015=CARTESIAN_POINT('Ctrl Pts',(48.6290765092106,-0.244804115819099,
-4.98679308332255));
#28016=CARTESIAN_POINT('Ctrl Pts',(48.6687128422089,0.567228140540522,-4.89265033547606));
#28017=CARTESIAN_POINT('Ctrl Pts',(48.7083491752073,1.37926039690017,-4.79850758762956));
#28018=CARTESIAN_POINT('Ctrl Pts',(48.7479855082056,2.16735006609319,-4.49784704075199));
#28019=CARTESIAN_POINT('Ctrl Pts',(48.7876218412039,2.83574356265565,-4.02719921477844));
#28020=CARTESIAN_POINT('Ctrl Pts',(48.8272581742023,3.50413705921809,-3.55655138880489));
#28021=CARTESIAN_POINT('Ctrl Pts',(48.8668945072006,4.05283438314997,-2.91591628373537));
#28022=CARTESIAN_POINT('Ctrl Pts',(48.9065308401989,4.41516832873248,-2.18313162626826));
#28023=CARTESIAN_POINT('Ctrl Pts',(48.9461671731972,4.77750227431499,-1.45034696880114));
#28024=CARTESIAN_POINT('Ctrl Pts',(48.9858035061955,4.95347284154814,-0.62541275893643));
#28025=CARTESIAN_POINT('Ctrl Pts',(49.0254398391939,4.92169945229804,0.191440773880888));
#28026=CARTESIAN_POINT('Ctrl Pts',(49.0650761721922,4.88992606304794,1.00829430669821));
#28027=CARTESIAN_POINT('Ctrl Pts',(49.1047125051905,4.6504087173146,1.81706716246813));
#28028=CARTESIAN_POINT('Ctrl Pts',(49.1443488381888,4.23224898251004,2.5194927304316));
#28029=CARTESIAN_POINT('Ctrl Pts',(49.1839851711871,3.81408924770549,3.22191829839507));
#28030=CARTESIAN_POINT('Ctrl Pts',(49.2236215041854,3.21728712382973,3.81799657855207));
#28031=CARTESIAN_POINT('Ctrl Pts',(49.2632578371838,2.51435459195233,4.23530353747916));
#28032=CARTESIAN_POINT('Ctrl Pts',(49.3028941701821,1.81142206007491,4.65261049640625));
#28033=CARTESIAN_POINT('Ctrl Pts',(49.3425305031804,1.00235912019584,4.89114613410341));
#28034=CARTESIAN_POINT('Ctrl Pts',(49.3821668361787,0.185467628547644,4.92192816154557));
#28035=CARTESIAN_POINT('Ctrl Pts',(49.4218031691771,-0.631423863100528,
4.95271018898772));
#28036=CARTESIAN_POINT('Ctrl Pts',(49.4614395021754,-1.45614390651782,4.77573860617489));
#28037=CARTESIAN_POINT('Ctrl Pts',(49.5010758351737,-2.18848829367015,4.41251561551062));
#28038=CARTESIAN_POINT('Ctrl Pts',(49.540712168172,-2.92083268082247,4.04929262484635));
#28039=CARTESIAN_POINT('Ctrl Pts',(49.5803485011703,-3.56080141170983,3.49981822633064));
#28040=CARTESIAN_POINT('Ctrl Pts',(49.6199848341686,-4.03063772468131,2.83085404092629));
#28041=CARTESIAN_POINT('Ctrl Pts',(49.659621167167,-4.50047403765279,2.16188985552195));
#28042=CARTESIAN_POINT('Ctrl Pts',(49.6992575001653,-4.8001779327084,1.37343588322897));
#28043=CARTESIAN_POINT('Ctrl Pts',(49.7388938331636,-4.89333512394708,0.561289972655089));
#28044=CARTESIAN_POINT('Ctrl Pts',(49.7479820468079,-4.9146951336259,0.375073060360803));
#28045=CARTESIAN_POINT('Ctrl Pts',(49.7570702604521,-4.92519617945162,0.18761057069032));
#28046=CARTESIAN_POINT('Ctrl Pts',(49.7661584740964,-4.92500433765405,0.000126715614453391));
#28047=CARTESIAN_POINT('Origin',(41.25,0.,0.));
#28048=CARTESIAN_POINT('',(51.4838415259036,-4.9251402971202,-0.000116503725961781));
#28049=CARTESIAN_POINT('',(51.2661584740964,-4.92519062564324,-0.000109311139069327));
#28050=CARTESIAN_POINT('',(41.25,-4.925,-6.03138548580071E-16));
#28051=CARTESIAN_POINT('Ctrl Pts',(51.4838415259036,-4.9251402971202,-0.000116503725961781));
#28052=CARTESIAN_POINT('Ctrl Pts',(51.4511976872858,-4.9244646577768,0.67325086546852));
#28053=CARTESIAN_POINT('Ctrl Pts',(51.4185538486681,-4.78528364631617,1.34688857405293));
#28054=CARTESIAN_POINT('Ctrl Pts',(51.3859100100504,-4.51678498406586,1.96428798565576));
#28055=CARTESIAN_POINT('Ctrl Pts',(51.3462736770521,-4.19077239372136,2.71393783406419));
#28056=CARTESIAN_POINT('Ctrl Pts',(51.3066373440537,-3.67410739356836,3.38067582335991));
#28057=CARTESIAN_POINT('Ctrl Pts',(51.2670010110554,-3.02956496398235,3.88349220413633));
#28058=CARTESIAN_POINT('Ctrl Pts',(51.2273646780571,-2.38502253439632,4.38630858491276));
#28059=CARTESIAN_POINT('Ctrl Pts',(51.1877283450588,-1.61260267537726,4.7252033571699));
#28060=CARTESIAN_POINT('Ctrl Pts',(51.1480920120604,-0.806155212049699,
4.85900075945319));
#28061=CARTESIAN_POINT('Ctrl Pts',(51.1084556790621,0.000292251277839023,
4.99279816173648));
#28062=CARTESIAN_POINT('Ctrl Pts',(51.0688193460638,0.840767318913887,4.92149819404594));
#28063=CARTESIAN_POINT('Ctrl Pts',(51.0291830130655,1.61315160142145,4.65376373941843));
#28064=CARTESIAN_POINT('Ctrl Pts',(50.9895466800672,2.38553588392901,4.38602928479092));
#28065=CARTESIAN_POINT('Ctrl Pts',(50.9499103470689,3.0898293813081,3.92186034322643));
#28066=CARTESIAN_POINT('Ctrl Pts',(50.9102740140705,3.64045978239183,3.31765391083831));
#28067=CARTESIAN_POINT('Ctrl Pts',(50.8706376810722,4.19109018347557,2.7134474784502));
#28068=CARTESIAN_POINT('Ctrl Pts',(50.8310013480739,4.58805748826396,1.96920355523843));
#28069=CARTESIAN_POINT('Ctrl Pts',(50.7913650150756,4.78312983838864,1.17534839855546));
#28070=CARTESIAN_POINT('Ctrl Pts',(50.7517286820773,4.97820218851332,0.381493241872491));
#28071=CARTESIAN_POINT('Ctrl Pts',(50.7120923490789,4.9713795839743,-0.461973148281703));
#28072=CARTESIAN_POINT('Ctrl Pts',(50.6724560160806,4.76349096865269,-1.25256885049863));
#28073=CARTESIAN_POINT('Ctrl Pts',(50.6328196830823,4.55560235333107,-2.04316455271558));
#28074=CARTESIAN_POINT('Ctrl Pts',(50.593183350084,4.14664772722689,-2.7808895669952));
#28075=CARTESIAN_POINT('Ctrl Pts',(50.5535470170856,3.58631544009297,-3.37610966551359));
#28076=CARTESIAN_POINT('Ctrl Pts',(50.5139106840873,3.02598315295906,-3.97132976403196));
#28077=CARTESIAN_POINT('Ctrl Pts',(50.474274351089,2.31427320479544,-4.42404494678905));
#28078=CARTESIAN_POINT('Ctrl Pts',(50.4346380180907,1.53765897587531,-4.67924991835887));
#28079=CARTESIAN_POINT('Ctrl Pts',(50.3950016850924,0.761044746955179,-4.93445488992869));
#28080=CARTESIAN_POINT('Ctrl Pts',(50.355365352094,-0.0804737627214679,
-4.99214965031124));
#28081=CARTESIAN_POINT('Ctrl Pts',(50.3157290190957,-0.884651315671221,
-4.84532423755135));
#28082=CARTESIAN_POINT('Ctrl Pts',(50.2760926860974,-1.68882886862102,-4.69849882479145));
#28083=CARTESIAN_POINT('Ctrl Pts',(50.2364563530991,-2.45566546484393,-4.34715323888908));
#28084=CARTESIAN_POINT('Ctrl Pts',(50.1968200201008,-3.0919897864075,-3.83397627544034));
#28085=CARTESIAN_POINT('Ctrl Pts',(50.1571836871025,-3.72831410797102,-3.32079931199164));
#28086=CARTESIAN_POINT('Ctrl Pts',(50.1175473541041,-4.23412615487522,-2.64579097099658));
#28087=CARTESIAN_POINT('Ctrl Pts',(50.0779110211058,-4.5479693198727,-1.89096535794314));
#28088=CARTESIAN_POINT('Ctrl Pts',(50.0465545227051,-4.79625219462155,-1.29381909495384));
#28089=CARTESIAN_POINT('Ctrl Pts',(50.0151980243043,-4.92439191888106,-0.646719431010621));
#28090=CARTESIAN_POINT('Ctrl Pts',(49.9838415259036,-4.92505697724291,0.000124540890093713));
#28091=CARTESIAN_POINT('Ctrl Pts',(49.7661584740964,-4.92500433765405,0.000126715614453391));
#28092=CARTESIAN_POINT('Ctrl Pts',(49.7967065934505,-4.92435950178655,-0.630060844448721));
#28093=CARTESIAN_POINT('Ctrl Pts',(49.8272547128045,-4.8029035475925,-1.26048979660438));
#28094=CARTESIAN_POINT('Ctrl Pts',(49.8578028321585,-4.56694351136301,-1.84466854276718));
#28095=CARTESIAN_POINT('Ctrl Pts',(49.8974391651569,-4.26078422011854,-2.6026432987608));
#28096=CARTESIAN_POINT('Ctrl Pts',(49.9370754981552,-3.76185515020785,-3.28275496189324));
#28097=CARTESIAN_POINT('Ctrl Pts',(49.9767118311536,-3.1307766208679,-3.80236936907387));
#28098=CARTESIAN_POINT('Ctrl Pts',(50.0163481641519,-2.49969809152796,-4.3219837762545));
#28099=CARTESIAN_POINT('Ctrl Pts',(50.0559844971501,-1.73647010275876,-4.68110092748333));
#28100=CARTESIAN_POINT('Ctrl Pts',(50.0956208301485,-0.93382552407062,-4.83608777415021));
#28101=CARTESIAN_POINT('Ctrl Pts',(50.1352571631468,-0.131180945382506,
-4.99107462081708));
#28102=CARTESIAN_POINT('Ctrl Pts',(50.1748934961451,0.710880223224554,-4.94193116292202));
#28103=CARTESIAN_POINT('Ctrl Pts',(50.2145298291435,1.49004681182054,-4.69462837370072));
#28104=CARTESIAN_POINT('Ctrl Pts',(50.2541661621418,2.26921340041652,-4.44732558447941));
#28105=CARTESIAN_POINT('Ctrl Pts',(50.2938024951401,2.98548540900144,-4.00186346393186));
#28106=CARTESIAN_POINT('Ctrl Pts',(50.3334388281384,3.55183516079068,-3.41236605002642));
#28107=CARTESIAN_POINT('Ctrl Pts',(50.3730751611367,4.11818491257993,-2.82286863612097));
#28108=CARTESIAN_POINT('Ctrl Pts',(50.412711494135,4.5346124075735,-2.08933592885763));
#28109=CARTESIAN_POINT('Ctrl Pts',(50.4523478271334,4.75052134023217,-1.3008927951479));
#28110=CARTESIAN_POINT('Ctrl Pts',(50.4919841601317,4.96643027289085,-0.512449661438156));
#28111=CARTESIAN_POINT('Ctrl Pts',(50.53162049313,4.98182064321461,0.330903898717918));
#28112=CARTESIAN_POINT('Ctrl Pts',(50.5712568261284,4.79482250762883,1.12669968894037));
#28113=CARTESIAN_POINT('Ctrl Pts',(50.6108931591267,4.60782437204306,1.92249547916279));
#28114=CARTESIAN_POINT('Ctrl Pts',(50.650529492125,4.21843773054774,2.67073349945155));
#28115=CARTESIAN_POINT('Ctrl Pts',(50.6901658251233,3.67397340151565,3.28050217407564));
#28116=CARTESIAN_POINT('Ctrl Pts',(50.7298021581216,3.12950907248357,3.89027084869974));
#28117=CARTESIAN_POINT('Ctrl Pts',(50.7694384911199,2.42996705591471,4.36157017765919));
#28118=CARTESIAN_POINT('Ctrl Pts',(50.8090748241183,1.66034231950991,4.63713688051827));
#28119=CARTESIAN_POINT('Ctrl Pts',(50.8487111571166,0.890717583105111,4.91270358337736));
#28120=CARTESIAN_POINT('Ctrl Pts',(50.8883474901149,0.051010126864362,4.99253766013608));
#28121=CARTESIAN_POINT('Ctrl Pts',(50.9279838231132,-0.756754856649776,
4.86693919837959));
#28122=CARTESIAN_POINT('Ctrl Pts',(50.9676201561115,-1.56451984016391,4.74134073662311));
#28123=CARTESIAN_POINT('Ctrl Pts',(51.0072564891099,-2.34034235095145,4.41030973635142));
#28124=CARTESIAN_POINT('Ctrl Pts',(51.0468928221082,-2.98995927551403,3.91406675844198));
#28125=CARTESIAN_POINT('Ctrl Pts',(51.0865291551065,-3.63957620007659,3.41782378053256));
#28126=CARTESIAN_POINT('Ctrl Pts',(51.1261654881048,-4.16298753841419,2.75636882498538));
#28127=CARTESIAN_POINT('Ctrl Pts',(51.1658018211031,-4.49659835128688,2.01006924011891));
#28128=CARTESIAN_POINT('Ctrl Pts',(51.1992540387675,-4.77815874507751,1.38020834564911));
#28129=CARTESIAN_POINT('Ctrl Pts',(51.232706256432,-4.92452424115612,0.689912629125271));
#28130=CARTESIAN_POINT('Ctrl Pts',(51.2661584740964,-4.92519062564324,-0.000109311139069327));
#28131=CARTESIAN_POINT('Origin',(27.2271873309261,0.,0.));
#28132=CARTESIAN_POINT('',(51.9771873309261,-4.07061595521377,-9.62900340455034E-5));
#28133=CARTESIAN_POINT('',(52.2728126690739,-4.07017027259505,4.41422946496905E-5));
#28134=CARTESIAN_POINT('',(27.2271873309261,-4.0705,-3.42898509504556E-13));
#28135=CARTESIAN_POINT('',(52.575,3.27123862564629,-2.42269060785926));
#28136=CARTESIAN_POINT('Ctrl Pts',(51.9771873309261,-4.07061595521377,-9.62900340453765E-5));
#28137=CARTESIAN_POINT('Ctrl Pts',(51.9841798253067,-4.07073557068603,-0.119309531040752));
#28138=CARTESIAN_POINT('Ctrl Pts',(52.0308086526856,-4.03650707267767,-0.914204069448567));
#28139=CARTESIAN_POINT('Ctrl Pts',(52.1170738130629,-3.53493171453767,-2.34618303073278));
#28140=CARTESIAN_POINT('Ctrl Pts',(52.2359828120577,-1.98456277868761,-3.74990797127371));
#28141=CARTESIAN_POINT('Ctrl Pts',(52.3548918110528,0.0480654662789952,
-4.24241179250651));
#28142=CARTESIAN_POINT('Ctrl Pts',(52.4678975403668,1.96866977915683,-3.73070679305914));
#28143=CARTESIAN_POINT('Ctrl Pts',(52.5412669366826,2.92852672977728,-2.88450285218581));
#28144=CARTESIAN_POINT('Ctrl Pts',(52.575,3.27123862564629,-2.42269060785926));
#28145=CARTESIAN_POINT('',(52.575,-1.2223317023727,-3.88263769354992));
#28146=CARTESIAN_POINT('Origin',(52.575,0.,0.));
#28147=CARTESIAN_POINT('Ctrl Pts',(52.2728126690739,-4.07017027259505,4.4142294649864E-5));
#28148=CARTESIAN_POINT('Ctrl Pts',(52.294269113386,-4.07009408388197,-0.365864931681719));
#28149=CARTESIAN_POINT('Ctrl Pts',(52.3553618906963,-3.93089510915561,-1.40778868062961));
#28150=CARTESIAN_POINT('Ctrl Pts',(52.456091001005,-3.05253321900086,-2.94673237789893));
#28151=CARTESIAN_POINT('Ctrl Pts',(52.5353636670017,-1.86695937376299,-3.67969605923878));
#28152=CARTESIAN_POINT('Ctrl Pts',(52.575,-1.2223317023727,-3.88263769354992));
#28153=CARTESIAN_POINT('Origin',(27.2271873309261,0.,0.));
#28154=CARTESIAN_POINT('',(50.4771873309261,-4.07054709154665,0.000102932729394074));
#28155=CARTESIAN_POINT('',(50.7728126690739,-4.07065755161032,-9.03453792341913E-5));
#28156=CARTESIAN_POINT('',(27.2271873309261,-4.0705,-3.42898509504556E-13));
#28157=CARTESIAN_POINT('Ctrl Pts',(50.4771873309261,-4.07054709154665,0.000102932729393948));
#28158=CARTESIAN_POINT('Ctrl Pts',(50.5085438293269,-4.06999742249853,-0.53451196831054));
#28159=CARTESIAN_POINT('Ctrl Pts',(50.5795366607259,-3.83021781331726,-1.74538787286129));
#28160=CARTESIAN_POINT('Ctrl Pts',(50.6901658251233,-2.66338977453238,-3.3025248835498));
#28161=CARTESIAN_POINT('Ctrl Pts',(50.8090748241182,-0.762024273055086,
-4.17368358857445));
#28162=CARTESIAN_POINT('Ctrl Pts',(50.9279838231132,1.32451446418683,-4.03062986950608));
#28163=CARTESIAN_POINT('Ctrl Pts',(51.0468928221082,3.08919386154722,-2.90812602092978));
#28164=CARTESIAN_POINT('Ctrl Pts',(51.1658018211032,4.10319374310485,-1.07894246521889));
#28165=CARTESIAN_POINT('Ctrl Pts',(51.2847108200981,4.12011033911056,1.01242602683551));
#28166=CARTESIAN_POINT('Ctrl Pts',(51.4036198190931,3.13583292948141,2.85777316760714));
#28167=CARTESIAN_POINT('Ctrl Pts',(51.522528818088,1.38954256537078,4.00867652393499));
#28168=CARTESIAN_POINT('Ctrl Pts',(51.641437817083,-0.694408965276457,4.18546425093048));
#28169=CARTESIAN_POINT('Ctrl Pts',(51.760346816078,-2.60961812434468,3.34517724353594));
#28170=CARTESIAN_POINT('Ctrl Pts',(51.8722633206923,-3.81535137102011,1.78922094636592));
#28171=CARTESIAN_POINT('Ctrl Pts',(51.9445434923084,-4.07005754101129,0.556440131551016));
#28172=CARTESIAN_POINT('Ctrl Pts',(51.9771873309261,-4.07061595521377,-9.62900340453765E-5));
#28173=CARTESIAN_POINT('Ctrl Pts',(50.7728126690739,-4.07065755161032,-9.03453792342607E-5));
#28174=CARTESIAN_POINT('Ctrl Pts',(50.7789967844078,-4.07075936832261,-0.105518617986562));
#28175=CARTESIAN_POINT('Ctrl Pts',(50.82481723274,-4.04102179465801,-0.886619249492749));
#28176=CARTESIAN_POINT('Ctrl Pts',(50.9102740140706,-3.55858319850174,-2.31015180666798));
#28177=CARTESIAN_POINT('Ctrl Pts',(51.0291830130655,-2.02255111411372,-3.72955803196629));
#28178=CARTESIAN_POINT('Ctrl Pts',(51.1480920120605,0.00496435909204525,
-4.24267489657216));
#28179=CARTESIAN_POINT('Ctrl Pts',(51.2670010110554,2.03127363780405,-3.72481476796509));
#28180=CARTESIAN_POINT('Ctrl Pts',(51.3859100100504,3.56397955602096,-2.30181723828556));
#28181=CARTESIAN_POINT('Ctrl Pts',(51.5048190090453,4.23063280642202,-0.3194758487847));
#28182=CARTESIAN_POINT('Ctrl Pts',(51.6237280080403,3.86923365048362,1.74050225085362));
#28183=CARTESIAN_POINT('Ctrl Pts',(51.7426370070353,2.56760636844359,3.37752823139821));
#28184=CARTESIAN_POINT('Ctrl Pts',(51.8615460060302,0.642041384412004,4.19382294217941));
#28185=CARTESIAN_POINT('Ctrl Pts',(51.9804550050252,-1.43953109567099,3.99098337113032));
#28186=CARTESIAN_POINT('Ctrl Pts',(52.0993640040201,-3.17131432296482,2.81838363574518));
#28187=CARTESIAN_POINT('Ctrl Pts',(52.196816558703,-3.95899732867403,1.29599053439507));
#28188=CARTESIAN_POINT('Ctrl Pts',(52.2546327803876,-4.07023482673565,0.310076230437316));
#28189=CARTESIAN_POINT('Ctrl Pts',(52.2728126690739,-4.07017027259505,4.4142294649864E-5));
#28190=CARTESIAN_POINT('Origin',(27.2271873309261,0.,0.));
#28191=CARTESIAN_POINT('',(48.9771873309261,-4.07020325257277,-5.60749305029008E-5));
#28192=CARTESIAN_POINT('',(49.2728126690739,-4.07050358506006,0.000104730133326306));
#28193=CARTESIAN_POINT('',(27.2271873309261,-4.0705,-3.42898509504556E-13));
#28194=CARTESIAN_POINT('Ctrl Pts',(48.9771873309261,-4.07020325257276,-5.60749305029626E-5));
#28195=CARTESIAN_POINT('Ctrl Pts',(48.9932715003487,-4.07033712457477,-0.274350810682044));
#28196=CARTESIAN_POINT('Ctrl Pts',(49.0489920027697,-3.9756937275254,-1.22450088620951));
#28197=CARTESIAN_POINT('Ctrl Pts',(49.1443488381888,-3.24442007311038,-2.73387162926461));
#28198=CARTESIAN_POINT('Ctrl Pts',(49.2632578371838,-1.54412953702292,-3.95170591883982));
#28199=CARTESIAN_POINT('Ctrl Pts',(49.3821668361787,0.531387183013984,-4.209268743835));
#28200=CARTESIAN_POINT('Ctrl Pts',(49.5010758351737,2.47777588619694,-3.44397188633769));
#28201=CARTESIAN_POINT('Ctrl Pts',(49.6199848341686,3.82206070614344,-1.84178382408138));
#28202=CARTESIAN_POINT('Ctrl Pts',(49.7388938331636,4.23757807543132,0.207960935586202));
#28203=CARTESIAN_POINT('Ctrl Pts',(49.8578028321586,3.62335654502556,2.20717082341209));
#28204=CARTESIAN_POINT('Ctrl Pts',(49.9767118311535,2.12865302339433,3.6700343325455));
#28205=CARTESIAN_POINT('Ctrl Pts',(50.0956208301485,0.11668308609495,4.24107306629136));
#28206=CARTESIAN_POINT('Ctrl Pts',(50.2145298291435,-1.92364104561195,3.78152361138994));
#28207=CARTESIAN_POINT('Ctrl Pts',(50.3334388281384,-3.49651703165463,2.40305729100861));
#28208=CARTESIAN_POINT('Ctrl Pts',(50.4209913287327,-4.02901994529592,0.95813548887407));
#28209=CARTESIAN_POINT('Ctrl Pts',(50.4689074963286,-4.07069223430921,0.141270575156956));
#28210=CARTESIAN_POINT('Ctrl Pts',(50.4771873309261,-4.07054709154665,0.000102932729393948));
#28211=CARTESIAN_POINT('Ctrl Pts',(49.2728126690739,-4.07050358506006,0.000104730133326219));
#28212=CARTESIAN_POINT('Ctrl Pts',(49.3033607884279,-4.06997062985216,-0.520743688797961));
#28213=CARTESIAN_POINT('Ctrl Pts',(49.3735452407803,-3.83934011354282,-1.71785383211517));
#28214=CARTESIAN_POINT('Ctrl Pts',(49.483366026131,-2.69680012382729,-3.27529920754662));
#28215=CARTESIAN_POINT('Ctrl Pts',(49.6022750251259,-0.804382137054723,
-4.16572744962391));
#28216=CARTESIAN_POINT('Ctrl Pts',(49.7211840241209,1.28350211887322,-4.04387661996188));
#28217=CARTESIAN_POINT('Ctrl Pts',(49.8400930231158,3.05949311031172,-2.93935668390779));
#28218=CARTESIAN_POINT('Ctrl Pts',(49.9590020221109,4.09202191338058,-1.12056792152273));
#28219=CARTESIAN_POINT('Ctrl Pts',(50.0779110211058,4.13018221941277,0.970520809410563));
#28220=CARTESIAN_POINT('Ctrl Pts',(50.1968200201008,3.16470100669801,2.82577128347271));
#28221=CARTESIAN_POINT('Ctrl Pts',(50.3157290190956,1.43019190307756,3.99435438105406));
#28222=CARTESIAN_POINT('Ctrl Pts',(50.4346380180907,-0.651856340959766,
4.1923023665036));
#28223=CARTESIAN_POINT('Ctrl Pts',(50.5535470170856,-2.57550234917945,3.37151352187054));
#28224=CARTESIAN_POINT('Ctrl Pts',(50.6662719007468,-3.8058022184373,1.81673645511013));
#28225=CARTESIAN_POINT('Ctrl Pts',(50.7393604514094,-4.07010678652308,0.570211036924561));
#28226=CARTESIAN_POINT('Ctrl Pts',(50.7728126690739,-4.07065755161032,-9.03453792342607E-5));
#28227=CARTESIAN_POINT('Origin',(27.2271873309261,0.,0.));
#28228=CARTESIAN_POINT('',(47.4771873309261,-4.0708438118707,-1.45670437023455E-5));
#28229=CARTESIAN_POINT('',(47.7728126690739,-4.07022605737327,-6.65076761975636E-5));
#28230=CARTESIAN_POINT('',(27.2271873309261,-4.0705,-3.42898509504556E-13));
#28231=CARTESIAN_POINT('Ctrl Pts',(47.4771873309261,-4.0708438118707,-1.4567043702333E-5));
#28232=CARTESIAN_POINT('Ctrl Pts',(47.4779991713705,-4.0708466276555,-0.0138531808457906));
#28233=CARTESIAN_POINT('Ctrl Pts',(47.5184473448133,-4.06740414240983,-0.703330421609799));
#28234=CARTESIAN_POINT('Ctrl Pts',(47.5985318512543,-3.70631686362458,-2.06483195502968));
#28235=CARTESIAN_POINT('Ctrl Pts',(47.7174408502492,-2.2695351249873,-3.58462355241781));
#28236=CARTESIAN_POINT('Ctrl Pts',(47.8363498492442,-0.281252373079731,
-4.23334534366577));
#28237=CARTESIAN_POINT('Ctrl Pts',(47.9552588482392,1.77537519844767,-3.85335679646156));
#28238=CARTESIAN_POINT('Ctrl Pts',(48.0741678472341,3.40058348498636,-2.53699579379582));
#28239=CARTESIAN_POINT('Ctrl Pts',(48.1930768462292,4.19944402434456,-0.604140366551068));
#28240=CARTESIAN_POINT('Ctrl Pts',(48.311985845224,3.97783230526572,1.47552222866482));
#28241=CARTESIAN_POINT('Ctrl Pts',(48.4308948442191,2.78960036391312,3.19663033611261));
#28242=CARTESIAN_POINT('Ctrl Pts',(48.549803843214,0.923490644693623,4.14095166903249));
#28243=CARTESIAN_POINT('Ctrl Pts',(48.6687128422089,-1.16702891982273,4.07901448837793));
#28244=CARTESIAN_POINT('Ctrl Pts',(48.787621841204,-2.97395841132729,3.02586963760755));
#28245=CARTESIAN_POINT('Ctrl Pts',(48.8904466707762,-3.91154991106107,1.4793451741346));
#28246=CARTESIAN_POINT('Ctrl Pts',(48.9536351673504,-4.07000722284897,0.401595655703711));
#28247=CARTESIAN_POINT('Ctrl Pts',(48.9771873309261,-4.07020325257276,-5.60749305029626E-5));
#28248=CARTESIAN_POINT('Ctrl Pts',(47.7728126690739,-4.07022605737327,-6.6507676197633E-5));
#28249=CARTESIAN_POINT('Ctrl Pts',(47.7880884594498,-4.07037794775498,-0.260571206839678));
#28250=CARTESIAN_POINT('Ctrl Pts',(47.843000582824,-3.98185834718379,-1.19690962418239));
#28251=CARTESIAN_POINT('Ctrl Pts',(47.9375490391964,-3.27202394254474,-2.70077306086147));
#28252=CARTESIAN_POINT('Ctrl Pts',(48.0564580381915,-1.58419215321593,-3.93581643735453));
#28253=CARTESIAN_POINT('Ctrl Pts',(48.1753670371864,0.48860110601671,-4.21444952111902));
#28254=CARTESIAN_POINT('Ctrl Pts',(48.2942760361814,2.44266344009801,-3.46896398442958));
#28255=CARTESIAN_POINT('Ctrl Pts',(48.4131850351763,3.80315427688869,-1.88051411934194));
#28256=CARTESIAN_POINT('Ctrl Pts',(48.5320940341713,4.23947195846584,0.164903972792664));
#28257=CARTESIAN_POINT('Ctrl Pts',(48.6510030331663,3.6455905234561,2.17025011050524));
#28258=CARTESIAN_POINT('Ctrl Pts',(48.7699120321612,2.16582420148474,3.64822166748742));
#28259=CARTESIAN_POINT('Ctrl Pts',(48.8888210311562,0.159758802432322,4.23966896489628));
#28260=CARTESIAN_POINT('Ctrl Pts',(49.0077300301511,-1.88512826562663,3.80086927281119));
#28261=CARTESIAN_POINT('Ctrl Pts',(49.1266390291461,-3.47192586100346,2.43845168550668));
#28262=CARTESIAN_POINT('Ctrl Pts',(49.214999908787,-4.02413103778621,0.985723268098756));
#28263=CARTESIAN_POINT('Ctrl Pts',(49.2637244554296,-4.07066214181886,0.155059660506298));
#28264=CARTESIAN_POINT('Ctrl Pts',(49.2728126690739,-4.07050358506006,0.000104730133326219));
#28265=CARTESIAN_POINT('Origin',(27.2271873309261,0.,0.));
#28266=CARTESIAN_POINT('',(45.9771873309261,-4.07025298643191,7.60445319761115E-5));
#28267=CARTESIAN_POINT('',(46.2728126690739,-4.07084821056548,-6.23604212610479E-8));
#28268=CARTESIAN_POINT('',(27.2271873309261,-4.0705,-3.42898509504556E-13));
#28269=CARTESIAN_POINT('Ctrl Pts',(45.9771873309261,-4.07025298643191,7.60445319760578E-5));
#28270=CARTESIAN_POINT('Ctrl Pts',(46.0023631753907,-4.06996423923268,-0.429250442864527));
#28271=CARTESIAN_POINT('Ctrl Pts',(46.0671753528536,-3.89585401982529,-1.53472846738843));
#28272=CARTESIAN_POINT('Ctrl Pts',(46.1716238633148,-2.91160450045647,-3.085915573865));
#28273=CARTESIAN_POINT('Ctrl Pts',(46.2905328623097,-1.08356448049494,-4.10197558655686));
#28274=CARTESIAN_POINT('Ctrl Pts',(46.4094418613047,1.00778360743057,-4.12124834203113));
#28275=CARTESIAN_POINT('Ctrl Pts',(46.5283508602997,2.85423851237071,-3.13905052692677));
#28276=CARTESIAN_POINT('Ctrl Pts',(46.6472598592946,4.00710845607509,-1.39405793184905));
#28277=CARTESIAN_POINT('Ctrl Pts',(46.7661688582896,4.18624402154559,0.689693184085104));
#28278=CARTESIAN_POINT('Ctrl Pts',(46.8850778572845,3.34811495239536,2.60584764743572));
#28279=CARTESIAN_POINT('Ctrl Pts',(47.0039868562795,1.6963880814478,3.88877656509363));
#28280=CARTESIAN_POINT('Ctrl Pts',(47.1228958552745,-0.367564066613851,
4.22672596143089));
#28281=CARTESIAN_POINT('Ctrl Pts',(47.2418048542694,-2.34219750224519,3.5375735408011));
#28282=CARTESIAN_POINT('Ctrl Pts',(47.3599020128199,-3.73807708372676,1.99935876618999));
#28283=CARTESIAN_POINT('Ctrl Pts',(47.4383628383722,-4.07070915312478,0.661786852459511));
#28284=CARTESIAN_POINT('Ctrl Pts',(47.4771873309261,-4.0708438118707,-1.4567043702333E-5));
#28285=CARTESIAN_POINT('Ctrl Pts',(46.2728126690739,-4.07084821052679,-6.2360414317037E-8));
#28286=CARTESIAN_POINT('Ctrl Pts',(46.2728161304716,-4.07084821058119,-5.90650821111205E-5));
#28287=CARTESIAN_POINT('Ctrl Pts',(46.3124559248676,-4.07083382666307,-0.675755980011897));
#28288=CARTESIAN_POINT('Ctrl Pts',(46.391732052262,-3.72710065291479,-2.02707585696816));
#28289=CARTESIAN_POINT('Ctrl Pts',(46.5106410512569,-2.30583141340579,-3.56138418312489));
#28290=CARTESIAN_POINT('Ctrl Pts',(46.6295500502519,-0.324241098922964,
-4.23026991061211));
#28291=CARTESIAN_POINT('Ctrl Pts',(46.7484590492469,1.73614037090757,-3.87119263526966));
#28292=CARTESIAN_POINT('Ctrl Pts',(46.8673680482418,3.37463668760993,-2.57140876437375));
#28293=CARTESIAN_POINT('Ctrl Pts',(46.9862770472368,4.1930903743722,-0.646768056731501));
#28294=CARTESIAN_POINT('Ctrl Pts',(47.1051860462317,3.99261575077701,1.43503842231084));
#28295=CARTESIAN_POINT('Ctrl Pts',(47.2240950452267,2.82192850173731,3.16812804948658));
#28296=CARTESIAN_POINT('Ctrl Pts',(47.3430040442217,0.965507680676692,4.13135700774157));
#28297=CARTESIAN_POINT('Ctrl Pts',(47.4619130432167,-1.12553319906949,4.0906589719327));
#28298=CARTESIAN_POINT('Ctrl Pts',(47.5808220422116,-2.943067538678,3.05592363609448));
#28299=CARTESIAN_POINT('Ctrl Pts',(47.6844552508307,-3.9038147944966,1.50692039589771));
#28300=CARTESIAN_POINT('Ctrl Pts',(47.7484521264515,-4.06998383539806,0.415364423959208));
#28301=CARTESIAN_POINT('Ctrl Pts',(47.7728126690739,-4.07022605737327,-6.6507676197633E-5));
#28302=CARTESIAN_POINT('Origin',(27.2271873309261,0.,0.));
#28303=CARTESIAN_POINT('',(44.4771873309261,-4.07046018544014,-0.000104814225191196));
#28304=CARTESIAN_POINT('',(44.7728126690739,-4.07022626980563,6.65930553608862E-5));
#28305=CARTESIAN_POINT('',(27.2271873309261,-4.0705,-3.42898509504556E-13));
#28306=CARTESIAN_POINT('Ctrl Pts',(44.4771873309261,-4.07046018544014,-0.000104814225191444));
#28307=CARTESIAN_POINT('Ctrl Pts',(44.4870908464125,-4.07062964953048,-0.168965898301323));
#28308=CARTESIAN_POINT('Ctrl Pts',(44.5366306948972,-4.01905312111591,-1.01354822912588));
#28309=CARTESIAN_POINT('Ctrl Pts',(44.6258068763802,-3.44676119221666,-2.47389429282434));
#28310=CARTESIAN_POINT('Ctrl Pts',(44.7447158753752,-1.84608863354493,-3.819983306226));
#28311=CARTESIAN_POINT('Ctrl Pts',(44.8636248743702,0.203186698440704,-4.23780967691975));
#28312=CARTESIAN_POINT('Ctrl Pts',(44.9825338733652,2.20308730674562,-3.62584087029532));
#28313=CARTESIAN_POINT('Ctrl Pts',(45.1014428723601,3.66763383799168,-2.13278637607099));
#28314=CARTESIAN_POINT('Ctrl Pts',(45.2203518713551,4.24093891825145,-0.12146105473511));
#28315=CARTESIAN_POINT('Ctrl Pts',(45.33926087035,3.78368840810334,1.91937951603509));
#28316=CARTESIAN_POINT('Ctrl Pts',(45.458169869345,2.40699498298607,3.49380750011858));
#28317=CARTESIAN_POINT('Ctrl Pts',(45.5770788683399,0.445397558168305,4.21923413800868));
#28318=CARTESIAN_POINT('Ctrl Pts',(45.6959878673349,-1.62443225394642,3.91937948512372));
#28319=CARTESIAN_POINT('Ctrl Pts',(45.8148968663298,-3.29952218115088,2.66710874772735));
#28320=CARTESIAN_POINT('Ctrl Pts',(45.9086300208603,-3.98792413853412,1.16908185563358));
#28321=CARTESIAN_POINT('Ctrl Pts',(45.9627268423924,-4.07041883689898,0.246672370505476));
#28322=CARTESIAN_POINT('Ctrl Pts',(45.9771873309261,-4.07025298643191,7.60445319760578E-5));
#28323=CARTESIAN_POINT('Ctrl Pts',(44.7728126690739,-4.07022626980563,6.65930553610944E-5));
#28324=CARTESIAN_POINT('Ctrl Pts',(44.7971801344918,-4.0699836514846,-0.415482333917985));
#28325=CARTESIAN_POINT('Ctrl Pts',(44.861183932908,-3.90374787388921,-1.50715653101103));
#28326=CARTESIAN_POINT('Ctrl Pts',(44.9648240643225,-2.94280167925739,-3.05617965494951));
#28327=CARTESIAN_POINT('Ctrl Pts',(45.0837330633174,-1.12517733033491,-4.09075687156072));
#28328=CARTESIAN_POINT('Ctrl Pts',(45.2026420623124,0.965867082001261,-4.13127299833094));
#28329=CARTESIAN_POINT('Ctrl Pts',(45.3215510613073,2.82220410049894,-3.16788254548659));
#28330=CARTESIAN_POINT('Ctrl Pts',(45.4404600603023,3.99274057599417,-1.43469108161613));
#28331=CARTESIAN_POINT('Ctrl Pts',(45.5593690592973,4.193034093298,0.647132829719501));
#28332=CARTESIAN_POINT('Ctrl Pts',(45.6782780582922,3.37441297664422,2.57170232918147));
#28333=CARTESIAN_POINT('Ctrl Pts',(45.7971870572872,1.73580359220705,3.87134365513335));
#28334=CARTESIAN_POINT('Ctrl Pts',(45.9160960562822,-0.324609107543747,
4.23024168744071));
#28335=CARTESIAN_POINT('Ctrl Pts',(46.0350050552771,-2.306141225207,3.56118357519822));
#28336=CARTESIAN_POINT('Ctrl Pts',(46.1539105928744,-3.72723561434065,2.02679627912053));
#28337=CARTESIAN_POINT('Ctrl Pts',(46.2331797974733,-4.07084758770274,0.675578847152629));
#28338=CARTESIAN_POINT('Ctrl Pts',(46.2728126690739,-4.07084821052679,-6.2360414317037E-8));
#28339=CARTESIAN_POINT('Origin',(27.2271873309261,0.,0.));
#28340=CARTESIAN_POINT('',(42.9771873309261,-4.07069838669775,9.14325826918604E-5));
#28341=CARTESIAN_POINT('',(43.2728126690739,-4.07050321383809,-0.0001047408713159));
#28342=CARTESIAN_POINT('',(27.2271873309261,-4.0705,-3.42898509504556E-13));
#28343=CARTESIAN_POINT('Ctrl Pts',(42.9771873309261,-4.07069838669775,9.14325826918867E-5));
#28344=CARTESIAN_POINT('Ctrl Pts',(43.0114548504327,-4.07016735320138,-0.584091151150294));
#28345=CARTESIAN_POINT('Ctrl Pts',(43.0853587029375,-3.79600152359016,-1.84449226855255));
#28346=CARTESIAN_POINT('Ctrl Pts',(43.1988988884408,-2.54082596366002,-3.39771592193865));
#28347=CARTESIAN_POINT('Ctrl Pts',(43.3178078874356,-0.608870803793044,
-4.19876433520088));
#28348=CARTESIAN_POINT('Ctrl Pts',(43.4367168864306,1.47103965821834,-3.97949031283073));
#28349=CARTESIAN_POINT('Ctrl Pts',(43.5556258854256,3.19348559196464,-2.79320086151097));
#28350=CARTESIAN_POINT('Ctrl Pts',(43.6745348844206,4.13990858508463,-0.928154848713153));
#28351=CARTESIAN_POINT('Ctrl Pts',(43.7934438834155,4.08032670854032,1.16243248575246));
#28352=CARTESIAN_POINT('Ctrl Pts',(43.9123528824105,3.0292182035071,2.97054765803357));
#28353=CARTESIAN_POINT('Ctrl Pts',(44.0312618814054,1.2420044090019,4.05681405687331));
#28354=CARTESIAN_POINT('Ctrl Pts',(44.1501708804004,-0.847018655558019,
4.15726777299333));
#28355=CARTESIAN_POINT('Ctrl Pts',(44.2690798793954,-2.73021469130703,3.24749801153628));
#28356=CARTESIAN_POINT('Ctrl Pts',(44.378085362904,-3.84837513323758,1.6900775035994));
#28357=CARTESIAN_POINT('Ctrl Pts',(44.4474545134142,-4.06995141207779,0.506858173271681));
#28358=CARTESIAN_POINT('Ctrl Pts',(44.4771873309261,-4.07046018544014,-0.000104814225191444));
#28359=CARTESIAN_POINT('Ctrl Pts',(43.2728126690739,-4.07050321383809,-0.000104740871315935));
#28360=CARTESIAN_POINT('Ctrl Pts',(43.2819078055136,-4.0706618730839,-0.155177721611787));
#28361=CARTESIAN_POINT('Ctrl Pts',(43.3306392749516,-4.0240885331959,-0.985959389093055));
#28362=CARTESIAN_POINT('Ctrl Pts',(43.419007077388,-3.47171372465588,-2.43875382803693));
#28363=CARTESIAN_POINT('Ctrl Pts',(43.5379160763829,-1.88479759986051,-3.80103319712063));
#28364=CARTESIAN_POINT('Ctrl Pts',(43.6568250753779,0.160127627215037,-4.23965507926387));
#28365=CARTESIAN_POINT('Ctrl Pts',(43.7757340743728,2.16614156925702,-3.64803322477728));
#28366=CARTESIAN_POINT('Ctrl Pts',(43.8946430733678,3.64577930876166,-2.16993296345209));
#28367=CARTESIAN_POINT('Ctrl Pts',(44.0135520723628,4.23948628841551,-0.1645351582025));
#28368=CARTESIAN_POINT('Ctrl Pts',(44.1324610713577,3.80299066814145,1.88084496359989));
#28369=CARTESIAN_POINT('Ctrl Pts',(44.2513700703527,2.44236165043659,3.46917647027723));
#28370=CARTESIAN_POINT('Ctrl Pts',(44.3702790693477,0.488234470571936,4.21449201028578));
#28371=CARTESIAN_POINT('Ctrl Pts',(44.4891880683426,-1.58453454124508,3.93567860682148));
#28372=CARTESIAN_POINT('Ctrl Pts',(44.6080970673376,-3.27225888233889,2.70048840272595));
#28373=CARTESIAN_POINT('Ctrl Pts',(44.7026386009147,-3.98191049238861,1.19667333697073));
#28374=CARTESIAN_POINT('Ctrl Pts',(44.7575438014934,-4.07037829657382,0.260453195861538));
#28375=CARTESIAN_POINT('Ctrl Pts',(44.7728126690739,-4.07022626980563,6.65930553610944E-5));
#28376=CARTESIAN_POINT('Origin',(27.2271873309261,0.,0.));
#28377=CARTESIAN_POINT('',(41.4771873309261,-4.06894895743657,0.00540651071496451));
#28378=CARTESIAN_POINT('',(41.7728126690739,-4.07070027400187,-0.000480811481659155));
#28379=CARTESIAN_POINT('',(27.2271873309261,-4.0705,-3.42898509504556E-13));
#28380=CARTESIAN_POINT('Ctrl Pts',(41.4771873309261,-4.06894895743657,0.00540651071496485));
#28381=CARTESIAN_POINT('Ctrl Pts',(41.5358188544528,-4.05939870704616,-0.995808554814875));
#28382=CARTESIAN_POINT('Ctrl Pts',(41.6737230439761,-3.1827766265387,-3.36894097376134));
#28383=CARTESIAN_POINT('Ctrl Pts',(41.8512635664978,0.0468156998159277,
-4.48442240866564));
#28384=CARTESIAN_POINT('Ctrl Pts',(42.0098088984911,2.60148746873208,-3.34400839089152));
#28385=CARTESIAN_POINT('Ctrl Pts',(42.1287178974861,3.88717983168713,-1.70435364109129));
#28386=CARTESIAN_POINT('Ctrl Pts',(42.247626896481,4.22697668061874,0.364604063255797));
#28387=CARTESIAN_POINT('Ctrl Pts',(42.366535895476,3.54029074951913,2.33730671702443));
#28388=CARTESIAN_POINT('Ctrl Pts',(42.485444894471,1.99296498656723,3.7458830298263));
#28389=CARTESIAN_POINT('Ctrl Pts',(42.6043538934659,-0.0384826524084342,
4.24227598834855));
#28390=CARTESIAN_POINT('Ctrl Pts',(42.7232628924609,-2.06066523781936,3.70875467629474));
#28391=CARTESIAN_POINT('Ctrl Pts',(42.8421718914558,-3.58205929234741,2.27351505986046));
#28392=CARTESIAN_POINT('Ctrl Pts',(42.9268133709443,-4.04543031358348,0.858803213014503));
#28393=CARTESIAN_POINT('Ctrl Pts',(42.9718185174344,-4.07078158559399,0.0916173843402187));
#28394=CARTESIAN_POINT('Ctrl Pts',(42.9771873309261,-4.07069838669775,9.14325826918867E-5));
#28395=CARTESIAN_POINT('Ctrl Pts',(41.7728126690739,-4.07070027400187,-0.000480811481659068));
#28396=CARTESIAN_POINT('Ctrl Pts',(41.8062718095338,-4.07015469889988,-0.57096407947981));
#28397=CARTESIAN_POINT('Ctrl Pts',(41.8793672829919,-3.80565769019447,-1.81613961322352));
#28398=CARTESIAN_POINT('Ctrl Pts',(41.9920990894484,-2.5752427483792,-3.37219006842077));
#28399=CARTESIAN_POINT('Ctrl Pts',(42.1110080884434,-0.651474736920205,
-4.19213227664958));
#28400=CARTESIAN_POINT('Ctrl Pts',(42.2299170874383,1.43053091718906,-3.99434360254506));
#28401=CARTESIAN_POINT('Ctrl Pts',(42.3488260864333,3.16495106439444,-2.82543900138727));
#28402=CARTESIAN_POINT('Ctrl Pts',(42.4677350854282,4.13026450704979,-0.970190049367721));
#28403=CARTESIAN_POINT('Ctrl Pts',(42.5866440844232,4.09192548053664,1.12093820678962));
#28404=CARTESIAN_POINT('Ctrl Pts',(42.7055530834182,3.05923685698906,2.9396156616928));
#28405=CARTESIAN_POINT('Ctrl Pts',(42.8244620824131,1.28315058703404,4.04399185547656));
#28406=CARTESIAN_POINT('Ctrl Pts',(42.9433710814081,-0.804744663182227,
4.16565565627073));
#28407=CARTESIAN_POINT('Ctrl Pts',(43.0622800804031,-2.69708497911968,3.27506549112629));
#28408=CARTESIAN_POINT('Ctrl Pts',(43.1720939429583,-3.83941755468911,1.71761765906299));
#28409=CARTESIAN_POINT('Ctrl Pts',(43.2422714725153,-4.06997044082866,0.520625697547703));
#28410=CARTESIAN_POINT('Ctrl Pts',(43.2728126690739,-4.07050321383809,-0.000104740871315935));
#28411=CARTESIAN_POINT('Origin',(27.2271873309261,0.,0.));
#28412=CARTESIAN_POINT('',(39.9771873309261,-4.07077050609724,-5.79609919884648E-5));
#28413=CARTESIAN_POINT('',(40.2728126690739,-4.07025619321701,0.000377108328969283));
#28414=CARTESIAN_POINT('',(27.2271873309261,-4.0705,-3.42898509504556E-13));
#28415=CARTESIAN_POINT('Ctrl Pts',(39.9771873309261,-4.07077050609724,-5.79609919882859E-5));
#28416=CARTESIAN_POINT('Ctrl Pts',(39.9809101924763,-4.07081705151356,-0.0635213177095936));
#28417=CARTESIAN_POINT('Ctrl Pts',(40.0242693870248,-4.05388725332644,-0.802638439329735));
#28418=CARTESIAN_POINT('Ctrl Pts',(40.1072649145718,-3.62830971000893,-2.19902759642159));
#28419=CARTESIAN_POINT('Ctrl Pts',(40.2261739135667,-2.13693872948098,-3.66517562577142));
#28420=CARTESIAN_POINT('Ctrl Pts',(40.3450829125617,-0.126195570511627,
-4.24090522757565));
#28421=CARTESIAN_POINT('Ctrl Pts',(40.4639919115566,1.91502918549748,-3.78563729041068));
#28422=CARTESIAN_POINT('Ctrl Pts',(40.5829009105516,3.49126579952493,-2.41135070611703));
#28423=CARTESIAN_POINT('Ctrl Pts',(40.7018099095465,4.21838606955971,-0.449310859787289));
#28424=CARTESIAN_POINT('Ctrl Pts',(40.8207189085415,3.92189238888511,1.61834114804089));
#28425=CARTESIAN_POINT('Ctrl Pts',(40.9396279075364,2.66945837179664,3.2998455083566));
#28426=CARTESIAN_POINT('Ctrl Pts',(41.0585369065315,0.774140435187547,4.16543344142367));
#28427=CARTESIAN_POINT('Ctrl Pts',(41.2170822385247,-2.01888746148146,4.0045386084997));
#28428=CARTESIAN_POINT('Ctrl Pts',(41.3566323799896,-3.87071962072282,2.05940168604075));
#28429=CARTESIAN_POINT('Ctrl Pts',(41.4565461884562,-4.07231110917807,0.357882816421777));
#28430=CARTESIAN_POINT('Ctrl Pts',(41.4771873309261,-4.06894895743657,0.00540651071496485));
#28431=CARTESIAN_POINT('Ctrl Pts',(40.2728126690739,-4.07025619321701,0.000377108328969492));
#28432=CARTESIAN_POINT('Ctrl Pts',(40.2909994805556,-4.07036169565849,-0.309620800904844));
#28433=CARTESIAN_POINT('Ctrl Pts',(40.3488226250356,-3.95913913945033,-1.29545413833272));
#28434=CARTESIAN_POINT('Ctrl Pts',(40.4462821025139,-3.17025406296392,-2.82213573711675));
#28435=CARTESIAN_POINT('Ctrl Pts',(40.5651911015089,-1.44080558796838,-3.98425201455624));
#28436=CARTESIAN_POINT('Ctrl Pts',(40.7237364335021,1.3412377851549,-4.2793985106552));
#28437=CARTESIAN_POINT('Ctrl Pts',(40.9219180984939,4.38508550900277,-1.98115657932714));
#28438=CARTESIAN_POINT('Ctrl Pts',(41.1597360964836,4.03738561363306,2.61791400162535));
#28439=CARTESIAN_POINT('Ctrl Pts',(41.3579177614753,0.682606151108172,4.43240558295318));
#28440=CARTESIAN_POINT('Ctrl Pts',(41.5164630934686,-2.02344151873906,3.72234728068988));
#28441=CARTESIAN_POINT('Ctrl Pts',(41.6353720924636,-3.55851387613991,2.31342601692174));
#28442=CARTESIAN_POINT('Ctrl Pts',(41.7208219509987,-4.04108037252554,0.88609737447698));
#28443=CARTESIAN_POINT('Ctrl Pts',(41.7666354765354,-4.07080099752324,0.104841230207512));
#28444=CARTESIAN_POINT('Ctrl Pts',(41.7728126690739,-4.07070027400187,-0.000480811481659068));
#28445=CARTESIAN_POINT('Origin',(27.2271873309261,0.,0.));
#28446=CARTESIAN_POINT('',(38.4771873309261,-4.07037658145865,9.98552888675809E-5));
#28447=CARTESIAN_POINT('',(38.7728126690739,-4.07079742697958,-5.00540521497506E-5));
#28448=CARTESIAN_POINT('',(27.2271873309261,-4.0705,-3.42898509504556E-13));
#28449=CARTESIAN_POINT('Ctrl Pts',(38.4771873309261,-4.07037658145865,9.98552888676826E-5));
#28450=CARTESIAN_POINT('Ctrl Pts',(38.5052741964965,-4.06993440527969,-0.478826890908034));
#28451=CARTESIAN_POINT('Ctrl Pts',(38.5729973950651,-3.86611251597914,-1.63398402620179));
#28452=CARTESIAN_POINT('Ctrl Pts',(38.6803569266322,-2.79679599758437,-3.19033663920374));
#28453=CARTESIAN_POINT('Ctrl Pts',(38.7992659256271,-0.932818789330533,
-4.13886031436587));
#28454=CARTESIAN_POINT('Ctrl Pts',(38.9181749246222,1.15783504299492,-4.081633735705));
#28455=CARTESIAN_POINT('Ctrl Pts',(39.037083923617,2.96713288406074,-3.03256289173867));
#28456=CARTESIAN_POINT('Ctrl Pts',(39.1559929226121,4.05541232630964,-1.24657417618181));
#28457=CARTESIAN_POINT('Ctrl Pts',(39.274901921607,4.15821928046345,0.8423347006637));
#28458=CARTESIAN_POINT('Ctrl Pts',(39.393810920602,3.25057202966842,2.72655386816114));
#28459=CARTESIAN_POINT('Ctrl Pts',(39.5127199195969,1.55302934330574,3.94821746331971));
#28460=CARTESIAN_POINT('Ctrl Pts',(39.631628918592,-0.521900729557193,4.21045371123498));
#28461=CARTESIAN_POINT('Ctrl Pts',(39.7505379175868,-2.47001093446444,3.44954947520581));
#28462=CARTESIAN_POINT('Ctrl Pts',(39.8657240550316,-3.77569799789881,1.90045186147924));
#28463=CARTESIAN_POINT('Ctrl Pts',(39.941273859478,-4.0703214946426,0.612156438801636));
#28464=CARTESIAN_POINT('Ctrl Pts',(39.9771873309261,-4.07077050609724,-5.79609919882859E-5));
#28465=CARTESIAN_POINT('Ctrl Pts',(38.7728126690739,-4.07079742697958,-5.00540521495944E-5));
#28466=CARTESIAN_POINT('Ctrl Pts',(38.7757271515774,-4.07082806252421,-0.049731900772906));
#28467=CARTESIAN_POINT('Ctrl Pts',(38.8182779670792,-4.05782430804937,-0.77506006973181));
#28468=CARTESIAN_POINT('Ctrl Pts',(38.9004651155794,-3.65047142573015,-2.16202983439362));
#28469=CARTESIAN_POINT('Ctrl Pts',(39.0193741145744,-2.17403875473271,-3.64333320582671));
#28470=CARTESIAN_POINT('Ctrl Pts',(39.1382831135694,-0.169311715692027,
-4.23929647022592));
#28471=CARTESIAN_POINT('Ctrl Pts',(39.2571921125643,1.87656008277306,-3.80511074896768));
#28472=CARTESIAN_POINT('Ctrl Pts',(39.3761011115593,3.46642106848062,-2.4462615072031));
#28473=CARTESIAN_POINT('Ctrl Pts',(39.4950101105543,4.21394248995934,-0.49299624037214));
#28474=CARTESIAN_POINT('Ctrl Pts',(39.6139191095491,3.93745486993259,1.58012745604));
#28475=CARTESIAN_POINT('Ctrl Pts',(39.7328281085442,2.7041860128382,3.26915872948103));
#28476=CARTESIAN_POINT('Ctrl Pts',(39.8517371075391,0.813740946052253,4.1640155130528));
#28477=CARTESIAN_POINT('Ctrl Pts',(39.9706461065341,-1.27433631150534,4.04653670722897));
#28478=CARTESIAN_POINT('Ctrl Pts',(40.089555105529,-3.05296367944959,2.94668522964312));
#28479=CARTESIAN_POINT('Ctrl Pts',(40.1902772930423,-3.93078192295446,1.40692776914096));
#28480=CARTESIAN_POINT('Ctrl Pts',(40.2513631475573,-4.0701317636604,0.365988575238109));
#28481=CARTESIAN_POINT('Ctrl Pts',(40.2728126690739,-4.07025619321701,0.000377108328969492));
#28482=CARTESIAN_POINT('Origin',(27.2271873309261,0.,0.));
#28483=CARTESIAN_POINT('',(36.9771873309261,-4.07031820724409,-9.1677525538646E-5));
#28484=CARTESIAN_POINT('',(37.2728126690739,-4.07033856695489,9.50420139643471E-5));
#28485=CARTESIAN_POINT('',(27.2271873309261,-4.0705,-3.42898509504556E-13));
#28486=CARTESIAN_POINT('Ctrl Pts',(36.9771873309261,-4.07031820724409,-9.16775255385346E-5));
#28487=CARTESIAN_POINT('Ctrl Pts',(36.9900018675183,-4.07049942327998,-0.218609364111448));
#28488=CARTESIAN_POINT('Ctrl Pts',(37.0424527371088,-3.99970858733677,-1.112902578135));
#28489=CARTESIAN_POINT('Ctrl Pts',(37.1345399396977,-3.35397800645881,-2.59829698616001));
#28490=CARTESIAN_POINT('Ctrl Pts',(37.2534489386926,-1.70514605210925,-3.88494435443889));
#28491=CARTESIAN_POINT('Ctrl Pts',(37.3723579376876,0.358039381572612,-4.22754343529587));
#28492=CARTESIAN_POINT('Ctrl Pts',(37.4912669366826,2.3342206179893,-3.54284205161814));
#28493=CARTESIAN_POINT('Ctrl Pts',(37.6101759356776,3.74318215294784,-1.99722383969792));
#28494=CARTESIAN_POINT('Ctrl Pts',(37.7290849346725,4.24254386394922,0.0337232658201172));
#28495=CARTESIAN_POINT('Ctrl Pts',(37.8479939336675,3.71095997990038,2.05647555874971));
#28496=CARTESIAN_POINT('Ctrl Pts',(37.9669029326624,2.27760631649146,3.57950068621502));
#28497=CARTESIAN_POINT('Ctrl Pts',(38.0858119316574,0.290790325944755,4.23270087345946));
#28498=CARTESIAN_POINT('Ctrl Pts',(38.2047209306524,-1.76668822311588,3.85734732873792));
#28499=CARTESIAN_POINT('Ctrl Pts',(38.3236299296473,-3.39485843815668,2.54465162401958));
#28500=CARTESIAN_POINT('Ctrl Pts',(38.4144520630719,-4.00834925103214,1.06972433652504));
#28501=CARTESIAN_POINT('Ctrl Pts',(38.4656378634982,-4.07055840663824,0.197037062173665));
#28502=CARTESIAN_POINT('Ctrl Pts',(38.4771873309261,-4.07037658145865,9.98552888676826E-5));
#28503=CARTESIAN_POINT('Ctrl Pts',(37.2728126690739,-4.07033856695489,9.50420139643297E-5));
#28504=CARTESIAN_POINT('Ctrl Pts',(37.3000911555976,-4.06993567621103,-0.465060000392124));
#28505=CARTESIAN_POINT('Ctrl Pts',(37.3670059751196,-3.87457929834536,-1.60642688649147));
#28506=CARTESIAN_POINT('Ctrl Pts',(37.4735571276399,-2.82905983413317,-3.16176157564063));
#28507=CARTESIAN_POINT('Ctrl Pts',(37.5924661266349,-0.974814094226818,
-4.12917101732149));
#28508=CARTESIAN_POINT('Ctrl Pts',(37.7113751256298,1.11631317895359,-4.09318466350003));
#28509=CARTESIAN_POINT('Ctrl Pts',(37.8302841246248,2.93617439347552,-3.06254726405115));
#28510=CARTESIAN_POINT('Ctrl Pts',(37.9491931236197,4.04254008318163,-1.28770550784711));
#28511=CARTESIAN_POINT('Ctrl Pts',(38.0681021226147,4.16656144887969,0.800050936289306));
#28512=CARTESIAN_POINT('Ctrl Pts',(38.1870111216096,3.27810107619118,2.69339361556102));
#28513=CARTESIAN_POINT('Ctrl Pts',(38.3059201206047,1.593056403167,3.93223689564486));
#28514=CARTESIAN_POINT('Ctrl Pts',(38.4248291195996,-0.479103781660292,
4.21553977736235));
#28515=CARTESIAN_POINT('Ctrl Pts',(38.5437381185946,-2.43484088061553,3.47445898581872));
#28516=CARTESIAN_POINT('Ctrl Pts',(38.659732635086,-3.76547389787559,1.92793678161055));
#28517=CARTESIAN_POINT('Ctrl Pts',(38.7360908185791,-4.07041142572947,0.625930491508946));
#28518=CARTESIAN_POINT('Ctrl Pts',(38.7728126690739,-4.07079742697958,-5.00540521495944E-5));
#28519=CARTESIAN_POINT('Origin',(27.2271873309261,0.,0.));
#28520=CARTESIAN_POINT('',(35.4771873309261,-4.07081121953653,4.27420412099477E-5));
#28521=CARTESIAN_POINT('',(35.7728126690739,-4.07035481323816,-9.73195012207717E-5));
#28522=CARTESIAN_POINT('',(27.2271873309261,-4.0705,-3.42898509504556E-13));
#28523=CARTESIAN_POINT('Ctrl Pts',(35.4771873309261,-4.07081121953653,4.27420412098516E-5));
#28524=CARTESIAN_POINT('Ctrl Pts',(35.5143658715385,-4.07046879867817,-0.633716582260352));
#28525=CARTESIAN_POINT('Ctrl Pts',(35.5911807451492,-3.75962139193843,-1.94345586451205));
#28526=CARTESIAN_POINT('Ctrl Pts',(35.7076319517581,-2.41486119677437,-3.48837513699617));
#28527=CARTESIAN_POINT('Ctrl Pts',(35.8265409507531,-0.454903298757822,
-4.21821984785987));
#28528=CARTESIAN_POINT('Ctrl Pts',(35.9454499497481,1.61559689818276,-3.92302974226322));
#28529=CARTESIAN_POINT('Ctrl Pts',(36.064358948743,3.29350421714833,-2.6745365332569));
#28530=CARTESIAN_POINT('Ctrl Pts',(36.183267947738,4.17108423869985,-0.776126258909775));
#28531=CARTESIAN_POINT('Ctrl Pts',(36.3021769467329,4.03508347943329,1.31088405669769));
#28532=CARTESIAN_POINT('Ctrl Pts',(36.4210859457279,2.91855036222394,3.07934724889256));
#28533=CARTESIAN_POINT('Ctrl Pts',(36.5399949447229,1.09280439154274,4.09952366232033));
#28534=CARTESIAN_POINT('Ctrl Pts',(36.6589039437179,-0.998494961682174,
4.12350864041721));
#28535=CARTESIAN_POINT('Ctrl Pts',(36.7778129427128,-2.84715828911907,3.14547379146596));
#28536=CARTESIAN_POINT('Ctrl Pts',(36.8839074051156,-3.87929173201797,1.59085652731975));
#28537=CARTESIAN_POINT('Ctrl Pts',(36.95036553452,-4.06993890834513,0.457282403743256));
#28538=CARTESIAN_POINT('Ctrl Pts',(36.9771873309261,-4.07031820724409,-9.16775255385346E-5));
#28539=CARTESIAN_POINT('Ctrl Pts',(35.7728126690739,-4.07035481323816,-9.73195012204595E-5));
#28540=CARTESIAN_POINT('Ctrl Pts',(35.7848188266194,-4.07053749389208,-0.204824981186366));
#28541=CARTESIAN_POINT('Ctrl Pts',(35.8364613171632,-4.0052715983505,-1.0853115636913));
#28542=CARTESIAN_POINT('Ctrl Pts',(35.9277401407054,-3.38019902696682,-2.56409249929749));
#28543=CARTESIAN_POINT('Ctrl Pts',(36.0466491397003,-1.74452218259612,-3.86742267683414));
#28544=CARTESIAN_POINT('Ctrl Pts',(36.1655581386953,0.315076609834192,-4.23096236532504));
#28545=CARTESIAN_POINT('Ctrl Pts',(36.2844671376903,2.29811123382828,-3.56637078327709));
#28546=CARTESIAN_POINT('Ctrl Pts',(36.4033761366852,3.72270080001742,-2.03514484998292));
#28547=CARTESIAN_POINT('Ctrl Pts',(36.5222851356802,4.24266754688635,-0.0093751510681078));
#28548=CARTESIAN_POINT('Ctrl Pts',(36.6411941346751,3.73165864358157,2.01867272598657));
#28549=CARTESIAN_POINT('Ctrl Pts',(36.7601031336701,2.31385014926909,3.55617959242768));
#28550=CARTESIAN_POINT('Ctrl Pts',(36.8790121326651,0.333772013114966,4.22952858485353));
#28551=CARTESIAN_POINT('Ctrl Pts',(36.99792113166,-1.72741330724408,3.87509471792328));
#28552=CARTESIAN_POINT('Ctrl Pts',(37.116830130655,-3.36883416623464,2.57900604248567));
#28553=CARTESIAN_POINT('Ctrl Pts',(37.2084606431263,-4.00286951946101,1.097315110437));
#28554=CARTESIAN_POINT('Ctrl Pts',(37.2604548225993,-4.07052108668355,0.210822077620177));
#28555=CARTESIAN_POINT('Ctrl Pts',(37.2728126690739,-4.07033856695489,9.50420139643297E-5));
#28556=CARTESIAN_POINT('Origin',(27.2271873309261,0.,0.));
#28557=CARTESIAN_POINT('',(33.9771873309261,-4.07016987886937,3.24954791396568E-5));
#28558=CARTESIAN_POINT('',(34.2728126690739,-4.07078562779549,5.5347657024335E-5));
#28559=CARTESIAN_POINT('',(27.2271873309261,-4.0705,-3.42898509504556E-13));
#28560=CARTESIAN_POINT('Ctrl Pts',(33.9771873309261,-4.07016987886936,3.24954791397145E-5));
#28561=CARTESIAN_POINT('Ctrl Pts',(33.9990935425603,-4.07006529445769,-0.373558417633581));
#28562=CARTESIAN_POINT('Ctrl Pts',(34.0606360871928,-3.92681616665385,-1.42319026575441));
#28563=CARTESIAN_POINT('Ctrl Pts',(34.1618149648236,-3.03590382713174,-2.96371450185516));
#28564=CARTESIAN_POINT('Ctrl Pts',(34.2807239638186,-1.25114215390858,-4.05400530424081));
#28565=CARTESIAN_POINT('Ctrl Pts',(34.3996329628135,0.837649255637629,-4.15916571209051));
#28566=CARTESIAN_POINT('Ctrl Pts',(34.5185419618086,2.72289042788497,-3.25364156197822));
#28567=CARTESIAN_POINT('Ctrl Pts',(34.6374509608034,3.94646445364522,-1.55747680952698));
#28568=CARTESIAN_POINT('Ctrl Pts',(34.7563599597985,4.21104070005508,0.517157537486679));
#28569=CARTESIAN_POINT('Ctrl Pts',(34.8752689587934,3.45232667550434,2.46612169644987));
#28570=CARTESIAN_POINT('Ctrl Pts',(34.9941779577884,1.85469121778504,3.8158139607128));
#28571=CARTESIAN_POINT('Ctrl Pts',(35.1130869567833,-0.193637456642115,
4.23825674440386));
#28572=CARTESIAN_POINT('Ctrl Pts',(35.2319959557783,-2.19491188970968,3.63079571065499));
#28573=CARTESIAN_POINT('Ctrl Pts',(35.3509049547733,-3.66281888647431,2.14104495538666));
#28574=CARTESIAN_POINT('Ctrl Pts',(35.4326354131559,-4.05998619783484,0.759479670105897));
#28575=CARTESIAN_POINT('Ctrl Pts',(35.4747295385402,-4.07083385623406,0.041939191340904));
#28576=CARTESIAN_POINT('Ctrl Pts',(35.4771873309261,-4.07081121953653,4.27420412098516E-5));
#28577=CARTESIAN_POINT('Ctrl Pts',(34.2728126690739,-4.07078562779549,5.5347657024309E-5));
#28578=CARTESIAN_POINT('Ctrl Pts',(34.3091828306396,-4.07036990121448,-0.619935370476085));
#28579=CARTESIAN_POINT('Ctrl Pts',(34.3851893252035,-3.76994385597486,-1.91598331854555));
#28580=CARTESIAN_POINT('Ctrl Pts',(34.5008321527658,-2.45017227519968,-3.46366447981092));
#28581=CARTESIAN_POINT('Ctrl Pts',(34.6197411517608,-0.497729417387068,
-4.21338121156021));
#28582=CARTESIAN_POINT('Ctrl Pts',(34.7386501507558,1.57566256123941,-3.93923892395085));
#28583=CARTESIAN_POINT('Ctrl Pts',(34.8575591497507,3.26616577576251,-2.70785467337129));
#28584=CARTESIAN_POINT('Ctrl Pts',(34.9764681487457,4.16298498204543,-0.818456991005179));
#28585=CARTESIAN_POINT('Ctrl Pts',(35.0953771477406,4.04819154107314,1.26982717471511));
#28586=CARTESIAN_POINT('Ctrl Pts',(35.2142861467356,2.94968046020461,3.04954111130644));
#28587=CARTESIAN_POINT('Ctrl Pts',(35.3331951457306,1.13439185749204,4.0882112128065));
#28588=CARTESIAN_POINT('Ctrl Pts',(35.4521041447256,-0.956555954881787,
4.13343882403517));
#28589=CARTESIAN_POINT('Ctrl Pts',(35.5710131437205,-2.81505899362824,3.17423355619177));
#28590=CARTESIAN_POINT('Ctrl Pts',(35.67791598517,-3.87091551080481,1.61841633854707));
#28591=CARTESIAN_POINT('Ctrl Pts',(35.7451824936211,-4.06993440408556,0.47104935594091));
#28592=CARTESIAN_POINT('Ctrl Pts',(35.7728126690739,-4.07035481323816,-9.73195012204595E-5));
#28593=CARTESIAN_POINT('Origin',(27.2271873309261,0.,0.));
#28594=CARTESIAN_POINT('',(32.4771873309261,-4.07063452722895,-9.39916808427117E-5));
#28595=CARTESIAN_POINT('',(32.7728126690739,-4.07016025367539,2.0115106517532E-5));
#28596=CARTESIAN_POINT('',(27.2271873309261,-4.0705,-3.42898509504556E-13));
#28597=CARTESIAN_POINT('Ctrl Pts',(32.4771873309261,-4.07063452722895,-9.399168084262E-5));
#28598=CARTESIAN_POINT('Ctrl Pts',(32.4838212135822,-4.07074636705293,-0.113191851009958));
#28599=CARTESIAN_POINT('Ctrl Pts',(32.5300914292365,-4.03852757013727,-0.901966866821061));
#28600=CARTESIAN_POINT('Ctrl Pts',(32.6159979778891,-3.54546956353323,-2.33022772913439));
#28601=CARTESIAN_POINT('Ctrl Pts',(32.7349069768841,-2.00143968510732,-3.74092968169653));
#28602=CARTESIAN_POINT('Ctrl Pts',(32.8538159758791,0.0289435448015357,
-4.24257916450323));
#28603=CARTESIAN_POINT('Ctrl Pts',(32.972724974874,2.05229344259103,-3.71327447432861));
#28604=CARTESIAN_POINT('Ctrl Pts',(33.091633973869,3.57693243670117,-2.28163757843869));
#28605=CARTESIAN_POINT('Ctrl Pts',(33.2105429728639,4.23237057927023,-0.295558751907219));
#28606=CARTESIAN_POINT('Ctrl Pts',(33.3294519718589,3.85933525284402,1.76234136938946));
#28607=CARTESIAN_POINT('Ctrl Pts',(33.4483609708539,2.54847469557654,3.39198944899592));
#28608=CARTESIAN_POINT('Ctrl Pts',(33.5672699698489,0.618330320477916,4.19737814723441));
#28609=CARTESIAN_POINT('Ctrl Pts',(33.6861789688438,-1.46206940626736,3.98279659879273));
#28610=CARTESIAN_POINT('Ctrl Pts',(33.8050879678388,-3.18718370466638,2.80038849605003));
#28611=CARTESIAN_POINT('Ctrl Pts',(33.9020907551995,-3.96267663186491,1.280678352677));
#28612=CARTESIAN_POINT('Ctrl Pts',(33.959457209562,-4.07025452583356,0.302403911433452));
#28613=CARTESIAN_POINT('Ctrl Pts',(33.9771873309261,-4.07016987886936,3.24954791397145E-5));
#28614=CARTESIAN_POINT('Ctrl Pts',(32.7728126690739,-4.07016025367539,2.01151065172891E-5));
#28615=CARTESIAN_POINT('Ctrl Pts',(32.7939105016614,-4.07009808342627,-0.359787052605734));
#28616=CARTESIAN_POINT('Ctrl Pts',(32.8546446672472,-3.93407800546665,-1.3956072406382));
#28617=CARTESIAN_POINT('Ctrl Pts',(32.9550151658314,-3.06585324807998,-2.93272222825354));
#28618=CARTESIAN_POINT('Ctrl Pts',(33.0739241648263,-1.29225906543464,-4.04108677395906));
#28619=CARTESIAN_POINT('Ctrl Pts',(33.1928331638213,0.795356335102055,-4.16746015062799));
#28620=CARTESIAN_POINT('Ctrl Pts',(33.3117421628162,2.68969875215823,-3.2811334062333));
#28621=CARTESIAN_POINT('Ctrl Pts',(33.4306511618112,3.93043965810529,-1.59748549315922));
#28622=CARTESIAN_POINT('Ctrl Pts',(33.5495601608062,4.21607683810534,0.47435419472437));
#28623=CARTESIAN_POINT('Ctrl Pts',(33.6684691598011,3.47719995677159,2.43092498187187));
#28624=CARTESIAN_POINT('Ctrl Pts',(33.7873781587961,1.89335739132502,3.79677673765208));
#28625=CARTESIAN_POINT('Ctrl Pts',(33.906287157791,-0.15057433877126,4.24000509143145));
#28626=CARTESIAN_POINT('Ctrl Pts',(34.025196156786,-2.1579162406289,3.65290477637881));
#28627=CARTESIAN_POINT('Ctrl Pts',(34.144105155781,-3.64088071375389,2.17814219808442));
#28628=CARTESIAN_POINT('Ctrl Pts',(34.2266439932103,-4.05612867944369,0.787058536401716));
#28629=CARTESIAN_POINT('Ctrl Pts',(34.2695464976412,-4.07082296153899,0.0557327459666281));
#28630=CARTESIAN_POINT('Ctrl Pts',(34.2728126690739,-4.07078562779549,5.5347657024309E-5));
#28631=CARTESIAN_POINT('Origin',(27.2271873309261,0.,0.));
#28632=CARTESIAN_POINT('',(30.9771873309261,-4.07052775430868,0.00010449998854035));
#28633=CARTESIAN_POINT('',(31.2728126690739,-4.07067546468071,-8.7070929181976E-5));
#28634=CARTESIAN_POINT('',(27.2271873309261,-4.0705,-3.42898509504556E-13));
#28635=CARTESIAN_POINT('Ctrl Pts',(30.9771873309261,-4.07052775430868,0.000104499988540334));
#28636=CARTESIAN_POINT('Ctrl Pts',(31.0081852176023,-4.06998453340041,-0.528403485036771));
#28637=CARTESIAN_POINT('Ctrl Pts',(31.0788194372768,-3.83428484306565,-1.73317487116484));
#28638=CARTESIAN_POINT('Ctrl Pts',(31.1890899899496,-2.67824532838493,-3.29048852198293));
#28639=CARTESIAN_POINT('Ctrl Pts',(31.3079989889446,-0.780824962758849,
-4.1702074196749));
#28640=CARTESIAN_POINT('Ctrl Pts',(31.4269079879395,1.30633725444068,-4.03655766520605));
#28641=CARTESIAN_POINT('Ctrl Pts',(31.5458169869345,3.07605722060134,-2.92201779428377));
#28642=CARTESIAN_POINT('Ctrl Pts',(31.6647259859295,4.09828989491981,-1.09742224157957));
#28643=CARTESIAN_POINT('Ctrl Pts',(31.7836349849244,4.12463093940056,0.993848720882264));
#28644=CARTESIAN_POINT('Ctrl Pts',(31.9025439839194,3.14867943729,2.84361276159299));
#28645=CARTESIAN_POINT('Ctrl Pts',(32.0214529829143,1.40759331257097,4.00237388736178));
#28646=CARTESIAN_POINT('Ctrl Pts',(32.1403619819093,-0.675540453973202,
4.18855115831721));
#28647=CARTESIAN_POINT('Ctrl Pts',(32.2592709809043,-2.59451670629275,3.35690314889015));
#28648=CARTESIAN_POINT('Ctrl Pts',(32.3715460972432,-3.81113575126776,1.80142850182054));
#28649=CARTESIAN_POINT('Ctrl Pts',(32.4441848805838,-4.07007814291696,0.562548834528985));
#28650=CARTESIAN_POINT('Ctrl Pts',(32.4771873309261,-4.07063452722895,-9.399168084262E-5));
#28651=CARTESIAN_POINT('Ctrl Pts',(31.2728126690739,-4.07067546468071,-8.70709291818372E-5));
#28652=CARTESIAN_POINT('Ctrl Pts',(31.2786381726832,-4.07076914227082,-0.0994003818986817));
#28653=CARTESIAN_POINT('Ctrl Pts',(31.3241000092909,-4.04297868156283,-0.874382434154477));
#28654=CARTESIAN_POINT('Ctrl Pts',(31.4091981788968,-3.56895760027616,-2.29409186709539));
#28655=CARTESIAN_POINT('Ctrl Pts',(31.5281071778918,-2.03933759614693,-3.72040561602178));
#28656=CARTESIAN_POINT('Ctrl Pts',(31.6470161768868,-0.0141549844227289,
-4.24265429393642));
#28657=CARTESIAN_POINT('Ctrl Pts',(31.7659251758817,2.01446731467499,-3.73393053486277));
#28658=CARTESIAN_POINT('Ctrl Pts',(31.8848341748767,3.55357052479912,-2.31785511487955));
#28659=CARTESIAN_POINT('Ctrl Pts',(32.0037431738717,4.229149869261,-0.338536837555411));
#28660=CARTESIAN_POINT('Ctrl Pts',(32.1226521728666,3.87703838273484,1.72304648374135));
#28661=CARTESIAN_POINT('Ctrl Pts',(32.2415611718616,2.58279977386025,3.36592648990226));
#28662=CARTESIAN_POINT('Ctrl Pts',(32.3604701708566,0.660936292926016,4.19088045920181));
#28663=CARTESIAN_POINT('Ctrl Pts',(32.4793791698515,-1.42153586561542,3.99744313151944));
#28664=CARTESIAN_POINT('Ctrl Pts',(32.5982881688465,-3.15857231724438,2.83262011635301));
#28665=CARTESIAN_POINT('Ctrl Pts',(32.6960993352539,-3.95605371558114,1.30826770260012));
#28666=CARTESIAN_POINT('Ctrl Pts',(32.7542741686631,-4.07021488218683,0.316179857998792));
#28667=CARTESIAN_POINT('Ctrl Pts',(32.7728126690739,-4.07016025367539,2.01151065172891E-5));
#28668=CARTESIAN_POINT('Origin',(52.575,4.52129938221115E-16,0.));
#28669=CARTESIAN_POINT('',(52.575,0.695807839646318,4.87560011181052));
#28670=CARTESIAN_POINT('Ctrl Pts',(52.575,3.27123862564629,-2.42269060785926));
#28671=CARTESIAN_POINT('Ctrl Pts',(52.575,3.33974877356658,-2.34761008169236));
#28672=CARTESIAN_POINT('Ctrl Pts',(52.575,3.40533191462526,-2.27003568459554));
#28673=CARTESIAN_POINT('Ctrl Pts',(52.575,3.46783701755502,-2.1901289314666));
#28674=CARTESIAN_POINT('Ctrl Pts',(52.575,3.54519071433771,-2.09123968142613));
#28675=CARTESIAN_POINT('Ctrl Pts',(52.575,3.61783176379727,-1.98877942727981));
#28676=CARTESIAN_POINT('Ctrl Pts',(52.575,3.68567005490555,-1.88315349412949));
#28677=CARTESIAN_POINT('Ctrl Pts',(52.575,3.72452565888664,-1.82265433706683));
#28678=CARTESIAN_POINT('Ctrl Pts',(52.575,3.76180508901478,-1.76111582740147));
#28679=CARTESIAN_POINT('Ctrl Pts',(52.575,3.79748635683124,-1.69860843369842));
#28680=CARTESIAN_POINT('Ctrl Pts',(52.575,3.81574454298833,-1.66662325771487));
#28681=CARTESIAN_POINT('Ctrl Pts',(52.575,3.83358420466306,-1.63438432888875));
#28682=CARTESIAN_POINT('Ctrl Pts',(52.575,3.85100198255905,-1.60190073374641));
#28683=CARTESIAN_POINT('Ctrl Pts',(52.575,3.86219017839908,-1.58103510862413));
#28684=CARTESIAN_POINT('Ctrl Pts',(52.575,3.87320429706676,-1.5600685282487));
#28685=CARTESIAN_POINT('Ctrl Pts',(52.575,3.88404338396807,-1.53900335395738));
#28686=CARTESIAN_POINT('Ctrl Pts',(52.575,3.89350384310779,-1.52061746753831));
#28687=CARTESIAN_POINT('Ctrl Pts',(52.575,3.90282655955187,-1.50216502101326));
#28688=CARTESIAN_POINT('Ctrl Pts',(52.575,3.91201088413724,-1.48364851325173));
#28689=CARTESIAN_POINT('Ctrl Pts',(52.575,3.96947384655046,-1.36779749125935));
#28690=CARTESIAN_POINT('Ctrl Pts',(52.575,4.02152670830412,-1.24943340089431));
#28691=CARTESIAN_POINT('Ctrl Pts',(52.575,4.06807408099195,-1.12898158468846));
#28692=CARTESIAN_POINT('Ctrl Pts',(52.575,4.11491086544974,-1.00778085030938));
#28693=CARTESIAN_POINT('Ctrl Pts',(52.575,4.15617394543224,-0.884465663289738));
#28694=CARTESIAN_POINT('Ctrl Pts',(52.575,4.1917261494215,-0.759434877005129));
#28695=CARTESIAN_POINT('Ctrl Pts',(52.575,4.20419944906554,-0.715568497791931));
#28696=CARTESIAN_POINT('Ctrl Pts',(52.575,4.21596939517056,-0.671490682417999));
#28697=CARTESIAN_POINT('Ctrl Pts',(52.575,4.22702874369151,-0.627217904445778));
#28698=CARTESIAN_POINT('Ctrl Pts',(52.575,4.23745334703906,-0.585486138005798));
#28699=CARTESIAN_POINT('Ctrl Pts',(52.575,4.24724657653273,-0.543581140564887));
#28700=CARTESIAN_POINT('Ctrl Pts',(52.575,4.25640176372427,-0.501516465484337));
#28701=CARTESIAN_POINT('Ctrl Pts',(52.575,4.26067115082541,-0.481900221988142));
#28702=CARTESIAN_POINT('Ctrl Pts',(52.575,4.26479980625067,-0.462258226011452));
#28703=CARTESIAN_POINT('Ctrl Pts',(52.575,4.26878680612531,-0.442595043227594));
#28704=CARTESIAN_POINT('Ctrl Pts',(52.575,4.27969784077511,-0.388783737627976));
#28705=CARTESIAN_POINT('Ctrl Pts',(52.575,4.28954966295039,-0.334806492626263));
#28706=CARTESIAN_POINT('Ctrl Pts',(52.575,4.29833604406102,-0.280694309983832));
#28707=CARTESIAN_POINT('Ctrl Pts',(52.575,4.31910349396582,-0.152795004442932));
#28708=CARTESIAN_POINT('Ctrl Pts',(52.575,4.33392209061696,-0.0241436197492663));
#28709=CARTESIAN_POINT('Ctrl Pts',(52.575,4.3429370549885,0.104855326937507));
#28710=CARTESIAN_POINT('Ctrl Pts',(52.575,4.35209690964512,0.235927570133247));
#28711=CARTESIAN_POINT('Ctrl Pts',(52.575,4.35526523050226,0.367359322916083));
#28712=CARTESIAN_POINT('Ctrl Pts',(52.575,4.35254513857273,0.498747978701545));
#28713=CARTESIAN_POINT('Ctrl Pts',(52.575,4.35009453448373,0.617119557845933));
#28714=CARTESIAN_POINT('Ctrl Pts',(52.575,4.34286386932909,0.735456833565131));
#28715=CARTESIAN_POINT('Ctrl Pts',(52.575,4.33089381744145,0.853472901232893));
#28716=CARTESIAN_POINT('Ctrl Pts',(52.575,4.32191627852572,0.941984951983714));
#28717=CARTESIAN_POINT('Ctrl Pts',(52.575,4.3102721617027,1.03031650957211));
#28718=CARTESIAN_POINT('Ctrl Pts',(52.575,4.2959663745933,1.11834669639071));
#28719=CARTESIAN_POINT('Ctrl Pts',(52.575,4.29282287279567,1.13769013051244));
#28720=CARTESIAN_POINT('Ctrl Pts',(52.575,4.28955081429939,1.1570190093928));
#28721=CARTESIAN_POINT('Ctrl Pts',(52.575,4.28615018278361,1.17633204195954));
#28722=CARTESIAN_POINT('Ctrl Pts',(52.575,4.28275394386741,1.19562012786028));
#28723=CARTESIAN_POINT('Ctrl Pts',(52.575,4.27923064364971,1.21488549512907));
#28724=CARTESIAN_POINT('Ctrl Pts',(52.575,4.27558218993528,1.23411866256198));
#28725=CARTESIAN_POINT('Ctrl Pts',(52.575,4.25019479115831,1.36795072665851));
#28726=CARTESIAN_POINT('Ctrl Pts',(52.575,4.21873023527054,1.50034525531864));
#28727=CARTESIAN_POINT('Ctrl Pts',(52.575,4.18131895579719,1.63087576261264));
#28728=CARTESIAN_POINT('Ctrl Pts',(52.575,4.15599231403848,1.71924214417873));
#28729=CARTESIAN_POINT('Ctrl Pts',(52.575,4.12793922655871,1.80675465116126));
#28730=CARTESIAN_POINT('Ctrl Pts',(52.575,4.09718683849603,1.89328327569644));
#28731=CARTESIAN_POINT('Ctrl Pts',(52.575,4.05202655950391,2.02035167821686));
#28732=CARTESIAN_POINT('Ctrl Pts',(52.575,4.00104762032723,2.14529897660314));
#28733=CARTESIAN_POINT('Ctrl Pts',(52.575,3.94453562255273,2.26782055577994));
#28734=CARTESIAN_POINT('Ctrl Pts',(52.575,3.88754808400084,2.39137313738635));
#28735=CARTESIAN_POINT('Ctrl Pts',(52.575,3.82493370056318,2.51245971712919));
#28736=CARTESIAN_POINT('Ctrl Pts',(52.575,3.75693415592833,2.63075466736293));
#28737=CARTESIAN_POINT('Ctrl Pts',(52.575,3.73798363353152,2.66372181612655));
#28738=CARTESIAN_POINT('Ctrl Pts',(52.575,3.71861457831358,2.69647203588586));
#28739=CARTESIAN_POINT('Ctrl Pts',(52.575,3.69883156699335,2.72899797900061));
#28740=CARTESIAN_POINT('Ctrl Pts',(52.575,3.68688426888272,2.74864095106543));
#28741=CARTESIAN_POINT('Ctrl Pts',(52.575,3.67478598909839,2.76820212301373));
#28742=CARTESIAN_POINT('Ctrl Pts',(52.575,3.66253768792789,2.78767984802252));
#28743=CARTESIAN_POINT('Ctrl Pts',(52.575,3.65179462941252,2.80476387760371));
#28744=CARTESIAN_POINT('Ctrl Pts',(52.575,3.64093526729776,2.8217849699757));
#28745=CARTESIAN_POINT('Ctrl Pts',(52.575,3.62997063555571,2.83872625989296));
#28746=CARTESIAN_POINT('Ctrl Pts',(52.575,3.55452375466503,2.95529811680457));
#28747=CARTESIAN_POINT('Ctrl Pts',(52.575,3.47399253337476,3.06826057686335));
#28748=CARTESIAN_POINT('Ctrl Pts',(52.575,3.38870787807495,3.17730716262715));
#28749=CARTESIAN_POINT('Ctrl Pts',(52.575,3.30236451551238,3.28770743167573));
#28750=CARTESIAN_POINT('Ctrl Pts',(52.575,3.21114868347686,3.39409473557566));
#28751=CARTESIAN_POINT('Ctrl Pts',(52.575,3.11535179231217,3.49613809434228));
#28752=CARTESIAN_POINT('Ctrl Pts',(52.575,3.02057356161899,3.59709637054837));
#28753=CARTESIAN_POINT('Ctrl Pts',(52.575,2.92131071507327,3.69380325966571));
#28754=CARTESIAN_POINT('Ctrl Pts',(52.575,2.8178008233524,3.78591524603509));
#28755=CARTESIAN_POINT('Ctrl Pts',(52.575,2.74290684774614,3.85256233401386));
#28756=CARTESIAN_POINT('Ctrl Pts',(52.575,2.66578852360097,3.91680346413161));
#28757=CARTESIAN_POINT('Ctrl Pts',(52.575,2.58658179140831,3.97858032782616));
#28758=CARTESIAN_POINT('Ctrl Pts',(52.575,2.5515363020237,4.005913868308));
#28759=CARTESIAN_POINT('Ctrl Pts',(52.575,2.51608184050385,4.03276485581719));
#28760=CARTESIAN_POINT('Ctrl Pts',(52.575,2.48022960363516,4.05912758981513));
#28761=CARTESIAN_POINT('Ctrl Pts',(52.575,2.45986381027416,4.07410288954327));
#28762=CARTESIAN_POINT('Ctrl Pts',(52.575,2.43936965724024,4.08892063278838));
#28763=CARTESIAN_POINT('Ctrl Pts',(52.575,2.41874915138383,4.1035797134609));
#28764=CARTESIAN_POINT('Ctrl Pts',(52.575,2.40331173815407,4.11455414287045));
#28765=CARTESIAN_POINT('Ctrl Pts',(52.575,2.38780325084898,4.12543975453688));
#28766=CARTESIAN_POINT('Ctrl Pts',(52.575,2.3722370798148,4.13622757204182));
#28767=CARTESIAN_POINT('Ctrl Pts',(52.575,2.25664941820129,4.21633324456537));
#28768=CARTESIAN_POINT('Ctrl Pts',(52.575,2.13771895193274,4.29116786534254));
#28769=CARTESIAN_POINT('Ctrl Pts',(52.575,2.01587804671584,4.36063651988135));
#28770=CARTESIAN_POINT('Ctrl Pts',(52.575,1.89144332325272,4.43158406251083));
#28771=CARTESIAN_POINT('Ctrl Pts',(52.575,1.76397243333656,4.49693525545565));
#28772=CARTESIAN_POINT('Ctrl Pts',(52.575,1.63388301973716,4.55655608155356));
#28773=CARTESIAN_POINT('Ctrl Pts',(52.575,1.50331587990202,4.61639585269885));
#28774=CARTESIAN_POINT('Ctrl Pts',(52.575,1.37011029782627,4.67046354765956));
#28775=CARTESIAN_POINT('Ctrl Pts',(52.575,1.23465458866001,4.71858364092287));
#28776=CARTESIAN_POINT('Ctrl Pts',(52.575,1.10035291241915,4.76629376865323));
#28777=CARTESIAN_POINT('Ctrl Pts',(52.575,0.96383858689367,4.80815757818582));
#28778=CARTESIAN_POINT('Ctrl Pts',(52.575,0.825466953202148,4.84395867267966));
#28779=CARTESIAN_POINT('Ctrl Pts',(52.575,0.782423633175989,4.85509533361567));
#28780=CARTESIAN_POINT('Ctrl Pts',(52.575,0.739200462732767,4.86564498253008));
#28781=CARTESIAN_POINT('Ctrl Pts',(52.575,0.695807839646318,4.87560011181052));
#28782=CARTESIAN_POINT('',(52.575,-4.925,-6.03138548580072E-16));
#28783=CARTESIAN_POINT('Origin',(52.575,0.,0.));
#28784=CARTESIAN_POINT('',(52.575,-3.42883835300376,3.535500303812));
#28785=CARTESIAN_POINT('Origin',(52.575,0.,0.));
#28786=CARTESIAN_POINT('Ctrl Pts',(52.575,-3.42895049711685,3.53554284596622));
#28787=CARTESIAN_POINT('Ctrl Pts',(52.575,-3.5091582599996,3.4437018410653));
#28788=CARTESIAN_POINT('Ctrl Pts',(52.575,-3.58581516971697,3.34898223367365));
#28789=CARTESIAN_POINT('Ctrl Pts',(52.575,-3.65871286157694,3.25152488213287));
#28790=CARTESIAN_POINT('Ctrl Pts',(52.575,-3.74535381180812,3.13569408791887));
#28791=CARTESIAN_POINT('Ctrl Pts',(52.575,-3.82668584084521,3.01599591002262));
#28792=CARTESIAN_POINT('Ctrl Pts',(52.575,-3.90252529089327,2.89283180460372));
#28793=CARTESIAN_POINT('Ctrl Pts',(52.575,-3.94702892486057,2.82055741097349));
#28794=CARTESIAN_POINT('Ctrl Pts',(52.575,-3.98964028296665,2.74708912931587));
#28795=CARTESIAN_POINT('Ctrl Pts',(52.575,-4.0303141866431,2.67250587749233));
#28796=CARTESIAN_POINT('Ctrl Pts',(52.575,-4.05883144723199,2.62021411703734));
#28797=CARTESIAN_POINT('Ctrl Pts',(52.575,-4.0863961915163,2.56737424131341));
#28798=CARTESIAN_POINT('Ctrl Pts',(52.575,-4.11299101431309,2.51401324086522));
#28799=CARTESIAN_POINT('Ctrl Pts',(52.575,-4.12678190058593,2.48634261135178));
#28800=CARTESIAN_POINT('Ctrl Pts',(52.575,-4.14031387620493,2.4585275644258));
#28801=CARTESIAN_POINT('Ctrl Pts',(52.575,-4.15357199766806,2.43059856460847));
#28802=CARTESIAN_POINT('Ctrl Pts',(52.575,-4.21456648591084,2.30211014671852));
#28803=CARTESIAN_POINT('Ctrl Pts',(52.575,-4.26981904241137,2.17111458465814));
#28804=CARTESIAN_POINT('Ctrl Pts',(52.575,-4.31915508190971,2.03799843572494));
#28805=CARTESIAN_POINT('Ctrl Pts',(52.575,-4.36809647196592,1.90594711109564));
#28806=CARTESIAN_POINT('Ctrl Pts',(52.575,-4.41121576812792,1.77180823660554));
#28807=CARTESIAN_POINT('Ctrl Pts',(52.575,-4.44829212455411,1.63595212520647));
#28808=CARTESIAN_POINT('Ctrl Pts',(52.575,-4.47402001950507,1.54167932983406));
#28809=CARTESIAN_POINT('Ctrl Pts',(52.575,-4.49683707512701,1.44657950014077));
#28810=CARTESIAN_POINT('Ctrl Pts',(52.575,-4.51665446402512,1.35077720141337));
#28811=CARTESIAN_POINT('Ctrl Pts',(52.575,-4.520764031306,1.33091050785917));
#28812=CARTESIAN_POINT('Ctrl Pts',(52.575,-4.52474456023551,1.3110136125633));
#28813=CARTESIAN_POINT('Ctrl Pts',(52.575,-4.5285951898601,1.29108763838625));
#28814=CARTESIAN_POINT('Ctrl Pts',(52.575,-4.53235405480569,1.27163652177849));
#28815=CARTESIAN_POINT('Ctrl Pts',(52.575,-4.53598714894778,1.25216798572193));
#28816=CARTESIAN_POINT('Ctrl Pts',(52.575,-4.53949403976558,1.23268319329843));
#28817=CARTESIAN_POINT('Ctrl Pts',(52.575,-4.54971862223298,1.17587393479983));
#28818=CARTESIAN_POINT('Ctrl Pts',(52.575,-4.55887058507416,1.11892617810197));
#28819=CARTESIAN_POINT('Ctrl Pts',(52.575,-4.56693872807373,1.06186570389229));
#28820=CARTESIAN_POINT('Ctrl Pts',(52.575,-4.58634449454588,0.924621949367475));
#28821=CARTESIAN_POINT('Ctrl Pts',(52.575,-4.59948385775869,0.786726058412982));
#28822=CARTESIAN_POINT('Ctrl Pts',(52.575,-4.60642483762348,0.648594126037778));
#28823=CARTESIAN_POINT('Ctrl Pts',(52.575,-4.61338604128565,0.510059721350728));
#28824=CARTESIAN_POINT('Ctrl Pts',(52.575,-4.61411253459408,0.371287080057338));
#28825=CARTESIAN_POINT('Ctrl Pts',(52.575,-4.60862119457809,0.232702682255874));
#28826=CARTESIAN_POINT('Ctrl Pts',(52.575,-4.60321433808265,0.0962503865976968));
#28827=CARTESIAN_POINT('Ctrl Pts',(52.575,-4.59177921640993,-0.0400201269089059));
#28828=CARTESIAN_POINT('Ctrl Pts',(52.575,-4.57428532046287,-0.175683930093663));
#28829=CARTESIAN_POINT('Ctrl Pts',(52.575,-4.56307295245554,-0.262634972399285));
#28830=CARTESIAN_POINT('Ctrl Pts',(52.575,-4.54937076504609,-0.349336392803606));
#28831=CARTESIAN_POINT('Ctrl Pts',(52.575,-4.5331611772412,-0.435670341473325));
#28832=CARTESIAN_POINT('Ctrl Pts',(52.575,-4.52960784261755,-0.454595770836303));
#28833=CARTESIAN_POINT('Ctrl Pts',(52.575,-4.52593398997846,-0.473503520597655));
#28834=CARTESIAN_POINT('Ctrl Pts',(52.575,-4.52213938767235,-0.492392312214098));
#28835=CARTESIAN_POINT('Ctrl Pts',(52.575,-4.51862284016697,-0.509897001159094));
#28836=CARTESIAN_POINT('Ctrl Pts',(52.575,-4.51500456977891,-0.527375548556558));
#28837=CARTESIAN_POINT('Ctrl Pts',(52.575,-4.51128481062968,-0.544826628462621));
#28838=CARTESIAN_POINT('Ctrl Pts',(52.575,-4.48314127653678,-0.676860731368406));
#28839=CARTESIAN_POINT('Ctrl Pts',(52.575,-4.44919050457636,-0.807332152072528));
#28840=CARTESIAN_POINT('Ctrl Pts',(52.575,-4.40946716653323,-0.935850761402154));
#28841=CARTESIAN_POINT('Ctrl Pts',(52.575,-4.38257279429726,-1.02286327064312));
#28842=CARTESIAN_POINT('Ctrl Pts',(52.575,-4.35303131455946,-1.10898041176107));
#28843=CARTESIAN_POINT('Ctrl Pts',(52.575,-4.32084101271981,-1.19407570764782));
#28844=CARTESIAN_POINT('Ctrl Pts',(52.575,-4.27308791576523,-1.3203113650548));
#28845=CARTESIAN_POINT('Ctrl Pts',(52.575,-4.21950722517578,-1.44430002393767));
#28846=CARTESIAN_POINT('Ctrl Pts',(52.575,-4.16031888017239,-1.56567297532392));
#28847=CARTESIAN_POINT('Ctrl Pts',(52.575,-4.10160823636378,-1.68606634189684));
#28848=CARTESIAN_POINT('Ctrl Pts',(52.575,-4.0373795113942,-1.8038866280582));
#28849=CARTESIAN_POINT('Ctrl Pts',(52.575,-3.96781301876157,-1.91873624560477));
#28850=CARTESIAN_POINT('Ctrl Pts',(52.575,-3.94906135545505,-1.94969398513736));
#28851=CARTESIAN_POINT('Ctrl Pts',(52.575,-3.92992169701845,-1.98043564353625));
#28852=CARTESIAN_POINT('Ctrl Pts',(52.575,-3.91039722592405,-2.01095287666042));
#28853=CARTESIAN_POINT('Ctrl Pts',(52.575,-3.89784596496109,-2.0305708092004));
#28854=CARTESIAN_POINT('Ctrl Pts',(52.575,-3.88513567617724,-2.05009599225496));
#28855=CARTESIAN_POINT('Ctrl Pts',(52.575,-3.87226717680479,-2.06952615257306));
#28856=CARTESIAN_POINT('Ctrl Pts',(52.575,-3.86251730577991,-2.08424749277064));
#28857=CARTESIAN_POINT('Ctrl Pts',(52.575,-3.85267685250824,-2.09891382958667));
#28858=CARTESIAN_POINT('Ctrl Pts',(52.575,-3.84275385977172,-2.11351315437222));
#28859=CARTESIAN_POINT('Ctrl Pts',(52.575,-3.76865945781698,-2.22252545213873));
#28860=CARTESIAN_POINT('Ctrl Pts',(52.575,-3.68985952194509,-2.32796672350722));
#28861=CARTESIAN_POINT('Ctrl Pts',(52.575,-3.60658777099566,-2.42951413079451));
#28862=CARTESIAN_POINT('Ctrl Pts',(52.575,-3.52423547904387,-2.52994028536101));
#28863=CARTESIAN_POINT('Ctrl Pts',(52.575,-3.4375089805729,-2.6265585971069));
#28864=CARTESIAN_POINT('Ctrl Pts',(52.575,-3.34660031521949,-2.71901977384784));
#28865=CARTESIAN_POINT('Ctrl Pts',(52.575,-3.26049006165378,-2.80660059293913));
#28866=CARTESIAN_POINT('Ctrl Pts',(52.575,-3.17062685965888,-2.89045165857665));
#28867=CARTESIAN_POINT('Ctrl Pts',(52.575,-3.07715226412168,-2.97023878224582));
#28868=CARTESIAN_POINT('Ctrl Pts',(52.575,-3.011002341584,-3.02670238093684));
#28869=CARTESIAN_POINT('Ctrl Pts',(52.575,-2.94304325285011,-3.08112987045868));
#28870=CARTESIAN_POINT('Ctrl Pts',(52.575,-2.87337756767158,-3.13344755448078));
#28871=CARTESIAN_POINT('Ctrl Pts',(52.575,-2.83651936368417,-3.16112740669057));
#28872=CARTESIAN_POINT('Ctrl Pts',(52.575,-2.79918341581072,-3.18821652073932));
#28873=CARTESIAN_POINT('Ctrl Pts',(52.575,-2.76138474990579,-3.2147028302475));
#28874=CARTESIAN_POINT('Ctrl Pts',(52.575,-2.74112364039756,-3.22890021009058));
#28875=CARTESIAN_POINT('Ctrl Pts',(52.575,-2.72072957913371,-3.24292437522167));
#28876=CARTESIAN_POINT('Ctrl Pts',(52.575,-2.7002048753135,-3.25677336970125));
#28877=CARTESIAN_POINT('Ctrl Pts',(52.575,-2.68589766540415,-3.26642712513607));
#28878=CARTESIAN_POINT('Ctrl Pts',(52.575,-2.67153123289055,-3.27599285175447));
#28879=CARTESIAN_POINT('Ctrl Pts',(52.575,-2.6571127928066,-3.28546597843703));
#28880=CARTESIAN_POINT('Ctrl Pts',(52.575,-2.54789859172799,-3.35722131093679));
#28881=CARTESIAN_POINT('Ctrl Pts',(52.575,-2.43559227130387,-3.42374252423472));
#28882=CARTESIAN_POINT('Ctrl Pts',(52.575,-2.32058097401746,-3.4848624014124));
#28883=CARTESIAN_POINT('Ctrl Pts',(52.575,-2.20823312579863,-3.54456685520368));
#28884=CARTESIAN_POINT('Ctrl Pts',(52.575,-2.09330325260344,-3.59911731784978));
#28885=CARTESIAN_POINT('Ctrl Pts',(52.575,-1.97613525323649,-3.6483087705229));
#28886=CARTESIAN_POINT('Ctrl Pts',(52.575,-1.85480067208434,-3.6992495080844));
#28887=CARTESIAN_POINT('Ctrl Pts',(52.575,-1.73106512455838,-3.74444394571983));
#28888=CARTESIAN_POINT('Ctrl Pts',(52.575,-1.6053049271685,-3.78360508850387));
#28889=CARTESIAN_POINT('Ctrl Pts',(52.575,-1.48790458016673,-3.82016301261065));
#28890=CARTESIAN_POINT('Ctrl Pts',(52.575,-1.3687391774276,-3.85146273611988));
#28891=CARTESIAN_POINT('Ctrl Pts',(52.575,-1.24812069852349,-3.8772198432059));
#28892=CARTESIAN_POINT('Ctrl Pts',(52.575,-1.23953169122129,-3.8790539567087));
#28893=CARTESIAN_POINT('Ctrl Pts',(52.575,-1.23093532080581,-3.88085994437867));
#28894=CARTESIAN_POINT('Ctrl Pts',(52.575,-1.22233170237281,-3.88263769354989));
#28895=CARTESIAN_POINT('Ctrl Pts',(29.5066541949775,-1.79217368492188,3.65473442716068));
#28896=CARTESIAN_POINT('Ctrl Pts',(29.5462905279758,-2.39896296820844,3.35718290666796));
#28897=CARTESIAN_POINT('Ctrl Pts',(29.6255631939724,-3.46086359021348,2.45430519088321));
#28898=CARTESIAN_POINT('Ctrl Pts',(29.7444721929674,-4.21283764794082,0.502366200250802));
#28899=CARTESIAN_POINT('Ctrl Pts',(29.8633811919624,-3.94100156145658,-1.57116912916543));
#28900=CARTESIAN_POINT('Ctrl Pts',(29.9822901909573,-2.71153768352562,-3.2631402427874));
#28901=CARTESIAN_POINT('Ctrl Pts',(30.1011991899523,-0.823144019015715,
-4.16204660810053));
#28902=CARTESIAN_POINT('Ctrl Pts',(30.2201081889472,1.26526436571728,-4.04962641418862));
#28903=CARTESIAN_POINT('Ctrl Pts',(30.3390171879422,3.04621666442482,-2.95311080905282));
#28904=CARTESIAN_POINT('Ctrl Pts',(30.4579261869372,4.08693028190598,-1.13899868222102));
#28905=CARTESIAN_POINT('Ctrl Pts',(30.5768351859321,4.13451402698658,0.951899428186699));
#28906=CARTESIAN_POINT('Ctrl Pts',(30.6957441849271,3.17740294051253,2.81148064688808));
#28907=CARTESIAN_POINT('Ctrl Pts',(30.814653183922,1.44817770927032,3.9878689759897));
#28908=CARTESIAN_POINT('Ctrl Pts',(30.933562182917,-0.632957413458418,4.19519723441137));
#28909=CARTESIAN_POINT('Ctrl Pts',(31.052471181912,-2.56028269018139,3.38308567277929));
#28910=CARTESIAN_POINT('Ctrl Pts',(31.1713801809069,-3.86545482835077,1.74887813197202));
#28911=CARTESIAN_POINT('Ctrl Pts',(31.2902891799019,-4.23131464672371,-0.310309744443803));
#28912=CARTESIAN_POINT('Ctrl Pts',(31.4091981788968,-3.56895760027616,-2.29409186709539));
#28913=CARTESIAN_POINT('Ctrl Pts',(31.5281071778918,-2.03933759614693,-3.72040561602178));
#28914=CARTESIAN_POINT('Ctrl Pts',(31.6470161768868,-0.0141549844227289,
-4.24265429393642));
#28915=CARTESIAN_POINT('Ctrl Pts',(31.7659251758817,2.01446731467499,-3.73393053486277));
#28916=CARTESIAN_POINT('Ctrl Pts',(31.8848341748767,3.55357052479912,-2.31785511487955));
#28917=CARTESIAN_POINT('Ctrl Pts',(32.0037431738717,4.229149869261,-0.338536837555411));
#28918=CARTESIAN_POINT('Ctrl Pts',(32.1226521728666,3.87703838273484,1.72304648374135));
#28919=CARTESIAN_POINT('Ctrl Pts',(32.2415611718616,2.58279977386025,3.36592648990226));
#28920=CARTESIAN_POINT('Ctrl Pts',(32.3604701708566,0.660936292926016,4.19088045920181));
#28921=CARTESIAN_POINT('Ctrl Pts',(32.4793791698515,-1.42153586561542,3.99744313151944));
#28922=CARTESIAN_POINT('Ctrl Pts',(32.5982881688465,-3.15857231724438,2.83262011635301));
#28923=CARTESIAN_POINT('Ctrl Pts',(32.7171971678415,-4.12807015963076,0.979465448103537));
#28924=CARTESIAN_POINT('Ctrl Pts',(32.8361061668364,-4.09443971780787,-1.11170104079509));
#28925=CARTESIAN_POINT('Ctrl Pts',(32.9550151658314,-3.06585324807998,-2.93272222825354));
#28926=CARTESIAN_POINT('Ctrl Pts',(33.0739241648263,-1.29225906543464,-4.04108677395906));
#28927=CARTESIAN_POINT('Ctrl Pts',(33.1928331638213,0.795356335102055,-4.16746015062799));
#28928=CARTESIAN_POINT('Ctrl Pts',(33.3117421628162,2.68969875215823,-3.2811334062333));
#28929=CARTESIAN_POINT('Ctrl Pts',(33.4306511618112,3.93043965810529,-1.59748549315922));
#28930=CARTESIAN_POINT('Ctrl Pts',(33.5495601608062,4.21607683810534,0.47435419472437));
#28931=CARTESIAN_POINT('Ctrl Pts',(33.6684691598011,3.47719995677159,2.43092498187187));
#28932=CARTESIAN_POINT('Ctrl Pts',(33.7873781587961,1.89335739132502,3.79677673765208));
#28933=CARTESIAN_POINT('Ctrl Pts',(33.906287157791,-0.15057433877126,4.24000509143145));
#28934=CARTESIAN_POINT('Ctrl Pts',(34.025196156786,-2.1579162406289,3.65290477637881));
#28935=CARTESIAN_POINT('Ctrl Pts',(34.144105155781,-3.64088071375389,2.17814219808442));
#28936=CARTESIAN_POINT('Ctrl Pts',(34.2630141547759,-4.23910479193002,0.174087247944916));
#28937=CARTESIAN_POINT('Ctrl Pts',(34.3819231537709,-3.80721897563096,-1.87227120857439));
#28938=CARTESIAN_POINT('Ctrl Pts',(34.5008321527658,-2.45017227519968,-3.46366447981092));
#28939=CARTESIAN_POINT('Ctrl Pts',(34.6197411517608,-0.497729417387068,
-4.21338121156021));
#28940=CARTESIAN_POINT('Ctrl Pts',(34.7386501507558,1.57566256123941,-3.93923892395085));
#28941=CARTESIAN_POINT('Ctrl Pts',(34.8575591497507,3.26616577576251,-2.70785467337129));
#28942=CARTESIAN_POINT('Ctrl Pts',(34.9764681487457,4.16298498204543,-0.818456991005179));
#28943=CARTESIAN_POINT('Ctrl Pts',(35.0953771477406,4.04819154107314,1.26982717471511));
#28944=CARTESIAN_POINT('Ctrl Pts',(35.2142861467356,2.94968046020461,3.04954111130644));
#28945=CARTESIAN_POINT('Ctrl Pts',(35.3331951457306,1.13439185749204,4.0882112128065));
#28946=CARTESIAN_POINT('Ctrl Pts',(35.4521041447256,-0.956555954881787,
4.13343882403517));
#28947=CARTESIAN_POINT('Ctrl Pts',(35.5710131437205,-2.81505899362824,3.17423355619177));
#28948=CARTESIAN_POINT('Ctrl Pts',(35.6899221427155,-3.98949776286473,1.44368397059688));
#28949=CARTESIAN_POINT('Ctrl Pts',(35.8088311417104,-4.1944815831844,-0.637683350251475));
#28950=CARTESIAN_POINT('Ctrl Pts',(35.9277401407054,-3.38019902696682,-2.56409249929749));
#28951=CARTESIAN_POINT('Ctrl Pts',(36.0466491397003,-1.74452218259612,-3.86742267683414));
#28952=CARTESIAN_POINT('Ctrl Pts',(36.1655581386953,0.315076609834192,-4.23096236532504));
#28953=CARTESIAN_POINT('Ctrl Pts',(36.2844671376903,2.29811123382828,-3.56637078327709));
#28954=CARTESIAN_POINT('Ctrl Pts',(36.4033761366852,3.72270080001742,-2.03514484998292));
#28955=CARTESIAN_POINT('Ctrl Pts',(36.5222851356802,4.24266754688635,-0.0093751510681078));
#28956=CARTESIAN_POINT('Ctrl Pts',(36.6411941346751,3.73165864358157,2.01867272598657));
#28957=CARTESIAN_POINT('Ctrl Pts',(36.7601031336701,2.31385014926909,3.55617959242768));
#28958=CARTESIAN_POINT('Ctrl Pts',(36.8790121326651,0.333772013114966,4.22952858485353));
#28959=CARTESIAN_POINT('Ctrl Pts',(36.99792113166,-1.72741330724408,3.87509471792328));
#28960=CARTESIAN_POINT('Ctrl Pts',(37.116830130655,-3.36883416623464,2.57900604248567));
#28961=CARTESIAN_POINT('Ctrl Pts',(37.23573912965,-4.19162241816321,0.65621437846393));
#28962=CARTESIAN_POINT('Ctrl Pts',(37.3546481286449,-3.99583907563888,-1.42603852981441));
#28963=CARTESIAN_POINT('Ctrl Pts',(37.4735571276399,-2.82905983413317,-3.16176157564063));
#28964=CARTESIAN_POINT('Ctrl Pts',(37.5924661266349,-0.974814094226818,
-4.12917101732149));
#28965=CARTESIAN_POINT('Ctrl Pts',(37.7113751256298,1.11631317895359,-4.09318466350003));
#28966=CARTESIAN_POINT('Ctrl Pts',(37.8302841246248,2.93617439347552,-3.06254726405115));
#28967=CARTESIAN_POINT('Ctrl Pts',(37.9491931236197,4.04254008318163,-1.28770550784711));
#28968=CARTESIAN_POINT('Ctrl Pts',(38.0681021226147,4.16656144887969,0.800050936289306));
#28969=CARTESIAN_POINT('Ctrl Pts',(38.1870111216096,3.27810107619118,2.69339361556102));
#28970=CARTESIAN_POINT('Ctrl Pts',(38.3059201206047,1.593056403167,3.93223689564486));
#28971=CARTESIAN_POINT('Ctrl Pts',(38.4248291195996,-0.479103781660292,
4.21553977736235));
#28972=CARTESIAN_POINT('Ctrl Pts',(38.5437381185946,-2.43484088061553,3.47445898581872));
#28973=CARTESIAN_POINT('Ctrl Pts',(38.6626471175895,-3.79890743219015,1.88907880761477));
#28974=CARTESIAN_POINT('Ctrl Pts',(38.7815561165844,-4.23983271101909,-0.155351304211019));
#28975=CARTESIAN_POINT('Ctrl Pts',(38.9004651155794,-3.65047142573015,-2.16202983439362));
#28976=CARTESIAN_POINT('Ctrl Pts',(39.0193741145744,-2.17403875473271,-3.64333320582671));
#28977=CARTESIAN_POINT('Ctrl Pts',(39.1382831135694,-0.169311715692027,
-4.23929647022592));
#28978=CARTESIAN_POINT('Ctrl Pts',(39.2571921125643,1.87656008277306,-3.80511074896768));
#28979=CARTESIAN_POINT('Ctrl Pts',(39.3761011115593,3.46642106848062,-2.4462615072031));
#28980=CARTESIAN_POINT('Ctrl Pts',(39.4950101105543,4.21394248995934,-0.49299624037214));
#28981=CARTESIAN_POINT('Ctrl Pts',(39.6139191095491,3.93745486993259,1.58012745604));
#28982=CARTESIAN_POINT('Ctrl Pts',(39.7328281085442,2.7041860128382,3.26915872948103));
#28983=CARTESIAN_POINT('Ctrl Pts',(39.8517371075391,0.813740946052253,4.1640155130528));
#28984=CARTESIAN_POINT('Ctrl Pts',(39.9706461065341,-1.27433631150534,4.04653670722897));
#28985=CARTESIAN_POINT('Ctrl Pts',(40.089555105529,-3.05296367944959,2.94668522964312));
#28986=CARTESIAN_POINT('Ctrl Pts',(40.208464104524,-4.08928438704866,1.12890284381863));
#28987=CARTESIAN_POINT('Ctrl Pts',(40.327373103519,-4.13276214523759,-0.959452031103675));
#28988=CARTESIAN_POINT('Ctrl Pts',(40.4462821025139,-3.17025406296392,-2.82213573711675));
#28989=CARTESIAN_POINT('Ctrl Pts',(40.5651911015089,-1.44080558796838,-3.98425201455624));
#28990=CARTESIAN_POINT('Ctrl Pts',(40.7237364335021,1.3412377851549,-4.2793985106552));
#28991=CARTESIAN_POINT('Ctrl Pts',(40.9219180984939,4.38508550900277,-1.98115657932714));
#28992=CARTESIAN_POINT('Ctrl Pts',(41.1597360964836,4.03738561363306,2.61791400162535));
#28993=CARTESIAN_POINT('Ctrl Pts',(41.3579177614753,0.682606151108172,4.43240558295318));
#28994=CARTESIAN_POINT('Ctrl Pts',(41.5164630934686,-2.02344151873906,3.72234728068988));
#28995=CARTESIAN_POINT('Ctrl Pts',(41.6353720924636,-3.55851387613991,2.31342601692174));
#28996=CARTESIAN_POINT('Ctrl Pts',(41.7542810914585,-4.23003633407526,0.327205992458881));
#28997=CARTESIAN_POINT('Ctrl Pts',(41.8731900904534,-3.87307885762452,-1.73087509415429));
#28998=CARTESIAN_POINT('Ctrl Pts',(41.9920990894484,-2.5752427483792,-3.37219006842077));
#28999=CARTESIAN_POINT('Ctrl Pts',(42.1110080884434,-0.651474736920205,
-4.19213227664958));
#29000=CARTESIAN_POINT('Ctrl Pts',(42.2299170874383,1.43053091718906,-3.99434360254506));
#29001=CARTESIAN_POINT('Ctrl Pts',(42.3488260864333,3.16495106439444,-2.82543900138727));
#29002=CARTESIAN_POINT('Ctrl Pts',(42.4677350854282,4.13026450704979,-0.970190049367721));
#29003=CARTESIAN_POINT('Ctrl Pts',(42.5866440844232,4.09192548053664,1.12093820678962));
#29004=CARTESIAN_POINT('Ctrl Pts',(42.7055530834182,3.05923685698906,2.9396156616928));
#29005=CARTESIAN_POINT('Ctrl Pts',(42.8244620824131,1.28315058703404,4.04399185547656));
#29006=CARTESIAN_POINT('Ctrl Pts',(42.9433710814081,-0.804744663182227,
4.16565565627073));
#29007=CARTESIAN_POINT('Ctrl Pts',(43.0622800804031,-2.69708497911968,3.27506549112629));
#29008=CARTESIAN_POINT('Ctrl Pts',(43.181189079398,-3.93402920382485,1.58862483246787));
#29009=CARTESIAN_POINT('Ctrl Pts',(43.300098078393,-4.21499729336116,-0.483852521028536));
#29010=CARTESIAN_POINT('Ctrl Pts',(43.419007077388,-3.47171372465588,-2.43875382803693));
#29011=CARTESIAN_POINT('Ctrl Pts',(43.5379160763829,-1.88479759986051,-3.80103319712063));
#29012=CARTESIAN_POINT('Ctrl Pts',(43.6568250753779,0.160127627215037,-4.23965507926387));
#29013=CARTESIAN_POINT('Ctrl Pts',(43.7757340743728,2.16614156925702,-3.64803322477728));
#29014=CARTESIAN_POINT('Ctrl Pts',(43.8946430733678,3.64577930876166,-2.16993296345209));
#29015=CARTESIAN_POINT('Ctrl Pts',(44.0135520723628,4.23948628841551,-0.1645351582025));
#29016=CARTESIAN_POINT('Ctrl Pts',(44.1324610713577,3.80299066814145,1.88084496359989));
#29017=CARTESIAN_POINT('Ctrl Pts',(44.2513700703527,2.44236165043659,3.46917647027723));
#29018=CARTESIAN_POINT('Ctrl Pts',(44.3702790693477,0.488234470571936,4.21449201028578));
#29019=CARTESIAN_POINT('Ctrl Pts',(44.4891880683426,-1.58453454124508,3.93567860682148));
#29020=CARTESIAN_POINT('Ctrl Pts',(44.6080970673376,-3.27225888233889,2.70048840272595));
#29021=CARTESIAN_POINT('Ctrl Pts',(44.7270060663325,-4.16481857957887,0.809074784004825));
#29022=CARTESIAN_POINT('Ctrl Pts',(44.8459150653275,-4.04532006216723,-1.27894542556692));
#29023=CARTESIAN_POINT('Ctrl Pts',(44.9648240643225,-2.94280167925739,-3.05617965494951));
#29024=CARTESIAN_POINT('Ctrl Pts',(45.0837330633174,-1.12517733033491,-4.09075687156072));
#29025=CARTESIAN_POINT('Ctrl Pts',(45.2026420623124,0.965867082001261,-4.13127299833094));
#29026=CARTESIAN_POINT('Ctrl Pts',(45.3215510613073,2.82220410049894,-3.16788254548659));
#29027=CARTESIAN_POINT('Ctrl Pts',(45.4404600603023,3.99274057599417,-1.43469108161613));
#29028=CARTESIAN_POINT('Ctrl Pts',(45.5593690592973,4.193034093298,0.647132829719501));
#29029=CARTESIAN_POINT('Ctrl Pts',(45.6782780582922,3.37441297664422,2.57170232918147));
#29030=CARTESIAN_POINT('Ctrl Pts',(45.7971870572872,1.73580359220705,3.87134365513335));
#29031=CARTESIAN_POINT('Ctrl Pts',(45.9160960562822,-0.324609107543747,
4.23024168744071));
#29032=CARTESIAN_POINT('Ctrl Pts',(46.0350050552771,-2.306141225207,3.56118357519822));
#29033=CARTESIAN_POINT('Ctrl Pts',(46.1539140542721,-3.7272769830857,2.02675161236416));
#29034=CARTESIAN_POINT('Ctrl Pts',(46.272823053267,-4.24267790113794,-0.000184544637164212));
#29035=CARTESIAN_POINT('Ctrl Pts',(46.391732052262,-3.72710065291479,-2.02707585696816));
#29036=CARTESIAN_POINT('Ctrl Pts',(46.5106410512569,-2.30583141340579,-3.56138418312489));
#29037=CARTESIAN_POINT('Ctrl Pts',(46.6295500502519,-0.324241098922964,
-4.23026991061211));
#29038=CARTESIAN_POINT('Ctrl Pts',(46.7484590492469,1.73614037090757,-3.87119263526966));
#29039=CARTESIAN_POINT('Ctrl Pts',(46.8673680482418,3.37463668760993,-2.57140876437375));
#29040=CARTESIAN_POINT('Ctrl Pts',(46.9862770472368,4.1930903743722,-0.646768056731501));
#29041=CARTESIAN_POINT('Ctrl Pts',(47.1051860462317,3.99261575077701,1.43503842231084));
#29042=CARTESIAN_POINT('Ctrl Pts',(47.2240950452267,2.82192850173731,3.16812804948658));
#29043=CARTESIAN_POINT('Ctrl Pts',(47.3430040442217,0.965507680676692,4.13135700774157));
#29044=CARTESIAN_POINT('Ctrl Pts',(47.4619130432167,-1.12553319906949,4.0906589719327));
#29045=CARTESIAN_POINT('Ctrl Pts',(47.5808220422116,-2.943067538678,3.05592363609448));
#29046=CARTESIAN_POINT('Ctrl Pts',(47.6997310412065,-4.04543130796411,1.27859350045461));
#29047=CARTESIAN_POINT('Ctrl Pts',(47.8186400402016,-4.16474817883747,-0.809437096833958));
#29048=CARTESIAN_POINT('Ctrl Pts',(47.9375490391964,-3.27202394254474,-2.70077306086147));
#29049=CARTESIAN_POINT('Ctrl Pts',(48.0564580381915,-1.58419215321593,-3.93581643735453));
#29050=CARTESIAN_POINT('Ctrl Pts',(48.1753670371864,0.48860110601671,-4.21444952111902));
#29051=CARTESIAN_POINT('Ctrl Pts',(48.2942760361814,2.44266344009801,-3.46896398442958));
#29052=CARTESIAN_POINT('Ctrl Pts',(48.4131850351763,3.80315427688869,-1.88051411934194));
#29053=CARTESIAN_POINT('Ctrl Pts',(48.5320940341713,4.23947195846584,0.164903972792664));
#29054=CARTESIAN_POINT('Ctrl Pts',(48.6510030331663,3.6455905234561,2.17025011050524));
#29055=CARTESIAN_POINT('Ctrl Pts',(48.7699120321612,2.16582420148474,3.64822166748742));
#29056=CARTESIAN_POINT('Ctrl Pts',(48.8888210311562,0.159758802432322,4.23966896489628));
#29057=CARTESIAN_POINT('Ctrl Pts',(49.0077300301511,-1.88512826562663,3.80086927281119));
#29058=CARTESIAN_POINT('Ctrl Pts',(49.1266390291461,-3.47192586100346,2.43845168550668));
#29059=CARTESIAN_POINT('Ctrl Pts',(49.2455480281411,-4.21503938678446,0.483486064662875));
#29060=CARTESIAN_POINT('Ctrl Pts',(49.364457027136,-3.93389095371854,-1.58896751732501));
#29061=CARTESIAN_POINT('Ctrl Pts',(49.483366026131,-2.69680012382729,-3.27529920754662));
#29062=CARTESIAN_POINT('Ctrl Pts',(49.6022750251259,-0.804382137054723,
-4.16572744962391));
#29063=CARTESIAN_POINT('Ctrl Pts',(49.7211840241209,1.28350211887322,-4.04387661996188));
#29064=CARTESIAN_POINT('Ctrl Pts',(49.8400930231158,3.05949311031172,-2.93935668390779));
#29065=CARTESIAN_POINT('Ctrl Pts',(49.9590020221109,4.09202191338058,-1.12056792152273));
#29066=CARTESIAN_POINT('Ctrl Pts',(50.0779110211058,4.13018221941277,0.970520809410563));
#29067=CARTESIAN_POINT('Ctrl Pts',(50.1968200201008,3.16470100669801,2.82577128347271));
#29068=CARTESIAN_POINT('Ctrl Pts',(50.3157290190956,1.43019190307756,3.99435438105406));
#29069=CARTESIAN_POINT('Ctrl Pts',(50.4346380180907,-0.651856340959766,
4.1923023665036));
#29070=CARTESIAN_POINT('Ctrl Pts',(50.5535470170856,-2.57550234917945,3.37151352187054));
#29071=CARTESIAN_POINT('Ctrl Pts',(50.6724560160807,-3.87329677722202,1.73144099605029));
#29072=CARTESIAN_POINT('Ctrl Pts',(50.7913650150755,-4.22987328984736,-0.329374754514203));
#29073=CARTESIAN_POINT('Ctrl Pts',(50.9102740140706,-3.55858319850174,-2.31015180666798));
#29074=CARTESIAN_POINT('Ctrl Pts',(51.0291830130655,-2.02255111411372,-3.72955803196629));
#29075=CARTESIAN_POINT('Ctrl Pts',(51.1480920120605,0.00496435909204525,
-4.24267489657216));
#29076=CARTESIAN_POINT('Ctrl Pts',(51.2670010110554,2.03127363780405,-3.72481476796509));
#29077=CARTESIAN_POINT('Ctrl Pts',(51.3859100100504,3.56397955602096,-2.30181723828556));
#29078=CARTESIAN_POINT('Ctrl Pts',(51.5048190090453,4.23063280642202,-0.3194758487847));
#29079=CARTESIAN_POINT('Ctrl Pts',(51.6237280080403,3.86923365048362,1.74050225085362));
#29080=CARTESIAN_POINT('Ctrl Pts',(51.7426370070353,2.56760636844359,3.37752823139821));
#29081=CARTESIAN_POINT('Ctrl Pts',(51.8615460060302,0.642041384412004,4.19382294217941));
#29082=CARTESIAN_POINT('Ctrl Pts',(51.9804550050252,-1.43953109567099,3.99098337113032));
#29083=CARTESIAN_POINT('Ctrl Pts',(52.0993640040201,-3.17131432296482,2.81838363574518));
#29084=CARTESIAN_POINT('Ctrl Pts',(52.2182730030151,-4.13242404491094,0.960800318946468));
#29085=CARTESIAN_POINT('Ctrl Pts',(52.3371820020101,-4.08942446914233,-1.13003555618484));
#29086=CARTESIAN_POINT('Ctrl Pts',(52.456091001005,-3.05253321900086,-2.94673237789893));
#29087=CARTESIAN_POINT('Ctrl Pts',(52.5353636670017,-1.86695937376299,-3.67969605923878));
#29088=CARTESIAN_POINT('Ctrl Pts',(52.575,-1.2223317023727,-3.88263769354992));
#29089=CARTESIAN_POINT('Ctrl Pts',(29.6711027966516,-1.91758108071809,3.91047455474607));
#29090=CARTESIAN_POINT('Ctrl Pts',(29.71073912965,-2.5668304583885,3.5921018596015));
#29091=CARTESIAN_POINT('Ctrl Pts',(29.7900117956466,-3.70303760141909,2.62604525439793));
#29092=CARTESIAN_POINT('Ctrl Pts',(29.9089207946415,-4.50763106153991,0.537519286940777));
#29093=CARTESIAN_POINT('Ctrl Pts',(30.0278297936365,-4.21677323850402,-1.68111172596939));
#29094=CARTESIAN_POINT('Ctrl Pts',(30.1467387926315,-2.9012775967691,-3.49147855810178));
#29095=CARTESIAN_POINT('Ctrl Pts',(30.2656477916264,-0.880743541125958,
-4.45328591749101));
#29096=CARTESIAN_POINT('Ctrl Pts',(30.3845567906214,1.35380126949692,-4.33299911786337));
#29097=CARTESIAN_POINT('Ctrl Pts',(30.5034657896164,3.25937574723617,-3.15975480744252));
#29098=CARTESIAN_POINT('Ctrl Pts',(30.6223747886113,4.3729133246025,-1.21870014182534));
#29099=CARTESIAN_POINT('Ctrl Pts',(30.7412837876063,4.42382674336541,1.01850861308497));
#29100=CARTESIAN_POINT('Ctrl Pts',(30.8601927866012,3.39974178608172,3.00821407134581));
#29101=CARTESIAN_POINT('Ctrl Pts',(30.9791017855962,1.54951397857154,4.26692020147249));
#29102=CARTESIAN_POINT('Ctrl Pts',(31.0980107845912,-0.677248623367102,
4.48875625965845));
#29103=CARTESIAN_POINT('Ctrl Pts',(31.2169197835861,-2.73943853170453,3.6198171723813));
#29104=CARTESIAN_POINT('Ctrl Pts',(31.3358287825811,-4.13594012097048,1.87125592043129));
#29105=CARTESIAN_POINT('Ctrl Pts',(31.4547377815761,-4.52740098874766,-0.332023676116975));
#29106=CARTESIAN_POINT('Ctrl Pts',(31.573646780571,-3.81869549238083,-2.45462099950604));
#29107=CARTESIAN_POINT('Ctrl Pts',(31.692555779566,-2.18204029245024,-3.98074108659382));
#29108=CARTESIAN_POINT('Ctrl Pts',(31.811464778561,-0.0151454797909917,
-4.53953412804105));
#29109=CARTESIAN_POINT('Ctrl Pts',(31.9303737775559,2.15542971244672,-3.99521241194915));
#29110=CARTESIAN_POINT('Ctrl Pts',(32.0492827765509,3.80223170593499,-2.48004708111342));
#29111=CARTESIAN_POINT('Ctrl Pts',(32.1681917755458,4.52508473093102,-0.362225960733676));
#29112=CARTESIAN_POINT('Ctrl Pts',(32.2871007745408,4.14833423484531,1.84361670200747));
#29113=CARTESIAN_POINT('Ctrl Pts',(32.4060097735358,2.76353124884398,3.60145727527845));
#29114=CARTESIAN_POINT('Ctrl Pts',(32.5249187725307,0.707185325584214,4.48413741800195));
#29115=CARTESIAN_POINT('Ctrl Pts',(32.6438277715257,-1.5210078712796,4.27716430876084));
#29116=CARTESIAN_POINT('Ctrl Pts',(32.7627367705206,-3.37959348950701,3.03083277568429));
#29117=CARTESIAN_POINT('Ctrl Pts',(32.8816457695156,-4.41693196623964,1.04800356589453));
#29118=CARTESIAN_POINT('Ctrl Pts',(33.0005547685106,-4.38094823345843,-1.1894923472979));
#29119=CARTESIAN_POINT('Ctrl Pts',(33.1194637675055,-3.28038640129495,-3.13793953522177));
#29120=CARTESIAN_POINT('Ctrl Pts',(33.2383727665005,-1.38268492396259,-4.32386191610767));
#29121=CARTESIAN_POINT('Ctrl Pts',(33.3572817654954,0.851011413376168,-4.4590782727843));
#29122=CARTESIAN_POINT('Ctrl Pts',(33.4761907644904,2.87791048566509,-3.51073079358346));
#29123=CARTESIAN_POINT('Ctrl Pts',(33.5950997634854,4.20547226571702,-1.70926957815328));
#29124=CARTESIAN_POINT('Ctrl Pts',(33.7140087624804,4.51109691411248,0.507547140668087));
#29125=CARTESIAN_POINT('Ctrl Pts',(33.8329177614753,3.72051710561174,2.60102901471052));
#29126=CARTESIAN_POINT('Ctrl Pts',(33.9518267604703,2.02584511935904,4.06245627925823));
#29127=CARTESIAN_POINT('Ctrl Pts',(34.0707357594652,-0.161110781671782,
4.53669954752843));
#29128=CARTESIAN_POINT('Ctrl Pts',(34.1896447584602,-2.30891648037153,3.90851687410766));
#29129=CARTESIAN_POINT('Ctrl Pts',(34.3085537574551,-3.89565142741744,2.33055774967624));
#29130=CARTESIAN_POINT('Ctrl Pts',(34.4274627564501,-4.53573624954818,0.186269007218487));
#29131=CARTESIAN_POINT('Ctrl Pts',(34.546371755445,-4.07362921308556,-2.00328343047395));
#29132=CARTESIAN_POINT('Ctrl Pts',(34.66528075444,-2.62162313784214,-3.70603448333205));
#29133=CARTESIAN_POINT('Ctrl Pts',(34.784189753435,-0.532558045086988,-4.50821266103637));
#29134=CARTESIAN_POINT('Ctrl Pts',(34.9030987524299,1.68591958605854,-4.21488726039734));
#29135=CARTESIAN_POINT('Ctrl Pts',(35.0220077514249,3.49471580281806,-2.89733686789252));
#29136=CARTESIAN_POINT('Ctrl Pts',(35.1409167504199,4.4542899541748,-0.875728538220039));
#29137=CARTESIAN_POINT('Ctrl Pts',(35.2598257494149,4.33146383946785,1.35868336116181));
#29138=CARTESIAN_POINT('Ctrl Pts',(35.3787347484098,3.15608441985291,3.26293282236661));
#29139=CARTESIAN_POINT('Ctrl Pts',(35.4976437474048,1.21377095442749,4.37428388867294));
#29140=CARTESIAN_POINT('Ctrl Pts',(35.6165527463997,-1.02349098034518,4.42267630306216));
#29141=CARTESIAN_POINT('Ctrl Pts',(35.7354617453947,-3.01204281298337,3.39635062401849));
#29142=CARTESIAN_POINT('Ctrl Pts',(35.8543707443896,-4.26866296274744,1.54470579042862));
#29143=CARTESIAN_POINT('Ctrl Pts',(35.9732797433846,-4.48799053072001,-0.68230525769852));
#29144=CARTESIAN_POINT('Ctrl Pts',(36.0921887423795,-3.61672853346016,-2.74351493230322));
#29145=CARTESIAN_POINT('Ctrl Pts',(36.2110977413746,-1.86659516339526,-4.1380456696978));
#29146=CARTESIAN_POINT('Ctrl Pts',(36.3300067403695,0.337124103025285,-4.52702405644983));
#29147=CARTESIAN_POINT('Ctrl Pts',(36.4489157393645,2.4589216215207,-3.81592766280134));
#29148=CARTESIAN_POINT('Ctrl Pts',(36.5678247383594,3.9831968761436,-2.17755415877468));
#29149=CARTESIAN_POINT('Ctrl Pts',(36.6867337373544,4.53954830836646,-0.0100311774848461));
#29150=CARTESIAN_POINT('Ctrl Pts',(36.8056427363494,3.99278154502206,2.15992939751383));
#29151=CARTESIAN_POINT('Ctrl Pts',(36.9245517353443,2.47576186794007,3.80502334313229));
#29152=CARTESIAN_POINT('Ctrl Pts',(37.0434607343393,0.357127717590833,4.52548994715605));
#29153=CARTESIAN_POINT('Ctrl Pts',(37.1623697333342,-1.84828909408761,4.14625456204281));
#29154=CARTESIAN_POINT('Ctrl Pts',(37.2812787323292,-3.60456841633064,2.75947205102715));
#29155=CARTESIAN_POINT('Ctrl Pts',(37.4001877313241,-4.48493129555913,0.702132995046478));
#29156=CARTESIAN_POINT('Ctrl Pts',(37.5190967303191,-4.27544800903229,-1.52582560951193));
#29157=CARTESIAN_POINT('Ctrl Pts',(37.6380057293141,-3.02702336263229,-3.38300591633462));
#29158=CARTESIAN_POINT('Ctrl Pts',(37.756914728309,-1.04302673342079,-4.4181098564732));
#29159=CARTESIAN_POINT('Ctrl Pts',(37.875823727304,1.19442721993263,-4.37960535669586));
#29160=CARTESIAN_POINT('Ctrl Pts',(37.994732726299,3.14163326578642,-3.27684908095586));
#29161=CARTESIAN_POINT('Ctrl Pts',(38.113641725294,4.32541692067733,-1.37781273107568));
#29162=CARTESIAN_POINT('Ctrl Pts',(38.2325507242888,4.45811668435999,0.856034519392032));
#29163=CARTESIAN_POINT('Ctrl Pts',(38.3514597232839,3.50748627617526,2.88186389722148));
#29164=CARTESIAN_POINT('Ctrl Pts',(38.4703687222788,1.70453056248457,4.20739526499576));
#29165=CARTESIAN_POINT('Ctrl Pts',(38.5892777212738,-0.51262908006167,4.51052227253135));
#29166=CARTESIAN_POINT('Ctrl Pts',(38.7081867202687,-2.60521892856097,3.7175843351519));
#29167=CARTESIAN_POINT('Ctrl Pts',(38.8270957192637,-4.06473606919677,2.02126714165294));
#29168=CARTESIAN_POINT('Ctrl Pts',(38.9460047182586,-4.53651510479265,-0.166222015380657));
#29169=CARTESIAN_POINT('Ctrl Pts',(39.0649137172536,-3.90591324969007,-2.31331792295678));
#29170=CARTESIAN_POINT('Ctrl Pts',(39.1838227162486,-2.32616716777937,-3.89827553268081));
#29171=CARTESIAN_POINT('Ctrl Pts',(39.3027317152435,-0.181159306983774,
-4.53594134053735));
#29172=CARTESIAN_POINT('Ctrl Pts',(39.4216407142385,2.00787241874566,-4.07137346321188));
#29173=CARTESIAN_POINT('Ctrl Pts',(39.5405497132335,3.70898396435881,-2.61743871376292));
#29174=CARTESIAN_POINT('Ctrl Pts',(39.6594587122284,4.50881321490469,-0.527493663899006));
#29175=CARTESIAN_POINT('Ctrl Pts',(39.7783677112234,4.21297836715714,1.69069691197792));
#29176=CARTESIAN_POINT('Ctrl Pts',(39.8972767102183,2.89341149275226,3.4979181885435));
#29177=CARTESIAN_POINT('Ctrl Pts',(40.0161857092133,0.870682487910497,4.45539259661367));
#29178=CARTESIAN_POINT('Ctrl Pts',(40.1350947082083,-1.36350802490509,4.32969320858648));
#29179=CARTESIAN_POINT('Ctrl Pts',(40.2540037072032,-3.26659488479615,3.15287959796235));
#29180=CARTESIAN_POINT('Ctrl Pts',(40.3729127061982,-4.37543215830797,1.20789784689305));
#29181=CARTESIAN_POINT('Ctrl Pts',(40.4918217051931,-4.42195227364979,-1.02658970956888));
#29182=CARTESIAN_POINT('Ctrl Pts',(40.6107307041881,-3.39209266565834,-3.01961475176409));
#29183=CARTESIAN_POINT('Ctrl Pts',(40.729639703183,-1.54162599290793,-4.26305014307757));
#29184=CARTESIAN_POINT('Ctrl Pts',(40.8881850351763,1.43509093074836,-4.57884952218982));
#29185=CARTESIAN_POINT('Ctrl Pts',(41.086366700168,4.69193197073497,-2.11978805760871));
#29186=CARTESIAN_POINT('Ctrl Pts',(41.3241846981578,4.31990176700075,2.80110259552361));
#29187=CARTESIAN_POINT('Ctrl Pts',(41.5223663631495,0.730371532602854,4.74256326797414));
#29188=CARTESIAN_POINT('Ctrl Pts',(41.6809116951428,-2.16503188665146,3.98281861929281));
#29189=CARTESIAN_POINT('Ctrl Pts',(41.7998206941377,-3.80752096840224,2.47530805692173));
#29190=CARTESIAN_POINT('Ctrl Pts',(41.9187296931327,-4.52603322614153,0.350102239484753));
#29191=CARTESIAN_POINT('Ctrl Pts',(42.0376386921276,-4.14409764187218,-1.85199311961837));
#29192=CARTESIAN_POINT('Ctrl Pts',(42.1565476911226,-2.75544542032698,-3.60815914785125));
#29193=CARTESIAN_POINT('Ctrl Pts',(42.2754566901175,-0.697061696974139,
-4.48547683140511));
#29194=CARTESIAN_POINT('Ctrl Pts',(42.3943656891125,1.53063235179888,-4.27384789017351));
#29195=CARTESIAN_POINT('Ctrl Pts',(42.5132746881075,3.38641858963907,-3.02314916202976));
#29196=CARTESIAN_POINT('Ctrl Pts',(42.6321836871024,4.41927986317098,-1.03807912091381));
#29197=CARTESIAN_POINT('Ctrl Pts',(42.7510926860974,4.37825806237496,1.19937588420037));
#29198=CARTESIAN_POINT('Ctrl Pts',(42.8700016850923,3.27330702808166,3.14531533682823));
#29199=CARTESIAN_POINT('Ctrl Pts',(42.9889106840873,1.37293907957147,4.32697028077277));
#29200=CARTESIAN_POINT('Ctrl Pts',(43.1078196830823,-0.861056689934789,
4.45714750889189));
#29201=CARTESIAN_POINT('Ctrl Pts',(43.2267286820772,-2.88581356403206,3.50423827597399));
#29202=CARTESIAN_POINT('Ctrl Pts',(43.3456376810722,-4.20931298998283,1.69978889252144));
#29203=CARTESIAN_POINT('Ctrl Pts',(43.4645466800671,-4.50994182819939,-0.517710112579008));
#29204=CARTESIAN_POINT('Ctrl Pts',(43.5834556790622,-3.71464697427457,-2.6094056845703));
#29205=CARTESIAN_POINT('Ctrl Pts',(43.7023646780571,-2.01668635628528,-4.06701058457831));
#29206=CARTESIAN_POINT('Ctrl Pts',(43.8212736770521,0.171332561699331,-4.53632504325118));
#29207=CARTESIAN_POINT('Ctrl Pts',(43.940182676047,2.31771737656405,-3.90330443556811));
#29208=CARTESIAN_POINT('Ctrl Pts',(44.0590916750419,3.90089280172621,-2.32177407365723));
#29209=CARTESIAN_POINT('Ctrl Pts',(44.178000674037,4.53614444125922,-0.176048509771458));
#29210=CARTESIAN_POINT('Ctrl Pts',(44.2969096730319,4.06910502967991,2.01245713420922));
#29211=CARTESIAN_POINT('Ctrl Pts',(44.4158186720269,2.61326596442736,3.71193217546101));
#29212=CARTESIAN_POINT('Ctrl Pts',(44.5347276710218,0.522398689144923,4.50940118792892));
#29213=CARTESIAN_POINT('Ctrl Pts',(44.6536366700168,-1.69541238307399,4.21107780999301));
#29214=CARTESIAN_POINT('Ctrl Pts',(44.7725456690117,-3.50123527467057,2.88945514228534));
#29215=CARTESIAN_POINT('Ctrl Pts',(44.8914546680068,-4.45625185773881,0.865689811063943));
#29216=CARTESIAN_POINT('Ctrl Pts',(45.0103636670016,-4.3283914287579,-1.36843966183164));
#29217=CARTESIAN_POINT('Ctrl Pts',(45.1292726659967,-3.14872429604695,-3.27003589825739));
#29218=CARTESIAN_POINT('Ctrl Pts',(45.2481816649915,-1.2039116405156,-4.37700767995842));
#29219=CARTESIAN_POINT('Ctrl Pts',(45.3670906639866,1.03345365380405,-4.42035892365329));
#29220=CARTESIAN_POINT('Ctrl Pts',(45.4859996629815,3.01968789887557,-3.3895552011897));
#29221=CARTESIAN_POINT('Ctrl Pts',(45.6049086619765,4.27213269180196,-1.53508362382972));
#29222=CARTESIAN_POINT('Ctrl Pts',(45.7238176609714,4.48644175269473,0.692415964714791));
#29223=CARTESIAN_POINT('Ctrl Pts',(45.8427266599664,3.61053760413,2.7516572602125));
#29224=CARTESIAN_POINT('Ctrl Pts',(45.9616356589614,1.85726648943845,4.14224101854581));
#29225=CARTESIAN_POINT('Ctrl Pts',(46.0805446579563,-0.34732363748649,4.52625294911356));
#29226=CARTESIAN_POINT('Ctrl Pts',(46.1994536569513,-2.46751351173521,3.81037747971504));
#29227=CARTESIAN_POINT('Ctrl Pts',(46.3183626559463,-3.98809327772981,2.16857360415595));
#29228=CARTESIAN_POINT('Ctrl Pts',(46.4372716549412,-4.53955938715706,-0.000197458152468345));
#29229=CARTESIAN_POINT('Ctrl Pts',(46.5561806539361,-3.98790460885106,-2.1689205377837));
#29230=CARTESIAN_POINT('Ctrl Pts',(46.6750896529312,-2.46718202084595,-3.81059212518606));
#29231=CARTESIAN_POINT('Ctrl Pts',(46.7939986519261,-0.346929877453853,
-4.52628314720205));
#29232=CARTESIAN_POINT('Ctrl Pts',(46.912907650921,1.85762683423641,-4.14207943106362));
#29233=CARTESIAN_POINT('Ctrl Pts',(47.031816649916,3.61077696927579,-2.75134315320047));
#29234=CARTESIAN_POINT('Ctrl Pts',(47.1507256489109,4.48650197203841,-0.692025666728421));
#29235=CARTESIAN_POINT('Ctrl Pts',(47.269634647906,4.27199913193732,1.53545526969767));
#29236=CARTESIAN_POINT('Ctrl Pts',(47.3885436469008,3.01939301508414,3.38981788433784));
#29237=CARTESIAN_POINT('Ctrl Pts',(47.5074526458959,1.03306910336338,4.42044881162439));
#29238=CARTESIAN_POINT('Ctrl Pts',(47.6263616448908,-1.20429241117321,4.37690292980164));
#29239=CARTESIAN_POINT('Ctrl Pts',(47.7452706438858,-3.14900875898673,3.26976196447697));
#29240=CARTESIAN_POINT('Ctrl Pts',(47.8641796428807,-4.32851045898203,1.36806311075136));
#29241=CARTESIAN_POINT('Ctrl Pts',(47.9830886418757,-4.45617653070388,-0.866077476741777));
#29242=CARTESIAN_POINT('Ctrl Pts',(48.1019976408706,-3.50098389495883,-2.88975971938056));
#29243=CARTESIAN_POINT('Ctrl Pts',(48.2209066398657,-1.69504603643448,-4.21122528522083));
#29244=CARTESIAN_POINT('Ctrl Pts',(48.3398156388606,0.522790979913529,-4.50935572558172));
#29245=CARTESIAN_POINT('Ctrl Pts',(48.4587246378556,2.61358887182741,-3.7117048209112));
#29246=CARTESIAN_POINT('Ctrl Pts',(48.5776336368505,4.06928008695307,-2.01210313911658));
#29247=CARTESIAN_POINT('Ctrl Pts',(48.6965426358455,4.53612910857099,0.176443132171203));
#29248=CARTESIAN_POINT('Ctrl Pts',(48.8154516348404,3.90069080616449,2.32211341308284));
#29249=CARTESIAN_POINT('Ctrl Pts',(48.9343606338354,2.31737780097448,3.90350606456131));
#29250=CARTESIAN_POINT('Ctrl Pts',(49.0532696328304,0.17093792839381,4.53633990053105));
#29251=CARTESIAN_POINT('Ctrl Pts',(49.1721786318254,-2.01704016039613,4.06683518966148));
#29252=CARTESIAN_POINT('Ctrl Pts',(49.2910876308203,-3.71487395486803,2.60908239960943));
#29253=CARTESIAN_POINT('Ctrl Pts',(49.4099966298152,-4.50998686711097,0.51731801342058));
#29254=CARTESIAN_POINT('Ctrl Pts',(49.5289056288102,-4.2091650658221,-1.70015555675947));
#29255=CARTESIAN_POINT('Ctrl Pts',(49.6478146278052,-2.88550877598391,-3.50448834670629));
#29256=CARTESIAN_POINT('Ctrl Pts',(49.7667236268002,-0.860668796033026,
-4.45722432598666));
#29257=CARTESIAN_POINT('Ctrl Pts',(49.885632625795,1.37331520985932,-4.32684698165025));
#29258=CARTESIAN_POINT('Ctrl Pts',(50.0045416247901,3.27358121273658,-3.14503823706665));
#29259=CARTESIAN_POINT('Ctrl Pts',(50.123450623785,4.37836124310941,-1.19897968821326));
#29260=CARTESIAN_POINT('Ctrl Pts',(50.24235962278,4.41919181745465,1.03843302589838));
#29261=CARTESIAN_POINT('Ctrl Pts',(50.3612686217749,3.38615103414948,3.02350469556191));
#29262=CARTESIAN_POINT('Ctrl Pts',(50.4801776207699,1.53026961516699,4.27385942290892));
#29263=CARTESIAN_POINT('Ctrl Pts',(50.5990866197649,-0.697470003765305,
4.48565882330066));
#29264=CARTESIAN_POINT('Ctrl Pts',(50.7179956187599,-2.7557231866993,3.60743525994027));
#29265=CARTESIAN_POINT('Ctrl Pts',(50.8369046177548,-4.14433081039863,1.85259862051291));
#29266=CARTESIAN_POINT('Ctrl Pts',(50.9558136167497,-4.52585877288994,-0.352422760715905));
#29267=CARTESIAN_POINT('Ctrl Pts',(51.0747226157447,-3.807595141598,-2.47180473372834));
#29268=CARTESIAN_POINT('Ctrl Pts',(51.1936316147397,-2.16407917594154,-3.99053394305953));
#29269=CARTESIAN_POINT('Ctrl Pts',(51.3125406137346,0.00531174023636265,
-4.53955617234671));
#29270=CARTESIAN_POINT('Ctrl Pts',(51.4314496127296,2.17341205843241,-3.9854587690482));
#29271=CARTESIAN_POINT('Ctrl Pts',(51.5503586117245,3.81336910936164,-2.46288695372717));
#29272=CARTESIAN_POINT('Ctrl Pts',(51.6692676107196,4.5266714366548,-0.341831178824977));
#29273=CARTESIAN_POINT('Ctrl Pts',(51.7881766097145,4.13998336627106,1.86229393683439));
#29274=CARTESIAN_POINT('Ctrl Pts',(51.9070856087095,2.74727468452559,3.61387084890872));
#29275=CARTESIAN_POINT('Ctrl Pts',(52.0259946077044,0.686968245402081,4.48728580129519));
#29276=CARTESIAN_POINT('Ctrl Pts',(52.1449036066994,-1.54026231798197,4.27025252648642));
#29277=CARTESIAN_POINT('Ctrl Pts',(52.2638126056943,-3.39322711737773,3.01560009701075));
#29278=CARTESIAN_POINT('Ctrl Pts',(52.3827216046892,-4.42159051474481,1.02803234388526));
#29279=CARTESIAN_POINT('Ctrl Pts',(52.5016306036843,-4.37558204264944,-1.20910982083371));
#29280=CARTESIAN_POINT('Ctrl Pts',(52.6205396026792,-3.26613430286741,-3.15293004541843));
#29281=CARTESIAN_POINT('Ctrl Pts',(52.6998122686759,-1.99759989989662,-3.93718287761649));
#29282=CARTESIAN_POINT('Ctrl Pts',(52.7394486016742,-1.30786439202407,-4.15432535756649));
#29283=CARTESIAN_POINT('Ctrl Pts',(29.8355513983258,-2.04298847651431,4.16621468233146));
#29284=CARTESIAN_POINT('Ctrl Pts',(29.8751877313241,-2.73469794856857,3.82702081253504));
#29285=CARTESIAN_POINT('Ctrl Pts',(29.9544603973208,-3.9452116126247,2.79778531791265));
#29286=CARTESIAN_POINT('Ctrl Pts',(30.0733693963157,-4.80242447513901,0.572672373630749));
#29287=CARTESIAN_POINT('Ctrl Pts',(30.1922783953107,-4.49254491555146,-1.79105432277335));
#29288=CARTESIAN_POINT('Ctrl Pts',(30.3111873943056,-3.09101751001259,-3.71981687341617));
#29289=CARTESIAN_POINT('Ctrl Pts',(30.4300963933007,-0.938343063236198,
-4.74452522688149));
#29290=CARTESIAN_POINT('Ctrl Pts',(30.5490053922956,1.44233817327656,-4.61637182153812));
#29291=CARTESIAN_POINT('Ctrl Pts',(30.6679143912906,3.47253483004752,-3.36639880583222));
#29292=CARTESIAN_POINT('Ctrl Pts',(30.7868233902855,4.65889636729902,-1.29840160142966));
#29293=CARTESIAN_POINT('Ctrl Pts',(30.9057323892805,4.71313945974424,1.08511779798324));
#29294=CARTESIAN_POINT('Ctrl Pts',(31.0246413882754,3.62208063165091,3.20494749580355));
#29295=CARTESIAN_POINT('Ctrl Pts',(31.1435503872704,1.65085024787275,4.54597142695528));
#29296=CARTESIAN_POINT('Ctrl Pts',(31.2624593862653,-0.721539833275788,
4.78231528490551));
#29297=CARTESIAN_POINT('Ctrl Pts',(31.3813683852603,-2.91859437322766,3.85654867198333));
#29298=CARTESIAN_POINT('Ctrl Pts',(31.5002773842553,-4.40642541359019,1.99363370889056));
#29299=CARTESIAN_POINT('Ctrl Pts',(31.6191863832502,-4.8234873307716,-0.353737607790146));
#29300=CARTESIAN_POINT('Ctrl Pts',(31.7380953822452,-4.0684333844855,-2.6151501319167));
#29301=CARTESIAN_POINT('Ctrl Pts',(31.8570043812401,-2.32474298875354,-4.24107655716586));
#29302=CARTESIAN_POINT('Ctrl Pts',(31.9759133802352,-0.0161359751592512,
-4.83641396214568));
#29303=CARTESIAN_POINT('Ctrl Pts',(32.09482237923,2.29639211021845,-4.25649428903554));
#29304=CARTESIAN_POINT('Ctrl Pts',(32.2137313782251,4.05089288707086,-2.64223904734728));
#29305=CARTESIAN_POINT('Ctrl Pts',(32.33264037722,4.82101959260105,-0.385915083911942));
#29306=CARTESIAN_POINT('Ctrl Pts',(32.451549376215,4.41963008695579,1.96418692027359));
#29307=CARTESIAN_POINT('Ctrl Pts',(32.5704583752099,2.94426272382771,3.83698806065463));
#29308=CARTESIAN_POINT('Ctrl Pts',(32.6893673742049,0.753434358242411,4.77739437680209));
#29309=CARTESIAN_POINT('Ctrl Pts',(32.8082763731998,-1.62047987694377,4.55688548600226));
#29310=CARTESIAN_POINT('Ctrl Pts',(32.9271853721948,-3.60061466176965,3.22904543501556));
#29311=CARTESIAN_POINT('Ctrl Pts',(33.0460943711898,-4.70579377284853,1.11654168368553));
#29312=CARTESIAN_POINT('Ctrl Pts',(33.1650033701848,-4.66745674910901,-1.26728365380071));
#29313=CARTESIAN_POINT('Ctrl Pts',(33.2839123691797,-3.49491955450991,-3.34315684219));
#29314=CARTESIAN_POINT('Ctrl Pts',(33.4028213681747,-1.47311078249056,-4.60663705825629));
#29315=CARTESIAN_POINT('Ctrl Pts',(33.5217303671696,0.906666491650291,-4.7506963949406));
#29316=CARTESIAN_POINT('Ctrl Pts',(33.6406393661646,3.06612221917194,-3.74032818093363));
#29317=CARTESIAN_POINT('Ctrl Pts',(33.7595483651595,4.48050487332878,-1.82105366314733));
#29318=CARTESIAN_POINT('Ctrl Pts',(33.8784573641545,4.80611699011961,0.540740086611801));
#29319=CARTESIAN_POINT('Ctrl Pts',(33.9973663631495,3.96383425445189,2.77113304754918));
#29320=CARTESIAN_POINT('Ctrl Pts',(34.1162753621445,2.15833284739307,4.32813582086438));
#29321=CARTESIAN_POINT('Ctrl Pts',(34.2351843611394,-0.171647224572306,
4.8333940036254));
#29322=CARTESIAN_POINT('Ctrl Pts',(34.3540933601344,-2.45991672011416,4.16412897183651));
#29323=CARTESIAN_POINT('Ctrl Pts',(34.4730023591293,-4.150422141081,2.48297330126805));
#29324=CARTESIAN_POINT('Ctrl Pts',(34.5919113581243,-4.83236770716634,0.198450766492061));
#29325=CARTESIAN_POINT('Ctrl Pts',(34.7108203571192,-4.34003945054015,-2.13429565237352));
#29326=CARTESIAN_POINT('Ctrl Pts',(34.8297293561142,-2.7930740004846,-3.94840448685318));
#29327=CARTESIAN_POINT('Ctrl Pts',(34.9486383551091,-0.567386672786905,
-4.80304411051253));
#29328=CARTESIAN_POINT('Ctrl Pts',(35.0675473541042,1.79617661087767,-4.4905355968438));
#29329=CARTESIAN_POINT('Ctrl Pts',(35.1864563530991,3.72326582987361,-3.08681906241375));
#29330=CARTESIAN_POINT('Ctrl Pts',(35.3053653520941,4.74559492630417,-0.933000085434894));
#29331=CARTESIAN_POINT('Ctrl Pts',(35.424274351089,4.61473613786257,1.4475395476085));
#29332=CARTESIAN_POINT('Ctrl Pts',(35.543183350084,3.36248837950119,3.47632453342676));
#29333=CARTESIAN_POINT('Ctrl Pts',(35.662092349079,1.29315005136293,4.66035656453939));
#29334=CARTESIAN_POINT('Ctrl Pts',(35.7810013480739,-1.09042600580856,4.71191378208915));
#29335=CARTESIAN_POINT('Ctrl Pts',(35.8999103470689,-3.20902663233849,3.61846769184522));
#29336=CARTESIAN_POINT('Ctrl Pts',(36.0188193460638,-4.54782816263016,1.64572761026036));
#29337=CARTESIAN_POINT('Ctrl Pts',(36.1377283450588,-4.78149947825562,-0.726927165145562));
#29338=CARTESIAN_POINT('Ctrl Pts',(36.2566373440538,-3.85325803995349,-2.92293736530895));
#29339=CARTESIAN_POINT('Ctrl Pts',(36.3755463430487,-1.9886681441944,-4.40866866256147));
#29340=CARTESIAN_POINT('Ctrl Pts',(36.4944553420437,0.359171596216373,-4.82308574757461));
#29341=CARTESIAN_POINT('Ctrl Pts',(36.6133643410386,2.61973200921313,-4.06548454232559));
#29342=CARTESIAN_POINT('Ctrl Pts',(36.7322733400336,4.24369295226976,-2.31996346756645));
#29343=CARTESIAN_POINT('Ctrl Pts',(36.8511823390285,4.83642906984657,-0.0106872039015828));
#29344=CARTESIAN_POINT('Ctrl Pts',(36.9700913380235,4.25390444646255,2.3011860690411));
#29345=CARTESIAN_POINT('Ctrl Pts',(37.0890003370185,2.63767358661105,4.05386709383689));
#29346=CARTESIAN_POINT('Ctrl Pts',(37.2079093360135,0.380483422066699,4.82145130945858));
#29347=CARTESIAN_POINT('Ctrl Pts',(37.3268183350084,-1.96916488093114,4.41741440616232));
#29348=CARTESIAN_POINT('Ctrl Pts',(37.4457273340034,-3.84030266642664,2.93993805956863));
#29349=CARTESIAN_POINT('Ctrl Pts',(37.5646363329983,-4.77824017295507,0.748051611629016));
#29350=CARTESIAN_POINT('Ctrl Pts',(37.6835453319933,-4.55505694242569,-1.62561268920943));
#29351=CARTESIAN_POINT('Ctrl Pts',(37.8024543309882,-3.22498689113141,-3.60425025702862));
#29352=CARTESIAN_POINT('Ctrl Pts',(37.9213633299832,-1.11123937261475,-4.70704869562491));
#29353=CARTESIAN_POINT('Ctrl Pts',(38.0402723289781,1.27254126091167,-4.66602604989169));
#29354=CARTESIAN_POINT('Ctrl Pts',(38.1591813279731,3.34709213809732,-3.49115089786058));
#29355=CARTESIAN_POINT('Ctrl Pts',(38.2780903269681,4.60829375817302,-1.46791995430425));
#29356=CARTESIAN_POINT('Ctrl Pts',(38.396999325963,4.74967191984029,0.912018102494755));
#29357=CARTESIAN_POINT('Ctrl Pts',(38.515908324958,3.73687147615934,3.07033417888194));
#29358=CARTESIAN_POINT('Ctrl Pts',(38.634817323953,1.81600472180213,4.48255363434665));
#29359=CARTESIAN_POINT('Ctrl Pts',(38.7537263229479,-0.546154378463043,
4.80550476770034));
#29360=CARTESIAN_POINT('Ctrl Pts',(38.8726353219429,-2.77559697650641,3.9607096844851));
#29361=CARTESIAN_POINT('Ctrl Pts',(38.9915443209379,-4.33056470620339,2.15345547569111));
#29362=CARTESIAN_POINT('Ctrl Pts',(39.1104533199328,-4.83319749856621,-0.17709272655029));
#29363=CARTESIAN_POINT('Ctrl Pts',(39.2293623189278,-4.16135507364998,-2.46460601151995));
#29364=CARTESIAN_POINT('Ctrl Pts',(39.3482713179228,-2.47829558082605,-4.15321785953489));
#29365=CARTESIAN_POINT('Ctrl Pts',(39.4671803169177,-0.193006898275515,
-4.83258621084879));
#29366=CARTESIAN_POINT('Ctrl Pts',(39.5860893159127,2.13918475471825,-4.33763617745607));
#29367=CARTESIAN_POINT('Ctrl Pts',(39.7049983149076,3.95154686023701,-2.78861592032275));
#29368=CARTESIAN_POINT('Ctrl Pts',(39.8239073139026,4.80368393985005,-0.561991087425867));
#29369=CARTESIAN_POINT('Ctrl Pts',(39.9428163128975,4.48850186438168,1.80126636791584));
#29370=CARTESIAN_POINT('Ctrl Pts',(40.0617253118926,3.08263697266631,3.72667764760597));
#29371=CARTESIAN_POINT('Ctrl Pts',(40.1806343108874,0.927624029768742,4.74676968017454));
#29372=CARTESIAN_POINT('Ctrl Pts',(40.2995433098825,-1.45267973830484,4.612849709944));
#29373=CARTESIAN_POINT('Ctrl Pts',(40.4184523088774,-3.48022609014271,3.35907396628158));
#29374=CARTESIAN_POINT('Ctrl Pts',(40.5373613078724,-4.66157992956727,1.28689284996747));
#29375=CARTESIAN_POINT('Ctrl Pts',(40.6562703068673,-4.71114240206199,-1.09372738803408));
#29376=CARTESIAN_POINT('Ctrl Pts',(40.7751793058623,-3.61393126835275,-3.21709376641143));
#29377=CARTESIAN_POINT('Ctrl Pts',(40.8940883048572,-1.64244639784748,-4.5418482715989));
#29378=CARTESIAN_POINT('Ctrl Pts',(41.0526336368505,1.52894407634182,-4.87830053372444));
#29379=CARTESIAN_POINT('Ctrl Pts',(41.2508153018422,4.99877843246716,-2.25841953589028));
#29380=CARTESIAN_POINT('Ctrl Pts',(41.488633299832,4.60241792036846,2.98429118942186));
#29381=CARTESIAN_POINT('Ctrl Pts',(41.6868149648237,0.778136914097525,5.0527209529951));
#29382=CARTESIAN_POINT('Ctrl Pts',(41.8453602968169,-2.30662225456386,4.24328995789574));
#29383=CARTESIAN_POINT('Ctrl Pts',(41.9642692958119,-4.05652806066456,2.63719009692172));
#29384=CARTESIAN_POINT('Ctrl Pts',(42.0831782948068,-4.8220301182078,0.372998486510622));
#29385=CARTESIAN_POINT('Ctrl Pts',(42.2020872938019,-4.41511642611984,-1.97311114508245));
#29386=CARTESIAN_POINT('Ctrl Pts',(42.3209962927967,-2.93564809227475,-3.84412822728174));
#29387=CARTESIAN_POINT('Ctrl Pts',(42.4399052917918,-0.742648657028073,
-4.77882138616062));
#29388=CARTESIAN_POINT('Ctrl Pts',(42.5588142907866,1.63073378640869,-4.55335217780196));
#29389=CARTESIAN_POINT('Ctrl Pts',(42.6777232897817,3.60788611488371,-3.22085932267223));
#29390=CARTESIAN_POINT('Ctrl Pts',(42.7966322887766,4.70829521929217,-1.10596819245989));
#29391=CARTESIAN_POINT('Ctrl Pts',(42.9155412877716,4.66459064421329,1.27781356161113));
#29392=CARTESIAN_POINT('Ctrl Pts',(43.0344502867665,3.48737719917427,3.35101501196365));
#29393=CARTESIAN_POINT('Ctrl Pts',(43.1533592857615,1.46272757210891,4.60994870606898));
#29394=CARTESIAN_POINT('Ctrl Pts',(43.2722682847565,-0.917368716687352,
4.74863936151306));
#29395=CARTESIAN_POINT('Ctrl Pts',(43.3911772837514,-3.07454214894444,3.73341106082168));
#29396=CARTESIAN_POINT('Ctrl Pts',(43.5100862827464,-4.48459677614081,1.810952952575));
#29397=CARTESIAN_POINT('Ctrl Pts',(43.6289952817414,-4.80488636303764,-0.551567704129478));
#29398=CARTESIAN_POINT('Ctrl Pts',(43.7479042807363,-3.95758022389326,-2.78005754110368));
#29399=CARTESIAN_POINT('Ctrl Pts',(43.8668132797313,-2.14857511271005,-4.33298797203599));
#29400=CARTESIAN_POINT('Ctrl Pts',(43.9857222787262,0.182537496183628,-4.83299500723848));
#29401=CARTESIAN_POINT('Ctrl Pts',(44.1046312777212,2.46929318387108,-4.15857564635895));
#29402=CARTESIAN_POINT('Ctrl Pts',(44.2235402767161,4.15600629469078,-2.47361518386237));
#29403=CARTESIAN_POINT('Ctrl Pts',(44.3424492757112,4.83280259410293,-0.187561861340418));
#29404=CARTESIAN_POINT('Ctrl Pts',(44.461358274706,4.33521939121839,2.14406930481855));
#29405=CARTESIAN_POINT('Ctrl Pts',(44.580267273701,2.78417027841813,3.95468788064478));
#29406=CARTESIAN_POINT('Ctrl Pts',(44.699176272696,0.556562907717911,4.80431036557206));
#29407=CARTESIAN_POINT('Ctrl Pts',(44.818085271691,-1.80629022490289,4.48647701316453));
#29408=CARTESIAN_POINT('Ctrl Pts',(44.9369942706859,-3.73021166700226,3.07842188184474));
#29409=CARTESIAN_POINT('Ctrl Pts',(45.0559032696809,-4.74768513589875,0.922304838123059));
#29410=CARTESIAN_POINT('Ctrl Pts',(45.1748122686758,-4.61146279534857,-1.45793389809636));
#29411=CARTESIAN_POINT('Ctrl Pts',(45.2937212676708,-3.3546469128365,-3.48389214156527));
#29412=CARTESIAN_POINT('Ctrl Pts',(45.4126302666657,-1.28264595069628,-4.66325848835612));
#29413=CARTESIAN_POINT('Ctrl Pts',(45.5315392656608,1.10104022560684,-4.70944484897563));
#29414=CARTESIAN_POINT('Ctrl Pts',(45.6504482646557,3.21717169725219,-3.61122785689281));
#29415=CARTESIAN_POINT('Ctrl Pts',(45.7693572636507,4.55152480760976,-1.63547616604331));
#29416=CARTESIAN_POINT('Ctrl Pts',(45.8882662626456,4.77984941209146,0.737699099710084));
#29417=CARTESIAN_POINT('Ctrl Pts',(46.0071752616406,3.84666223161579,2.93161219124352));
#29418=CARTESIAN_POINT('Ctrl Pts',(46.1260842606355,1.97872938666984,4.41313838195828));
#29419=CARTESIAN_POINT('Ctrl Pts',(46.2449932596306,-0.370038167429234,
4.82226421078643));
#29420=CARTESIAN_POINT('Ctrl Pts',(46.3639022586254,-2.62888579826341,4.05957138423185));
#29421=CARTESIAN_POINT('Ctrl Pts',(46.4828112576205,-4.24890957237392,2.31039559594774));
#29422=CARTESIAN_POINT('Ctrl Pts',(46.6017202566154,-4.83644087317617,-0.000210371667774191));
#29423=CARTESIAN_POINT('Ctrl Pts',(46.7206292556104,-4.24870856478734,-2.31076521859925));
#29424=CARTESIAN_POINT('Ctrl Pts',(46.8395382546053,-2.62853262828611,-4.05980006724723));
#29425=CARTESIAN_POINT('Ctrl Pts',(46.9584472536003,-0.369618655984746,
-4.82229638379199));
#29426=CARTESIAN_POINT('Ctrl Pts',(47.0773562525952,1.97911329756526,-4.41296622685759));
#29427=CARTESIAN_POINT('Ctrl Pts',(47.1962652515902,3.84691725094163,-2.9312775420272));
#29428=CARTESIAN_POINT('Ctrl Pts',(47.3151742505852,4.77991356970463,-0.737283276725339));
#29429=CARTESIAN_POINT('Ctrl Pts',(47.4340832495801,4.55138251309761,1.6358721170845));
#29430=CARTESIAN_POINT('Ctrl Pts',(47.552992248575,3.21685752843096,3.61150771918909));
#29431=CARTESIAN_POINT('Ctrl Pts',(47.6719012475701,1.10063052605007,4.70954061550722));
#29432=CARTESIAN_POINT('Ctrl Pts',(47.7908102465649,-1.28305162327693,4.66314688767058));
#29433=CARTESIAN_POINT('Ctrl Pts',(47.9097192455601,-3.35494997929547,3.48360029285948));
#29434=CARTESIAN_POINT('Ctrl Pts',(48.0286282445548,-4.61158960999993,1.45753272104811));
#29435=CARTESIAN_POINT('Ctrl Pts',(48.1475372435499,-4.7476048825703,-0.922717856649593));
#29436=CARTESIAN_POINT('Ctrl Pts',(48.2664462425448,-3.72994384737292,-3.07874637789965));
#29437=CARTESIAN_POINT('Ctrl Pts',(48.3853552415398,-1.80589991965302,-4.48663413308713));
#29438=CARTESIAN_POINT('Ctrl Pts',(48.5042642405348,0.556980853810344,-4.80426193004442));
#29439=CARTESIAN_POINT('Ctrl Pts',(48.6231732395297,2.7845143035568,-3.95444565739282));
#29440=CARTESIAN_POINT('Ctrl Pts',(48.7420822385247,4.33540589701746,-2.14369215889122));
#29441=CARTESIAN_POINT('Ctrl Pts',(48.8609912375196,4.83278625867614,0.187982291549743));
#29442=CARTESIAN_POINT('Ctrl Pts',(48.9799002365146,4.15579108887287,2.47397671566045));
#29443=CARTESIAN_POINT('Ctrl Pts',(49.0988092355096,2.46893140046422,4.1587904616352));
#29444=CARTESIAN_POINT('Ctrl Pts',(49.2177182345045,0.182117054355301,4.8330108361658));
#29445=CARTESIAN_POINT('Ctrl Pts',(49.3366272334995,-2.14895205516562,4.33280110651177));
#29446=CARTESIAN_POINT('Ctrl Pts',(49.4555362324944,-3.95782204873261,2.77971311371218));
#29447=CARTESIAN_POINT('Ctrl Pts',(49.5744452314894,-4.80493434743749,0.551149962178289));
#29448=CARTESIAN_POINT('Ctrl Pts',(49.6933542304843,-4.48443917792565,-1.81134359619393));
#29449=CARTESIAN_POINT('Ctrl Pts',(49.8122632294794,-3.07421742814054,-3.73367748586597));
#29450=CARTESIAN_POINT('Ctrl Pts',(49.9311722284743,-0.91695545501133,-4.74872120234939));
#29451=CARTESIAN_POINT('Ctrl Pts',(50.0500812274693,1.46312830084543,-4.60981734333861));
#29452=CARTESIAN_POINT('Ctrl Pts',(50.1689902264642,3.48766931516144,-3.35071979022551));
#29453=CARTESIAN_POINT('Ctrl Pts',(50.2878992254592,4.66470057283824,-1.2773914549038));
#29454=CARTESIAN_POINT('Ctrl Pts',(50.4068082244542,4.70820141549651,1.1063452423862));
#29455=CARTESIAN_POINT('Ctrl Pts',(50.5257172234491,3.60760106160095,3.2212381076511));
#29456=CARTESIAN_POINT('Ctrl Pts',(50.6446262224441,1.63034732725642,4.55336446476378));
#29457=CARTESIAN_POINT('Ctrl Pts',(50.763535221439,-0.743083666570843,4.77901528009773));
#29458=CARTESIAN_POINT('Ctrl Pts',(50.882444220434,-2.93594402421914,3.84335699801001));
#29459=CARTESIAN_POINT('Ctrl Pts',(51.001353219429,-4.41536484357523,1.97375624497553));
#29460=CARTESIAN_POINT('Ctrl Pts',(51.1202622184239,-4.82184425593253,-0.375470766917604));
#29461=CARTESIAN_POINT('Ctrl Pts',(51.2391712174189,-4.05660708469425,-2.6334576607887));
#29462=CARTESIAN_POINT('Ctrl Pts',(51.3580802164138,-2.30560723776937,-4.25150985415276));
#29463=CARTESIAN_POINT('Ctrl Pts',(51.4769892154088,0.00565912138068442,
-4.83643744812126));
#29464=CARTESIAN_POINT('Ctrl Pts',(51.5958982144037,2.31555047906077,-4.2461027701313));
#29465=CARTESIAN_POINT('Ctrl Pts',(51.7148072133987,4.06275866270233,-2.62395666916879));
#29466=CARTESIAN_POINT('Ctrl Pts',(51.8337162123937,4.82271006688757,-0.364186508865252));
#29467=CARTESIAN_POINT('Ctrl Pts',(51.9526252113887,4.41073308205851,1.98408562281516));
#29468=CARTESIAN_POINT('Ctrl Pts',(52.0715342103836,2.92694300060758,3.85021346641923));
#29469=CARTESIAN_POINT('Ctrl Pts',(52.1904432093786,0.731895106392164,4.78074866041095));
#29470=CARTESIAN_POINT('Ctrl Pts',(52.3093522083735,-1.64099354029295,4.54952168184252));
#29471=CARTESIAN_POINT('Ctrl Pts',(52.4282612073685,-3.61513991179064,3.21281655827632));
#29472=CARTESIAN_POINT('Ctrl Pts',(52.5471702063634,-4.71075698457868,1.09526436882405));
#29473=CARTESIAN_POINT('Ctrl Pts',(52.6660792053584,-4.66173961615656,-1.28818408548258));
#29474=CARTESIAN_POINT('Ctrl Pts',(52.7849882043534,-3.47973538673397,-3.35912771293794));
#29475=CARTESIAN_POINT('Ctrl Pts',(52.86426087035,-2.12824042603024,-4.1946696959942));
#29476=CARTESIAN_POINT('Ctrl Pts',(52.9038972033484,-1.39339708167545,-4.42601302158306));
#29477=CARTESIAN_POINT('Ctrl Pts',(30.,-2.16839587231052,4.42195480991684));
#29478=CARTESIAN_POINT('Ctrl Pts',(30.0396363329983,-2.90256543874863,4.06193976546858));
#29479=CARTESIAN_POINT('Ctrl Pts',(30.118908998995,-4.1873856238303,2.96952538142736));
#29480=CARTESIAN_POINT('Ctrl Pts',(30.2378179979899,-5.0972178887381,0.607825460320724));
#29481=CARTESIAN_POINT('Ctrl Pts',(30.3567269969849,-4.7683165925989,-1.90099691957731));
#29482=CARTESIAN_POINT('Ctrl Pts',(30.4756359959799,-3.28075742325608,-3.94815518873056));
#29483=CARTESIAN_POINT('Ctrl Pts',(30.5945449949748,-0.995942585346445,
-5.03576453627197));
#29484=CARTESIAN_POINT('Ctrl Pts',(30.7134539939698,1.53087507705621,-4.89974452521287));
#29485=CARTESIAN_POINT('Ctrl Pts',(30.8323629929647,3.68569391285887,-3.57304280422193));
#29486=CARTESIAN_POINT('Ctrl Pts',(30.9512719919597,4.94487940999554,-1.37810306103397));
#29487=CARTESIAN_POINT('Ctrl Pts',(31.0701809909546,5.00245217612307,1.15172698288151));
#29488=CARTESIAN_POINT('Ctrl Pts',(31.1890899899496,3.8444194772201,3.40168092026129));
#29489=CARTESIAN_POINT('Ctrl Pts',(31.3079989889446,1.75218651717396,4.82502265243806));
#29490=CARTESIAN_POINT('Ctrl Pts',(31.4269079879395,-0.765831043184473,
5.07587431015258));
#29491=CARTESIAN_POINT('Ctrl Pts',(31.5458169869345,-3.0977502147508,4.09328017158535));
#29492=CARTESIAN_POINT('Ctrl Pts',(31.6647259859294,-4.6769107062099,2.11601149734983));
#29493=CARTESIAN_POINT('Ctrl Pts',(31.7836349849244,-5.11957367279555,-0.375451539463316));
#29494=CARTESIAN_POINT('Ctrl Pts',(31.9025439839194,-4.31817127659016,-2.77567926432736));
#29495=CARTESIAN_POINT('Ctrl Pts',(32.0214529829144,-2.46744568505685,-4.5014120277379));
#29496=CARTESIAN_POINT('Ctrl Pts',(32.1403619819093,-0.0171264705275148,
-5.1332937962503));
#29497=CARTESIAN_POINT('Ctrl Pts',(32.2592709809043,2.43735450799018,-4.51777616612193));
#29498=CARTESIAN_POINT('Ctrl Pts',(32.3781799798992,4.29955406820673,-2.80443101358115));
#29499=CARTESIAN_POINT('Ctrl Pts',(32.4970889788942,5.11695445427107,-0.409604207090211));
#29500=CARTESIAN_POINT('Ctrl Pts',(32.6159979778891,4.69092593906626,2.08475713853971));
#29501=CARTESIAN_POINT('Ctrl Pts',(32.7349069768841,3.12499419881144,4.07251884603082));
#29502=CARTESIAN_POINT('Ctrl Pts',(32.8538159758791,0.799683390900607,5.07065133560223));
#29503=CARTESIAN_POINT('Ctrl Pts',(32.9727249748741,-1.71995188260795,4.83660666324366));
#29504=CARTESIAN_POINT('Ctrl Pts',(33.091633973869,-3.82163583403228,3.42725809434683));
#29505=CARTESIAN_POINT('Ctrl Pts',(33.210542972864,-4.99465557945741,1.18507980147653));
#29506=CARTESIAN_POINT('Ctrl Pts',(33.3294519718589,-4.95396526475957,-1.34507496030352));
#29507=CARTESIAN_POINT('Ctrl Pts',(33.4483609708539,-3.70945270772488,-3.54837414915822));
#29508=CARTESIAN_POINT('Ctrl Pts',(33.5672699698489,-1.56353664101852,-4.88941220040492));
#29509=CARTESIAN_POINT('Ctrl Pts',(33.6861789688438,0.962321569924411,-5.0423145170969));
#29510=CARTESIAN_POINT('Ctrl Pts',(33.8050879678388,3.2543339526788,-3.9699255682838));
#29511=CARTESIAN_POINT('Ctrl Pts',(33.9239969668337,4.75553748094053,-1.93283774814137));
#29512=CARTESIAN_POINT('Ctrl Pts',(34.0429059658287,5.10113706612673,0.573933032555513));
#29513=CARTESIAN_POINT('Ctrl Pts',(34.1618149648236,4.20715140329205,2.94123708038784));
#29514=CARTESIAN_POINT('Ctrl Pts',(34.2807239638186,2.29082057542709,4.59381536247054));
#29515=CARTESIAN_POINT('Ctrl Pts',(34.3996329628136,-0.182183667472828,
5.13008845972237));
#29516=CARTESIAN_POINT('Ctrl Pts',(34.5185419618085,-2.61091695985679,4.41974106956536));
#29517=CARTESIAN_POINT('Ctrl Pts',(34.6374509608035,-4.40519285474456,2.63538885285986));
#29518=CARTESIAN_POINT('Ctrl Pts',(34.7563599597985,-5.1289991647845,0.210632525765634));
#29519=CARTESIAN_POINT('Ctrl Pts',(34.8752689587934,-4.60644968799474,-2.26530787427308));
#29520=CARTESIAN_POINT('Ctrl Pts',(34.9941779577884,-2.96452486312706,-4.19077449037431));
#29521=CARTESIAN_POINT('Ctrl Pts',(35.1130869567833,-0.602215300486822,
-5.09787555998869));
#29522=CARTESIAN_POINT('Ctrl Pts',(35.2319959557783,1.90643363569679,-4.76618393329028));
#29523=CARTESIAN_POINT('Ctrl Pts',(35.3509049547733,3.95181585692917,-3.27630125693498));
#29524=CARTESIAN_POINT('Ctrl Pts',(35.4698139537682,5.03689989843353,-0.990271632649752));
#29525=CARTESIAN_POINT('Ctrl Pts',(35.5887229527632,4.89800843625729,1.53639573405519));
#29526=CARTESIAN_POINT('Ctrl Pts',(35.7076319517581,3.56889233914948,3.68971624448692));
#29527=CARTESIAN_POINT('Ctrl Pts',(35.8265409507531,1.37252914829839,4.94642924040584));
#29528=CARTESIAN_POINT('Ctrl Pts',(35.9454499497481,-1.15736103127196,5.00115126111614));
#29529=CARTESIAN_POINT('Ctrl Pts',(36.064358948743,-3.40601045169361,3.84058475967195));
#29530=CARTESIAN_POINT('Ctrl Pts',(36.183267947738,-4.82699336251288,1.7467494300921));
#29531=CARTESIAN_POINT('Ctrl Pts',(36.3021769467329,-5.07500842579123,-0.771549072592608));
#29532=CARTESIAN_POINT('Ctrl Pts',(36.421085945728,-4.08978754644683,-3.10235979831467));
#29533=CARTESIAN_POINT('Ctrl Pts',(36.5399949447229,-2.11074112499353,-4.67929165542513));
#29534=CARTESIAN_POINT('Ctrl Pts',(36.6589039437178,0.381219089407465,-5.11914743869939));
#29535=CARTESIAN_POINT('Ctrl Pts',(36.7778129427128,2.78054239690555,-4.31504142184985));
#29536=CARTESIAN_POINT('Ctrl Pts',(36.8967219417078,4.50418902839594,-2.46237277635822));
#29537=CARTESIAN_POINT('Ctrl Pts',(37.0156309407027,5.13330983132668,-0.0113432303183229));
#29538=CARTESIAN_POINT('Ctrl Pts',(37.1345399396977,4.51502734790305,2.44244274056837));
#29539=CARTESIAN_POINT('Ctrl Pts',(37.2534489386926,2.79958530528203,4.3027108445415));
#29540=CARTESIAN_POINT('Ctrl Pts',(37.3723579376876,0.403839126542568,5.11741267176111));
#29541=CARTESIAN_POINT('Ctrl Pts',(37.4912669366826,-2.09004066777468,4.68857425028185));
#29542=CARTESIAN_POINT('Ctrl Pts',(37.6101759356776,-4.07603691652264,3.12040406811011));
#29543=CARTESIAN_POINT('Ctrl Pts',(37.7290849346725,-5.071549050351,0.793970228211562));
#29544=CARTESIAN_POINT('Ctrl Pts',(37.8479939336675,-4.83466587581909,-1.72539976890694));
#29545=CARTESIAN_POINT('Ctrl Pts',(37.9669029326624,-3.42295041963053,-3.82549459772262));
#29546=CARTESIAN_POINT('Ctrl Pts',(38.0858119316574,-1.17945201180872,-4.99598753477663));
#29547=CARTESIAN_POINT('Ctrl Pts',(38.2047209306523,1.35065530189071,-4.95244674308752));
#29548=CARTESIAN_POINT('Ctrl Pts',(38.3236299296473,3.55255101040822,-3.7054527147653));
#29549=CARTESIAN_POINT('Ctrl Pts',(38.4425389286423,4.89117059566871,-1.55802717753281));
#29550=CARTESIAN_POINT('Ctrl Pts',(38.5614479276372,5.0412271553206,0.968001685597478));
#29551=CARTESIAN_POINT('Ctrl Pts',(38.6803569266322,3.96625667614341,3.25880446054239));
#29552=CARTESIAN_POINT('Ctrl Pts',(38.7992659256271,1.9274788811197,4.75771200369754));
#29553=CARTESIAN_POINT('Ctrl Pts',(38.9181749246221,-0.57967967686442,5.10048726286934));
#29554=CARTESIAN_POINT('Ctrl Pts',(39.0370839236171,-2.94597502445185,4.20383503381829));
#29555=CARTESIAN_POINT('Ctrl Pts',(39.1559929226121,-4.59639334321001,2.28564380972928));
#29556=CARTESIAN_POINT('Ctrl Pts',(39.274901921607,-5.12987989233977,-0.18796343771993));
#29557=CARTESIAN_POINT('Ctrl Pts',(39.393810920602,-4.41679689760991,-2.6158941000831));
#29558=CARTESIAN_POINT('Ctrl Pts',(39.5127199195969,-2.63042399387271,-4.408160186389));
#29559=CARTESIAN_POINT('Ctrl Pts',(39.6316289185919,-0.204854489567262,
-5.12923108116021));
#29560=CARTESIAN_POINT('Ctrl Pts',(39.7505379175869,2.27049709069084,-4.60389889170027));
#29561=CARTESIAN_POINT('Ctrl Pts',(39.8694469165818,4.19410975611519,-2.95979312688258));
#29562=CARTESIAN_POINT('Ctrl Pts',(39.9883559155768,5.09855466479541,-0.596488510952733));
#29563=CARTESIAN_POINT('Ctrl Pts',(40.1072649145717,4.76402536160622,1.91183582385376));
#29564=CARTESIAN_POINT('Ctrl Pts',(40.2261739135667,3.27186245258037,3.95543710666844));
#29565=CARTESIAN_POINT('Ctrl Pts',(40.3450829125616,0.984565571626985,5.03814676373541));
#29566=CARTESIAN_POINT('Ctrl Pts',(40.4639919115567,-1.54185145170459,4.89600621130151));
#29567=CARTESIAN_POINT('Ctrl Pts',(40.5829009105515,-3.69385729548926,3.56526833460081));
#29568=CARTESIAN_POINT('Ctrl Pts',(40.7018099095466,-4.94772770082657,1.3658878530419));
#29569=CARTESIAN_POINT('Ctrl Pts',(40.8207189085415,-5.0003325304742,-1.16086506649928));
#29570=CARTESIAN_POINT('Ctrl Pts',(40.9396279075364,-3.83576987104716,-3.41457278105877));
#29571=CARTESIAN_POINT('Ctrl Pts',(41.0585369065314,-1.74326680278702,-4.82064640012023));
#29572=CARTESIAN_POINT('Ctrl Pts',(41.2170822385247,1.62279722193528,-5.17775154525906));
#29573=CARTESIAN_POINT('Ctrl Pts',(41.4152639035163,5.30562489419936,-2.39705101417185));
#29574=CARTESIAN_POINT('Ctrl Pts',(41.6530819015062,4.88493407373615,3.16747978332012));
#29575=CARTESIAN_POINT('Ctrl Pts',(41.8512635664978,0.825902295592203,5.36287863801606));
#29576=CARTESIAN_POINT('Ctrl Pts',(42.0098088984911,-2.44821262247626,4.50376129649866));
#29577=CARTESIAN_POINT('Ctrl Pts',(42.1287178974861,-4.30553515292689,2.79907213692171));
#29578=CARTESIAN_POINT('Ctrl Pts',(42.247626896481,-5.11802701027407,0.395894733536493));
#29579=CARTESIAN_POINT('Ctrl Pts',(42.366535895476,-4.6861352103675,-2.09422917054652));
#29580=CARTESIAN_POINT('Ctrl Pts',(42.485444894471,-3.11585076422253,-4.08009730671223));
#29581=CARTESIAN_POINT('Ctrl Pts',(42.6043538934659,-0.788235617082007,
-5.07216594091614));
#29582=CARTESIAN_POINT('Ctrl Pts',(42.7232628924609,1.73083522101851,-4.83285646543042));
#29583=CARTESIAN_POINT('Ctrl Pts',(42.8421718914558,3.82935364012834,-3.41856948331472));
#29584=CARTESIAN_POINT('Ctrl Pts',(42.9610808904508,4.99731057541337,-1.17385726400598));
#29585=CARTESIAN_POINT('Ctrl Pts',(43.0799898894458,4.9509232260516,1.35625123902188));
#29586=CARTESIAN_POINT('Ctrl Pts',(43.1988988884407,3.70144737026687,3.55671468709909));
#29587=CARTESIAN_POINT('Ctrl Pts',(43.3178078874357,1.55251606464634,4.89292713136518));
#29588=CARTESIAN_POINT('Ctrl Pts',(43.4367168864306,-0.973680743439912,
5.04013121413423));
#29589=CARTESIAN_POINT('Ctrl Pts',(43.5556258854256,-3.26327073385682,3.96258384566937));
#29590=CARTESIAN_POINT('Ctrl Pts',(43.6745348844206,-4.7598805622988,1.92211701262856));
#29591=CARTESIAN_POINT('Ctrl Pts',(43.7934438834155,-5.09983089787587,-0.58542529567995));
#29592=CARTESIAN_POINT('Ctrl Pts',(43.9123528824105,-4.20051347351195,-2.95070939763705));
#29593=CARTESIAN_POINT('Ctrl Pts',(44.0312618814054,-2.28046386913482,-4.59896535949367));
#29594=CARTESIAN_POINT('Ctrl Pts',(44.1501708804004,0.193742430667919,-5.12966497122579));
#29595=CARTESIAN_POINT('Ctrl Pts',(44.2690798793954,2.62086899117812,-4.41384685714979));
#29596=CARTESIAN_POINT('Ctrl Pts',(44.3879888783903,4.41111978765533,-2.62545629406751));
#29597=CARTESIAN_POINT('Ctrl Pts',(44.5068978773853,5.12946074694665,-0.199075212909377));
#29598=CARTESIAN_POINT('Ctrl Pts',(44.6258068763802,4.60133375275685,2.27568147542788));
#29599=CARTESIAN_POINT('Ctrl Pts',(44.7447158753752,2.9550745924089,4.19744358582857));
#29600=CARTESIAN_POINT('Ctrl Pts',(44.8636248743702,0.590727126290896,5.09921954321519));
#29601=CARTESIAN_POINT('Ctrl Pts',(44.9825338733651,-1.91716806673179,4.76187621633605));
#29602=CARTESIAN_POINT('Ctrl Pts',(45.1014428723601,-3.95918805933394,3.26738862140414));
#29603=CARTESIAN_POINT('Ctrl Pts',(45.220351871355,-5.03911841405869,0.978919865182178));
#29604=CARTESIAN_POINT('Ctrl Pts',(45.3392608703501,-4.89453416193924,-1.54742813436108));
#29605=CARTESIAN_POINT('Ctrl Pts',(45.458169869345,-3.56056952962606,-3.69774838487314));
#29606=CARTESIAN_POINT('Ctrl Pts',(45.5770788683399,-1.36138026087697,-4.94950929675383));
#29607=CARTESIAN_POINT('Ctrl Pts',(45.6959878673349,1.16862679740963,-4.99853077429798));
#29608=CARTESIAN_POINT('Ctrl Pts',(45.8148968663299,3.41465549562881,-3.83290051259592));
#29609=CARTESIAN_POINT('Ctrl Pts',(45.9338058653249,4.83091692341755,-1.7358687082569));
#29610=CARTESIAN_POINT('Ctrl Pts',(46.0527148643198,5.0732570714882,0.782982234705375));
#29611=CARTESIAN_POINT('Ctrl Pts',(46.1716238633147,4.08278685910157,3.11156712227454));
#29612=CARTESIAN_POINT('Ctrl Pts',(46.2905328623098,2.10019228390124,4.68403574537074));
#29613=CARTESIAN_POINT('Ctrl Pts',(46.4094418613047,-0.392752697371978,
5.11827547245928));
#29614=CARTESIAN_POINT('Ctrl Pts',(46.5283508602997,-2.79025808479161,4.30876528874866));
#29615=CARTESIAN_POINT('Ctrl Pts',(46.6472598592946,-4.50972586701803,2.45221758773953));
#29616=CARTESIAN_POINT('Ctrl Pts',(46.7661688582895,-5.13332235919528,-0.000223285183078947));
#29617=CARTESIAN_POINT('Ctrl Pts',(46.8850778572845,-4.50951252072361,-2.4526098994148));
#29618=CARTESIAN_POINT('Ctrl Pts',(47.0039868562795,-2.78988323572627,-4.30900800930841));
#29619=CARTESIAN_POINT('Ctrl Pts',(47.1228958552744,-0.392307434515635,
-5.11830962038193));
#29620=CARTESIAN_POINT('Ctrl Pts',(47.2418048542694,2.10059976089411,-4.68385302265156));
#29621=CARTESIAN_POINT('Ctrl Pts',(47.3607138532644,4.08305753260748,-3.11121193085393));
#29622=CARTESIAN_POINT('Ctrl Pts',(47.4796228522593,5.07332516737085,-0.782540886722258));
#29623=CARTESIAN_POINT('Ctrl Pts',(47.5985318512543,4.83076589425792,1.73628896447134));
#29624=CARTESIAN_POINT('Ctrl Pts',(47.7174408502492,3.41432204177779,3.83319755404034));
#29625=CARTESIAN_POINT('Ctrl Pts',(47.8363498492442,1.16819194873676,4.99863241939004));
#29626=CARTESIAN_POINT('Ctrl Pts',(47.9552588482392,-1.36181083538065,4.94939084553952));
#29627=CARTESIAN_POINT('Ctrl Pts',(48.0741678472341,-3.56089119960421,3.69743862124198));
#29628=CARTESIAN_POINT('Ctrl Pts',(48.1930768462291,-4.89466876101785,1.54700233134486));
#29629=CARTESIAN_POINT('Ctrl Pts',(48.311985845224,-5.03903323443671,-0.979358236557413));
#29630=CARTESIAN_POINT('Ctrl Pts',(48.4308948442191,-3.95890379978701,-3.26773303641874));
#29631=CARTESIAN_POINT('Ctrl Pts',(48.549803843214,-1.91675380287157,-4.76204298095343));
#29632=CARTESIAN_POINT('Ctrl Pts',(48.6687128422089,0.591170727707161,-5.09916813450712));
#29633=CARTESIAN_POINT('Ctrl Pts',(48.787621841204,2.9554397352862,-4.19718649387443));
#29634=CARTESIAN_POINT('Ctrl Pts',(48.9065308401988,4.60153170708184,-2.27528117866585));
#29635=CARTESIAN_POINT('Ctrl Pts',(49.0254398391939,5.12944340878129,0.19952145092828));
#29636=CARTESIAN_POINT('Ctrl Pts',(49.1443488381888,4.41089137158125,2.62584001823806));
#29637=CARTESIAN_POINT('Ctrl Pts',(49.2632578371838,2.62048499995396,4.4140748587091));
#29638=CARTESIAN_POINT('Ctrl Pts',(49.3821668361788,0.193296180316791,5.12968177180056));
#29639=CARTESIAN_POINT('Ctrl Pts',(49.5010758351737,-2.28086394993512,4.59876702336206));
#29640=CARTESIAN_POINT('Ctrl Pts',(49.6199848341686,-4.20077014259718,2.95034382781493));
#29641=CARTESIAN_POINT('Ctrl Pts',(49.7388938331637,-5.09988182776401,0.584981910935992));
#29642=CARTESIAN_POINT('Ctrl Pts',(49.8578028321585,-4.75971329002921,-1.92253163562839));
#29643=CARTESIAN_POINT('Ctrl Pts',(49.9767118311536,-3.26292608029717,-3.96286662502565));
#29644=CARTESIAN_POINT('Ctrl Pts',(50.0956208301484,-0.973242113989631,
-5.04021807871213));
#29645=CARTESIAN_POINT('Ctrl Pts',(50.2145298291435,1.55294139183154,-4.89278770502699));
#29646=CARTESIAN_POINT('Ctrl Pts',(50.3334388281384,3.7017574175863,-3.55640134338437));
#29647=CARTESIAN_POINT('Ctrl Pts',(50.4523478271334,4.95103990256707,-1.35580322159434));
#29648=CARTESIAN_POINT('Ctrl Pts',(50.5712568261284,4.99721101353838,1.17425745887403));
#29649=CARTESIAN_POINT('Ctrl Pts',(50.6901658251233,3.82905108905242,3.41897151974029));
#29650=CARTESIAN_POINT('Ctrl Pts',(50.8090748241183,1.73042503934585,4.83286950661864));
#29651=CARTESIAN_POINT('Ctrl Pts',(50.9279838231132,-0.78869732937638,5.07237173689479));
#29652=CARTESIAN_POINT('Ctrl Pts',(51.0468928221082,-3.11616486173899,4.07927873607974));
#29653=CARTESIAN_POINT('Ctrl Pts',(51.1658018211031,-4.68639887675184,2.09491386943815));
#29654=CARTESIAN_POINT('Ctrl Pts',(51.2847108200981,-5.11782973897512,-0.398518773119308));
#29655=CARTESIAN_POINT('Ctrl Pts',(51.403619819093,-4.3056190277905,-2.79511058784905));
#29656=CARTESIAN_POINT('Ctrl Pts',(51.522528818088,-2.44713529959719,-4.51248576524599));
#29657=CARTESIAN_POINT('Ctrl Pts',(51.641437817083,0.00600650252500089,
-5.13331872389581));
#29658=CARTESIAN_POINT('Ctrl Pts',(51.7603468160779,2.45768889968914,-4.5067467712144));
#29659=CARTESIAN_POINT('Ctrl Pts',(51.879255815073,4.312148216043,-2.7850263846104));
#29660=CARTESIAN_POINT('Ctrl Pts',(51.9981648140678,5.11874869712036,-0.386541838905528));
#29661=CARTESIAN_POINT('Ctrl Pts',(52.1170738130629,4.68148279784595,2.10587730879592));
#29662=CARTESIAN_POINT('Ctrl Pts',(52.2359828120578,3.10661131668958,4.08655608392974));
#29663=CARTESIAN_POINT('Ctrl Pts',(52.3548918110528,0.776821967382241,5.07421151952673));
#29664=CARTESIAN_POINT('Ctrl Pts',(52.4738008100477,-1.74172476260393,4.82879083719861));
#29665=CARTESIAN_POINT('Ctrl Pts',(52.5927098090427,-3.83705270620355,3.41003301954189));
#29666=CARTESIAN_POINT('Ctrl Pts',(52.7116188080376,-4.99992345441255,1.16249639376284));
#29667=CARTESIAN_POINT('Ctrl Pts',(52.8305278070326,-4.94789718966368,-1.36725835013145));
#29668=CARTESIAN_POINT('Ctrl Pts',(52.9494368060275,-3.69333647060053,-3.56532538045744));
#29669=CARTESIAN_POINT('Ctrl Pts',(53.0287094720242,-2.25888095216386,-4.45215651437191));
#29670=CARTESIAN_POINT('Ctrl Pts',(53.0683458050225,-1.47892977132682,-4.69770068559963));
#29671=CARTESIAN_POINT('Ctrl Pts',(51.2661584740964,-4.92519062564324,-0.000109311139069327));
#29672=CARTESIAN_POINT('Ctrl Pts',(51.2723425894303,-4.92531381623605,-0.127669621319975));
#29673=CARTESIAN_POINT('Ctrl Pts',(51.2785267047642,-4.92045777626379,-0.255220575265934));
#29674=CARTESIAN_POINT('Ctrl Pts',(51.2847108200981,-4.91055614340714,-0.382378635148));
#29675=CARTESIAN_POINT('Ctrl Pts',(51.3243471530964,-4.84709283524692,-1.19738271136255));
#29676=CARTESIAN_POINT('Ctrl Pts',(51.3639834860947,-4.57635593151871,-1.99624664960581));
#29677=CARTESIAN_POINT('Ctrl Pts',(51.4036198190931,-4.13124019162237,-2.68190781496027));
#29678=CARTESIAN_POINT('Ctrl Pts',(51.4432561520914,-3.68612445172606,-3.3675689803147));
#29679=CARTESIAN_POINT('Ctrl Pts',(51.4828924850897,-3.0666298756616,-3.94002737278036));
#29680=CARTESIAN_POINT('Ctrl Pts',(51.522528818088,-2.34802562060904,-4.32972872878814));
#29681=CARTESIAN_POINT('Ctrl Pts',(51.5621651510864,-1.62942136555644,-4.71943008479595));
#29682=CARTESIAN_POINT('Ctrl Pts',(51.6018014840847,-0.811707431515759,
-4.92637440434587));
#29683=CARTESIAN_POINT('Ctrl Pts',(51.641437817083,0.0057632683653263,-4.92541790534061));
#29684=CARTESIAN_POINT('Ctrl Pts',(51.6810741500813,0.823233968246388,-4.92446140633534));
#29685=CARTESIAN_POINT('Ctrl Pts',(51.7207104830796,1.64046143396783,-4.71560408877485));
#29686=CARTESIAN_POINT('Ctrl Pts',(51.7603468160779,2.35815171955416,-4.32422203222727));
#29687=CARTESIAN_POINT('Ctrl Pts',(51.7999831490763,3.07584200514046,-3.9328399756797));
#29688=CARTESIAN_POINT('Ctrl Pts',(51.8396194820746,3.69399511059172,-3.35893318014506));
#29689=CARTESIAN_POINT('Ctrl Pts',(51.8792558150729,4.13750507683024,-2.67223235809361));
#29690=CARTESIAN_POINT('Ctrl Pts',(51.9188921480713,4.58101504306879,-1.98553153604211));
#29691=CARTESIAN_POINT('Ctrl Pts',(51.9585284810695,4.84988187009458,-1.18603668747381));
#29692=CARTESIAN_POINT('Ctrl Pts',(51.9981648140678,4.9114376337284,-0.370886071906074));
#29693=CARTESIAN_POINT('Ctrl Pts',(52.0378011470662,4.97299339736222,0.444264543661619));
#29694=CARTESIAN_POINT('Ctrl Pts',(52.0774374800645,4.82723809760408,1.2750709262288));
#29695=CARTESIAN_POINT('Ctrl Pts',(52.1170738130628,4.49188186753229,2.02058724670132));
#29696=CARTESIAN_POINT('Ctrl Pts',(52.1567101460612,4.15652563746048,2.76610356717389));
#29697=CARTESIAN_POINT('Ctrl Pts',(52.1963464790595,3.63156847707506,3.42632982555178));
#29698=CARTESIAN_POINT('Ctrl Pts',(52.2359828120578,2.98079167199775,3.92105219400693));
#29699=CARTESIAN_POINT('Ctrl Pts',(52.2756191450561,2.33001486692049,4.41577456246206));
#29700=CARTESIAN_POINT('Ctrl Pts',(52.3152554780544,1.55341841715134,4.7449930409944));
#29701=CARTESIAN_POINT('Ctrl Pts',(52.3548918110528,0.745362403935769,4.86869883320588));
#29702=CARTESIAN_POINT('Ctrl Pts',(52.3945281440511,-0.0626936092798216,
4.99240462541736));
#29703=CARTESIAN_POINT('Ctrl Pts',(52.4341644770494,-0.90220918594187,4.91059773130798));
#29704=CARTESIAN_POINT('Ctrl Pts',(52.4738008100477,-1.67118829820617,4.63323464797717));
#29705=CARTESIAN_POINT('Ctrl Pts',(52.5075338733651,-2.32563887729704,4.39718086236812));
#29706=CARTESIAN_POINT('Ctrl Pts',(52.5412669366826,-2.92899917280827,4.01948372606978));
#29707=CARTESIAN_POINT('Ctrl Pts',(52.575,-3.4289504971169,3.53554284596617));
#29708=CARTESIAN_POINT('',(30.,-2.36248025497576,-3.31498400274172));
#29709=CARTESIAN_POINT('Ctrl Pts',(30.,-2.36248025497577,-3.31498400274171));
#29710=CARTESIAN_POINT('Ctrl Pts',(30.,-2.45083843615591,-3.26474897896515));
#29711=CARTESIAN_POINT('Ctrl Pts',(30.,-2.53718351659932,-3.21123764907035));
#29712=CARTESIAN_POINT('Ctrl Pts',(30.,-2.62132194611034,-3.1545569519088));
#29713=CARTESIAN_POINT('Ctrl Pts',(30.,-2.72544815198244,-3.0844112886736));
#29714=CARTESIAN_POINT('Ctrl Pts',(30.,-2.82619586363277,-3.00941311150835));
#29715=CARTESIAN_POINT('Ctrl Pts',(30.,-2.92335412828235,-2.92992006081671));
#29716=CARTESIAN_POINT('Ctrl Pts',(30.,-2.97900326879923,-2.88438898876629));
#29717=CARTESIAN_POINT('Ctrl Pts',(30.,-3.03347455648341,-2.83738236952648));
#29718=CARTESIAN_POINT('Ctrl Pts',(30.,-3.0867253031436,-2.78896042769935));
#29719=CARTESIAN_POINT('Ctrl Pts',(30.,-3.11397382321371,-2.76418281730958));
#29720=CARTESIAN_POINT('Ctrl Pts',(30.,-3.14090271699396,-2.73903454273245));
#29721=CARTESIAN_POINT('Ctrl Pts',(30.,-3.16750598172609,-2.71352320765771));
#29722=CARTESIAN_POINT('Ctrl Pts',(30.,-3.18459441442187,-2.69713616881892));
#29723=CARTESIAN_POINT('Ctrl Pts',(30.,-3.20154848687735,-2.68059932313958));
#29724=CARTESIAN_POINT('Ctrl Pts',(30.,-3.21836656153023,-2.6639146213908));
#29725=CARTESIAN_POINT('Ctrl Pts',(30.,-3.23304554999825,-2.64935204216473));
#29726=CARTESIAN_POINT('Ctrl Pts',(30.,-3.24761410550802,-2.63468359558042));
#29727=CARTESIAN_POINT('Ctrl Pts',(30.,-3.26207083845536,-2.61991145761989));
#29728=CARTESIAN_POINT('Ctrl Pts',(30.,-3.35252130085124,-2.52748762202905));
#29729=CARTESIAN_POINT('Ctrl Pts',(30.,-3.438603032295,-2.43100190270749));
#29730=CARTESIAN_POINT('Ctrl Pts',(30.,-3.52009387524001,-2.33082934687855));
#29731=CARTESIAN_POINT('Ctrl Pts',(30.,-3.6020913892008,-2.23003396609431));
#29732=CARTESIAN_POINT('Ctrl Pts',(30.,-3.67944139748576,-2.12550525076635));
#29733=CARTESIAN_POINT('Ctrl Pts',(30.,-3.75189019008547,-2.01758014367288));
#29734=CARTESIAN_POINT('Ctrl Pts',(30.,-3.77730845825652,-1.97971520188362));
#29735=CARTESIAN_POINT('Ctrl Pts',(30.,-3.80212313498671,-1.94143182393266));
#29736=CARTESIAN_POINT('Ctrl Pts',(30.,-3.82632224018495,-1.90274343853103));
#29737=CARTESIAN_POINT('Ctrl Pts',(30.,-3.84913245280764,-1.86627554892064));
#29738=CARTESIAN_POINT('Ctrl Pts',(30.,-3.87139572461206,-1.82944780129425));
#29739=CARTESIAN_POINT('Ctrl Pts',(30.,-3.89310152531943,-1.79227102496496));
#29740=CARTESIAN_POINT('Ctrl Pts',(30.,-3.90322370519929,-1.77493418388585));
#29741=CARTESIAN_POINT('Ctrl Pts',(30.,-3.91321999930958,-1.75752936221767));
#29742=CARTESIAN_POINT('Ctrl Pts',(30.,-3.92308811812892,-1.74006061666844));
#29743=CARTESIAN_POINT('Ctrl Pts',(30.,-3.95009373709925,-1.69225471821614));
#29744=CARTESIAN_POINT('Ctrl Pts',(30.,-3.97614326344458,-1.64396368682966));
#29745=CARTESIAN_POINT('Ctrl Pts',(30.,-4.00122119337617,-1.59521508212482));
#29746=CARTESIAN_POINT('Ctrl Pts',(30.,-4.0604952655639,-1.47999311913951));
#29747=CARTESIAN_POINT('Ctrl Pts',(30.,-4.11434404997915,-1.3622175869153));
#29748=CARTESIAN_POINT('Ctrl Pts',(30.,-4.16278065659499,-1.24231808149129));
#29749=CARTESIAN_POINT('Ctrl Pts',(30.,-4.21199575008708,-1.1204915172173));
#29750=CARTESIAN_POINT('Ctrl Pts',(30.,-4.2556236519386,-0.996471551733676));
#29751=CARTESIAN_POINT('Ctrl Pts',(30.,-4.29363802308023,-0.87067295455618));
#29752=CARTESIAN_POINT('Ctrl Pts',(30.,-4.32788619742269,-0.757337598510937));
#29753=CARTESIAN_POINT('Ctrl Pts',(30.,-4.35757766257454,-0.64255774676954));
#29754=CARTESIAN_POINT('Ctrl Pts',(30.,-4.38266244319943,-0.526618832262701));
#29755=CARTESIAN_POINT('Ctrl Pts',(30.,-4.40147602866809,-0.439664646382571));
#29756=CARTESIAN_POINT('Ctrl Pts',(30.,-4.41769777174343,-0.352058102522942));
#29757=CARTESIAN_POINT('Ctrl Pts',(30.,-4.43129498639204,-0.263915679232762));
#29758=CARTESIAN_POINT('Ctrl Pts',(30.,-4.43428278031165,-0.244547639294291));
#29759=CARTESIAN_POINT('Ctrl Pts',(30.,-4.43714381242759,-0.225153716221833));
#29760=CARTESIAN_POINT('Ctrl Pts',(30.,-4.4398776682558,-0.205735132850079));
#29761=CARTESIAN_POINT('Ctrl Pts',(30.,-4.44260800951335,-0.186341513480707));
#29762=CARTESIAN_POINT('Ctrl Pts',(30.,-4.4452104870011,-0.166930236534766));
#29763=CARTESIAN_POINT('Ctrl Pts',(30.,-4.44768398526052,-0.147510908969862));
#29764=CARTESIAN_POINT('Ctrl Pts',(30.,-4.46489551805196,-0.012383911448028));
#29765=CARTESIAN_POINT('Ctrl Pts',(30.,-4.47588310664295,0.123253849694283));
#29766=CARTESIAN_POINT('Ctrl Pts',(30.,-4.48063900854761,0.258956454195002));
#29767=CARTESIAN_POINT('Ctrl Pts',(30.,-4.4838586534793,0.350824245321806));
#29768=CARTESIAN_POINT('Ctrl Pts',(30.,-4.48422143108531,0.442722468953853));
#29769=CARTESIAN_POINT('Ctrl Pts',(30.,-4.48171298305417,0.534519091339923));
#29770=CARTESIAN_POINT('Ctrl Pts',(30.,-4.47802929541655,0.669323591517527));
#29771=CARTESIAN_POINT('Ctrl Pts',(30.,-4.46815627423761,0.803908859886495));
#29772=CARTESIAN_POINT('Ctrl Pts',(30.,-4.45227141268219,0.937896937469047));
#29773=CARTESIAN_POINT('Ctrl Pts',(30.,-4.43625288130477,1.0730125138602));
#29774=CARTESIAN_POINT('Ctrl Pts',(30.,-4.41412086479104,1.2075215698057));
#29775=CARTESIAN_POINT('Ctrl Pts',(30.,-4.38600459470813,1.34103973351968));
#29776=CARTESIAN_POINT('Ctrl Pts',(30.,-4.37816898656248,1.37824936367704));
#29777=CARTESIAN_POINT('Ctrl Pts',(30.,-4.36986829568835,1.41538201582188));
#29778=CARTESIAN_POINT('Ctrl Pts',(30.,-4.36110460428173,1.4524292877219));
#29779=CARTESIAN_POINT('Ctrl Pts',(30.,-4.35581208964338,1.47480264841483));
#29780=CARTESIAN_POINT('Ctrl Pts',(30.,-4.35035070722005,1.49714486882584));
#29781=CARTESIAN_POINT('Ctrl Pts',(30.,-4.34472086140207,1.51945408603399));
#29782=CARTESIAN_POINT('Ctrl Pts',(30.,-4.33978280888481,1.5390219551648));
#29783=CARTESIAN_POINT('Ctrl Pts',(30.,-4.33471469361921,1.55856590682949));
#29784=CARTESIAN_POINT('Ctrl Pts',(30.,-4.32952179802673,1.57806649106293));
#29785=CARTESIAN_POINT('Ctrl Pts',(30.,-4.29379022144892,1.71224723982657));
#29786=CARTESIAN_POINT('Ctrl Pts',(30.,-4.25210778635853,1.84456639657365));
#29787=CARTESIAN_POINT('Ctrl Pts',(30.,-4.20469449786056,1.97463023125887));
#29788=CARTESIAN_POINT('Ctrl Pts',(30.,-4.15669262462677,2.10630866788804));
#29789=CARTESIAN_POINT('Ctrl Pts',(30.,-4.10281668457366,2.23567622712646));
#29790=CARTESIAN_POINT('Ctrl Pts',(30.,-4.04324154822773,2.36232808049223));
#29791=CARTESIAN_POINT('Ctrl Pts',(30.,-3.98429992171791,2.48763314390853));
#29792=CARTESIAN_POINT('Ctrl Pts',(30.,-3.91977942670783,2.61028072798556));
#29793=CARTESIAN_POINT('Ctrl Pts',(30.,-3.84979985529667,2.72987071969418));
#29794=CARTESIAN_POINT('Ctrl Pts',(30.,-3.79916653436002,2.81639937811389));
#29795=CARTESIAN_POINT('Ctrl Pts',(30.,-3.74567425248624,2.90132720096679));
#29796=CARTESIAN_POINT('Ctrl Pts',(30.,-3.68943427790583,2.98455672438395));
#29797=CARTESIAN_POINT('Ctrl Pts',(30.,-3.66455056642679,3.02138212238069));
#29798=CARTESIAN_POINT('Ctrl Pts',(30.,-3.63912878255226,3.05787496526537));
#29799=CARTESIAN_POINT('Ctrl Pts',(30.,-3.61317781345119,3.0940263714018));
#29800=CARTESIAN_POINT('Ctrl Pts',(30.,-3.59843641711917,3.11456210568369));
#29801=CARTESIAN_POINT('Ctrl Pts',(30.,-3.58352425595821,3.1349876603743));
#29802=CARTESIAN_POINT('Ctrl Pts',(30.,-3.56844289678737,3.15530136335054));
#29803=CARTESIAN_POINT('Ctrl Pts',(30.,-3.55715233051782,3.17050909144953));
#29804=CARTESIAN_POINT('Ctrl Pts',(30.,-3.54576672263584,3.1856543120516));
#29805=CARTESIAN_POINT('Ctrl Pts',(30.,-3.5342960342479,3.20072435022002));
#29806=CARTESIAN_POINT('Ctrl Pts',(30.,-3.44911962237923,3.31262798969641));
#29807=CARTESIAN_POINT('Ctrl Pts',(30.,-3.3591351679399,3.42055154611245));
#29808=CARTESIAN_POINT('Ctrl Pts',(30.,-3.26472454399061,3.52427113846828));
#29809=CARTESIAN_POINT('Ctrl Pts',(30.,-3.16830407185099,3.63019875176792));
#29810=CARTESIAN_POINT('Ctrl Pts',(30.,-3.06726666550583,3.73174214688255));
#29811=CARTESIAN_POINT('Ctrl Pts',(30.,-2.96196811198104,3.82864480359171));
#29812=CARTESIAN_POINT('Ctrl Pts',(30.,-2.85628289510497,3.92590329335591));
#29813=CARTESIAN_POINT('Ctrl Pts',(30.,-2.74630470038239,4.01848753401441));
#29814=CARTESIAN_POINT('Ctrl Pts',(30.,-2.63234859559177,4.10611059145895));
#29815=CARTESIAN_POINT('Ctrl Pts',(30.,-2.51936339958007,4.19298709832716));
#29816=CARTESIAN_POINT('Ctrl Pts',(30.,-2.40246723845599,4.27498717097717));
#29817=CARTESIAN_POINT('Ctrl Pts',(30.,-2.28193118961066,4.35179519432719));
#29818=CARTESIAN_POINT('Ctrl Pts',(30.,-2.24443600532371,4.37568788881828));
#29819=CARTESIAN_POINT('Ctrl Pts',(30.,-2.206588376614,4.399077878459));
#29820=CARTESIAN_POINT('Ctrl Pts',(30.,-2.16839587231052,4.42195480991684));
#29821=CARTESIAN_POINT('Ctrl Pts',(30.,-2.36248025497576,-3.31498400274172));
#29822=CARTESIAN_POINT('Ctrl Pts',(30.0337330633174,-1.89383404148126,-3.64828974744648));
#29823=CARTESIAN_POINT('Ctrl Pts',(30.1071024596332,-0.719464415258844,
-4.15646547691744));
#29824=CARTESIAN_POINT('Ctrl Pts',(30.2201081889472,1.26526436571728,-4.04962641418862));
#29825=CARTESIAN_POINT('Ctrl Pts',(30.3390171879422,3.04621666442482,-2.95311080905282));
#29826=CARTESIAN_POINT('Ctrl Pts',(30.4579261869372,4.08693028190598,-1.13899868222102));
#29827=CARTESIAN_POINT('Ctrl Pts',(30.5768351859321,4.13451402698658,0.951899428186699));
#29828=CARTESIAN_POINT('Ctrl Pts',(30.6957441849271,3.17740294051253,2.81148064688808));
#29829=CARTESIAN_POINT('Ctrl Pts',(30.814653183922,1.44817770927032,3.9878689759897));
#29830=CARTESIAN_POINT('Ctrl Pts',(30.933562182917,-0.632957413458418,4.19519723441137));
#29831=CARTESIAN_POINT('Ctrl Pts',(31.052471181912,-2.56028269018139,3.38308567277929));
#29832=CARTESIAN_POINT('Ctrl Pts',(31.1655546772976,-3.80151277967511,1.82894004492933));
#29833=CARTESIAN_POINT('Ctrl Pts',(31.2390018396849,-4.0701317662764,0.576320676525326));
#29834=CARTESIAN_POINT('Ctrl Pts',(31.2728126690739,-4.07067546468071,-8.70709291818372E-5));
#29835=CARTESIAN_POINT('Origin',(27.2271873309261,0.,0.));
#29836=CARTESIAN_POINT('',(30.,2.36230756092327,-3.31488661006749));
#29837=CARTESIAN_POINT('Origin',(30.,0.,0.));
#29838=CARTESIAN_POINT('Ctrl Pts',(30.,2.36230756092327,-3.31488661006749));
#29839=CARTESIAN_POINT('Ctrl Pts',(30.0396363329983,2.91267249451483,-2.92267674082436));
#29840=CARTESIAN_POINT('Ctrl Pts',(30.118908998995,3.81372229645613,-1.85922486464953));
#29841=CARTESIAN_POINT('Ctrl Pts',(30.2378179979899,4.23847383186721,0.18897419945147));
#29842=CARTESIAN_POINT('Ctrl Pts',(30.3567269969849,3.63326524445147,2.1907645291121));
#29843=CARTESIAN_POINT('Ctrl Pts',(30.4756359959799,2.14517067243769,3.66043220391454));
#29844=CARTESIAN_POINT('Ctrl Pts',(30.5945449949748,0.135793758977664,4.24049025960433));
#29845=CARTESIAN_POINT('Ctrl Pts',(30.7134539939698,-1.90658020521281,3.79016095005708));
#29846=CARTESIAN_POINT('Ctrl Pts',(30.8323629929647,-3.48565237567683,2.4187862103776));
#29847=CARTESIAN_POINT('Ctrl Pts',(30.9202741052835,-4.02686901485062,0.970374195636228));
#29848=CARTESIAN_POINT('Ctrl Pts',(30.968548884604,-4.07067913832741,0.147388342502041));
#29849=CARTESIAN_POINT('Ctrl Pts',(30.9771873309261,-4.07052775430868,0.000104499988540334));
#29850=CARTESIAN_POINT('Ctrl Pts',(29.5066541949775,2.85821514250015,-4.01076441581687));
#29851=CARTESIAN_POINT('Ctrl Pts',(29.5462905279758,3.52411547364828,-3.53621986207105));
#29852=CARTESIAN_POINT('Ctrl Pts',(29.6255631939724,4.61431821890341,-2.24952277567846));
#29853=CARTESIAN_POINT('Ctrl Pts',(29.7444721929674,5.12823575038595,0.228644621618519));
#29854=CARTESIAN_POINT('Ctrl Pts',(29.8633811919623,4.39597870751103,2.65066092761991));
#29855=CARTESIAN_POINT('Ctrl Pts',(29.9822901909573,2.59549577736295,4.42884869285811));
#29856=CARTESIAN_POINT('Ctrl Pts',(30.1011991899523,0.16430027342226,5.1306754768582));
#29857=CARTESIAN_POINT('Ctrl Pts',(30.2201081889472,-2.30681918945408,4.58581075519745));
#29858=CARTESIAN_POINT('Ctrl Pts',(30.3390171879422,-4.21737819683287,2.9265500764304));
#29859=CARTESIAN_POINT('Ctrl Pts',(30.4579261869371,-5.10310658405598,0.556150600520288));
#29860=CARTESIAN_POINT('Ctrl Pts',(30.5768351859321,-4.74877129058131,-1.94940347074711));
#29861=CARTESIAN_POINT('Ctrl Pts',(30.6957441849271,-3.24047616811104,-3.98124455736783));
#29862=CARTESIAN_POINT('Ctrl Pts',(30.814653183922,-0.944739698215852,-5.04563850679249));
#29863=CARTESIAN_POINT('Ctrl Pts',(30.933562182917,1.58057019484585,-4.8839323181771));
#29864=CARTESIAN_POINT('Ctrl Pts',(31.052471181912,3.72179874989839,-3.53542258613139));
#29865=CARTESIAN_POINT('Ctrl Pts',(31.1713801809069,4.95862369057364,-1.32779868315432));
#29866=CARTESIAN_POINT('Ctrl Pts',(31.2902891799019,4.99049438067752,1.20248248380908));
#29867=CARTESIAN_POINT('Ctrl Pts',(31.4091981788969,3.80966619055483,3.44055837141513));
#29868=CARTESIAN_POINT('Ctrl Pts',(31.5281071778918,1.70308243813102,4.84257250835442));
#29869=CARTESIAN_POINT('Ctrl Pts',(31.6470161768868,-0.817353331486976,
5.06783305606493));
#29870=CARTESIAN_POINT('Ctrl Pts',(31.7659251758817,-3.13917080911228,4.06160127951951));
#29871=CARTESIAN_POINT('Ctrl Pts',(31.8848341748767,-4.6981642778999,2.06839327767044));
#29872=CARTESIAN_POINT('Ctrl Pts',(32.0037431738716,-5.11549559255233,-0.427437918277657));
#29873=CARTESIAN_POINT('Ctrl Pts',(32.1226521728666,-4.28975251207502,-2.81940094975718));
#29874=CARTESIAN_POINT('Ctrl Pts',(32.2415611718616,-2.42159205236551,-4.52624460934904));
#29875=CARTESIAN_POINT('Ctrl Pts',(32.3604701708566,0.0350195204882076,
-5.13320289526554));
#29876=CARTESIAN_POINT('Ctrl Pts',(32.4793791698515,2.48312128848067,-4.49278388062119));
#29877=CARTESIAN_POINT('Ctrl Pts',(32.5982881688465,4.32782023111487,-2.76061050824488));
#29878=CARTESIAN_POINT('Ctrl Pts',(32.7171971678414,5.12085127205647,-0.357603943776774));
#29879=CARTESIAN_POINT('Ctrl Pts',(32.8361061668364,4.66950647838273,2.1323010058329));
#29880=CARTESIAN_POINT('Ctrl Pts',(32.9550151658313,3.08346342604463,4.10405307365304));
#29881=CARTESIAN_POINT('Ctrl Pts',(33.0739241648263,0.748133356677078,5.07851305125401));
#29882=CARTESIAN_POINT('Ctrl Pts',(33.1928331638213,-1.76899442964414,4.81888545609981));
#29883=CARTESIAN_POINT('Ctrl Pts',(33.3117421628162,-3.85625346897966,3.38826024887523));
#29884=CARTESIAN_POINT('Ctrl Pts',(33.4306511618112,-5.00643615635466,1.134281862444));
#29885=CARTESIAN_POINT('Ctrl Pts',(33.5495601608061,-4.94004608276915,-1.39532900465872));
#29886=CARTESIAN_POINT('Ctrl Pts',(33.6684691598011,-3.67321615246874,-3.58587247798463));
#29887=CARTESIAN_POINT('Ctrl Pts',(33.7873781587961,-1.51378825893625,-4.90504265406851));
#29888=CARTESIAN_POINT('Ctrl Pts',(33.9062871577911,1.01349283479057,-5.0322788679636));
#29889=CARTESIAN_POINT('Ctrl Pts',(34.025196156786,3.2944933932768,-3.93666249668171));
#29890=CARTESIAN_POINT('Ctrl Pts',(34.144105155781,4.77492628281602,-1.88443023877182));
#29891=CARTESIAN_POINT('Ctrl Pts',(34.2630141547759,5.09504371644056,0.625721870070408));
#29892=CARTESIAN_POINT('Ctrl Pts',(34.3819231537709,4.17705659669796,2.98382246775958));
#29893=CARTESIAN_POINT('Ctrl Pts',(34.5008321527659,2.24403740267574,4.61684897592689));
#29894=CARTESIAN_POINT('Ctrl Pts',(34.6197411517608,-0.234286813404278,
5.12797309082153));
#29895=CARTESIAN_POINT('Ctrl Pts',(34.7386501507558,-2.65567892318387,4.39299075665791));
#29896=CARTESIAN_POINT('Ctrl Pts',(34.8575591497507,-4.43173639992282,2.59050396886859));
#29897=CARTESIAN_POINT('Ctrl Pts',(34.9764681487457,-5.13087416381178,0.158520176171834));
#29898=CARTESIAN_POINT('Ctrl Pts',(35.0953771477407,-4.58320051282105,-2.31198429717886));
#29899=CARTESIAN_POINT('Ctrl Pts',(35.2142861467356,-2.92180110406929,-4.22067253401449));
#29900=CARTESIAN_POINT('Ctrl Pts',(35.3331951457306,-0.550398905879517,
-5.10372994735531));
#29901=CARTESIAN_POINT('Ctrl Pts',(35.4521041447255,1.95475119114355,-4.74657203799202));
#29902=CARTESIAN_POINT('Ctrl Pts',(35.5710131437205,3.98489332255382,-3.23598880390381));
#29903=CARTESIAN_POINT('Ctrl Pts',(35.6899221427155,5.04669939211318,-0.939054618629394));
#29904=CARTESIAN_POINT('Ctrl Pts',(35.8088311417105,4.88214866385187,1.58607148488782));
#29905=CARTESIAN_POINT('Ctrl Pts',(35.9277401407054,3.53122725315149,3.72577943761101));
#29906=CARTESIAN_POINT('Ctrl Pts',(36.0466491397003,1.32221143062236,4.96011645668286));
#29907=CARTESIAN_POINT('Ctrl Pts',(36.1655581386953,-1.20810408703707,4.98913648300082));
#29908=CARTESIAN_POINT('Ctrl Pts',(36.2844671376903,-3.44484819405753,3.80578759930478));
#29909=CARTESIAN_POINT('Ctrl Pts',(36.4033761366852,-4.84448815200906,1.69762565843315));
#29910=CARTESIAN_POINT('Ctrl Pts',(36.5222851356802,-5.06690899790788,-0.823062292930284));
#29911=CARTESIAN_POINT('Ctrl Pts',(36.6411941346751,-4.05806207635667,-3.14374466449768));
#29912=CARTESIAN_POINT('Ctrl Pts',(36.7601031336701,-2.06309895753307,-4.70049157243862));
#29913=CARTESIAN_POINT('Ctrl Pts',(36.8790121326651,0.433200824037541,-5.11501078954236));
#29914=CARTESIAN_POINT('Ctrl Pts',(36.9979211316601,2.82423204608698,-4.28657341953556));
#29915=CARTESIAN_POINT('Ctrl Pts',(37.116830130655,4.52896993078687,-2.41649119531078));
#29916=CARTESIAN_POINT('Ctrl Pts',(37.23573912965,5.13316018424025,0.0408026247792082));
#29917=CARTESIAN_POINT('Ctrl Pts',(37.3546481286449,4.48998351578663,2.48818133566934));
#29918=CARTESIAN_POINT('Ctrl Pts',(37.4735571276399,2.75573298334866,4.33092762058931));
#29919=CARTESIAN_POINT('Ctrl Pts',(37.5924661266348,0.351834505657344,5.12125090327671));
#29920=CARTESIAN_POINT('Ctrl Pts',(37.7113751256298,-2.13756037313485,4.66710123916826));
#29921=CARTESIAN_POINT('Ctrl Pts',(37.8302841246247,-4.10752433556602,3.07883779592106));
#29922=CARTESIAN_POINT('Ctrl Pts',(37.9491931236198,-5.07935268326507,0.742411367522402));
#29923=CARTESIAN_POINT('Ctrl Pts',(38.0681021226147,-4.81688942970997,-1.7744223157606));
#29924=CARTESIAN_POINT('Ctrl Pts',(38.1870111216097,-3.38391359491544,-3.86006828352247));
#29925=CARTESIAN_POINT('Ctrl Pts',(38.3059201206046,-1.12864083956594,-5.00771085818741));
#29926=CARTESIAN_POINT('Ctrl Pts',(38.4248291195997,1.40089364617361,-4.93847098595927));
#29927=CARTESIAN_POINT('Ctrl Pts',(38.5437381185945,3.59000846431617,-3.66917387097732));
#29928=CARTESIAN_POINT('Ctrl Pts',(38.6626471175895,4.90674504534453,-1.50826134816256));
#29929=CARTESIAN_POINT('Ctrl Pts',(38.7815561165844,5.03113375661037,1.01916187219467));
#29930=CARTESIAN_POINT('Ctrl Pts',(38.9004651155795,3.93294859258498,3.2989258815117));
#29931=CARTESIAN_POINT('Ctrl Pts',(39.0193741145744,1.87904913788996,4.77704729317024));
#29932=CARTESIAN_POINT('Ctrl Pts',(39.1382831135694,-0.631460777071341,
5.09433350395094));
#29933=CARTESIAN_POINT('Ctrl Pts',(39.2571921125643,-2.98852815433904,4.17369639243061));
#29934=CARTESIAN_POINT('Ctrl Pts',(39.3761011115593,-4.6193708951497,2.2388264922051));
#29935=CARTESIAN_POINT('Ctrl Pts',(39.4950101105542,-5.12771248771455,-0.240047762388298));
#29936=CARTESIAN_POINT('Ctrl Pts',(39.6139191095492,-4.38998288215063,-2.66065861991797));
#29937=CARTESIAN_POINT('Ctrl Pts',(39.7328281085441,-2.58553574319963,-4.43458787788333));
#29938=CARTESIAN_POINT('Ctrl Pts',(39.8517371075391,-0.152687184564566,
-5.13117755701021));
#29939=CARTESIAN_POINT('Ctrl Pts',(39.970646106534,2.31704182252175,-4.58033746598028));
#29940=CARTESIAN_POINT('Ctrl Pts',(40.0895551055291,4.22417001907876,-2.91755367341275));
#29941=CARTESIAN_POINT('Ctrl Pts',(40.208464104524,5.10393106315724,-0.543632473763103));
#29942=CARTESIAN_POINT('Ctrl Pts',(40.327373103519,4.74519592562567,1.95807152784698));
#29943=CARTESIAN_POINT('Ctrl Pts',(40.4462821025139,3.22984460904033,3.99256580976687));
#29944=CARTESIAN_POINT('Ctrl Pts',(40.5651911015089,0.936651920722019,5.03986235081967));
#29945=CARTESIAN_POINT('Ctrl Pts',(40.7237364335022,-2.4427025544272,4.84519165873018));
#29946=CARTESIAN_POINT('Ctrl Pts',(40.9219180984937,-5.62465210210655,1.50291923965302));
#29947=CARTESIAN_POINT('Ctrl Pts',(41.1597360964838,-4.30522090115316,-3.91925381966069));
#29948=CARTESIAN_POINT('Ctrl Pts',(41.3579177614752,0.0566434889063053,
-5.42581509954019));
#29949=CARTESIAN_POINT('Ctrl Pts',(41.5164630934686,3.14760490934904,-4.04599958853725));
#29950=CARTESIAN_POINT('Ctrl Pts',(41.6353720924635,4.70319633240609,-2.0621401995762));
#29951=CARTESIAN_POINT('Ctrl Pts',(41.7542810914585,5.1143250588496,0.441143596986738));
#29952=CARTESIAN_POINT('Ctrl Pts',(41.8731900904534,4.28348653516322,2.82796599468003));
#29953=CARTESIAN_POINT('Ctrl Pts',(41.9920990894484,2.41133830213583,4.53223778943481));
#29954=CARTESIAN_POINT('Ctrl Pts',(42.1110080884434,-0.0465611259332376,
5.13283607483518));
#29955=CARTESIAN_POINT('Ctrl Pts',(42.2299170874384,-2.4932505334136,4.48731526366583));
#29956=CARTESIAN_POINT('Ctrl Pts',(42.3488260864333,-4.33402334229477,2.75078286938043));
#29957=CARTESIAN_POINT('Ctrl Pts',(42.4677350854283,-5.12164712760539,0.34609925976627));
#29958=CARTESIAN_POINT('Ctrl Pts',(42.5866440844232,-4.6646885261814,-2.14283439364853));
#29959=CARTESIAN_POINT('Ctrl Pts',(42.7055530834183,-3.07420903354032,-4.11098167683274));
#29960=CARTESIAN_POINT('Ctrl Pts',(42.8244620824131,-0.736688050284008,
-5.08019023482725));
#29961=CARTESIAN_POINT('Ctrl Pts',(42.9433710814081,1.77984776236949,-4.81488509782371));
#29962=CARTESIAN_POINT('Ctrl Pts',(43.0622800804031,3.86387828041411,-3.3795637496479));
#29963=CARTESIAN_POINT('Ctrl Pts',(43.181189079398,5.00897918721084,-1.12299782088504));
#29964=CARTESIAN_POINT('Ctrl Pts',(43.3000980783931,4.93688958102473,1.40645620742674));
#29965=CARTESIAN_POINT('Ctrl Pts',(43.4190070773879,3.6651270488325,3.59414008495642));
#29966=CARTESIAN_POINT('Ctrl Pts',(43.5379160763829,1.50273227228464,4.90844103429577));
#29967=CARTESIAN_POINT('Ctrl Pts',(43.6568250753779,-1.02482910665101,5.02998250386739));
#29968=CARTESIAN_POINT('Ctrl Pts',(43.7757340743728,-3.30335520321506,3.92922926097933));
#29969=CARTESIAN_POINT('Ctrl Pts',(43.8946430733678,-4.77916020210216,1.87366649485778));
#29970=CARTESIAN_POINT('Ctrl Pts',(44.0135520723628,-5.09362089194941,-0.63720055070383));
#29971=CARTESIAN_POINT('Ctrl Pts',(44.1324610713577,-4.17032277893803,-2.99322672697694));
#29972=CARTESIAN_POINT('Ctrl Pts',(44.2513700703527,-2.23362892033142,-4.62189357159142));
#29973=CARTESIAN_POINT('Ctrl Pts',(44.3702790693477,0.2458406804619,-5.12743217266424));
#29974=CARTESIAN_POINT('Ctrl Pts',(44.4891880683426,2.6655705652185,-4.38699577108576));
#29975=CARTESIAN_POINT('Ctrl Pts',(44.6080970673376,4.43756213047755,-2.58051170670677));
#29976=CARTESIAN_POINT('Ctrl Pts',(44.7270060663325,5.13121832020351,-0.146958775229261));
#29977=CARTESIAN_POINT('Ctrl Pts',(44.8459150653274,4.57797946441693,2.32230539650474));
#29978=CARTESIAN_POINT('Ctrl Pts',(44.9648240643225,2.91228357479588,4.22724528634906));
#29979=CARTESIAN_POINT('Ctrl Pts',(45.0837330633174,0.538897672025354,5.10495716243527));
#29980=CARTESIAN_POINT('Ctrl Pts',(45.2026420623124,-1.96544130958994,4.74215550036467));
#29981=CARTESIAN_POINT('Ctrl Pts',(45.3215510613073,-3.99217460807465,3.22700173997235));
#29982=CARTESIAN_POINT('Ctrl Pts',(45.4404600603023,-5.0488024795639,0.927680900671747));
#29983=CARTESIAN_POINT('Ctrl Pts',(45.5593690592972,-4.8785624992962,-1.59706802346811));
#29984=CARTESIAN_POINT('Ctrl Pts',(45.6782780582923,-3.52282328086189,-3.73372661866722));
#29985=CARTESIAN_POINT('Ctrl Pts',(45.7971870572872,-1.31103183059522,-4.96308310128791));
#29986=CARTESIAN_POINT('Ctrl Pts',(45.9160960562822,1.21934265240026,-4.9864016913164));
#29987=CARTESIAN_POINT('Ctrl Pts',(46.0350050552771,3.45341473367536,-3.79801593050351));
#29988=CARTESIAN_POINT('Ctrl Pts',(46.1539140542721,4.84830098173927,-1.68670564165504));
#29989=CARTESIAN_POINT('Ctrl Pts',(46.272823053267,5.06504159344358,0.834477074467225));
#29990=CARTESIAN_POINT('Ctrl Pts',(46.391732052262,4.05096822025483,3.15288039887499));
#29991=CARTESIAN_POINT('Ctrl Pts',(46.510641051257,2.05250246926194,4.70512826018573));
#29992=CARTESIAN_POINT('Ctrl Pts',(46.6295500502519,-0.444724979258798,
5.11402170741854));
#29993=CARTESIAN_POINT('Ctrl Pts',(46.7484590492469,-2.83388347833368,4.28019891621314));
#29994=CARTESIAN_POINT('Ctrl Pts',(46.8673680482419,-4.53440332512082,2.40628028630458));
#29995=CARTESIAN_POINT('Ctrl Pts',(46.9862770472368,-5.13305521628673,-0.052368670752719));
#29996=CARTESIAN_POINT('Ctrl Pts',(47.1051860462318,-4.4843656929987,-2.4982919490286));
#29997=CARTESIAN_POINT('Ctrl Pts',(47.2240950452266,-2.74596744639791,-4.33712590484156));
#29998=CARTESIAN_POINT('Ctrl Pts',(47.3430040442218,-0.340294297363466,
-5.12203066393659));
#29999=CARTESIAN_POINT('Ctrl Pts',(47.4619130432166,2.14807096237674,-4.66227299412192));
#30000=CARTESIAN_POINT('Ctrl Pts',(47.5808220422116,4.11445121325577,-3.06957481499685));
#30001=CARTESIAN_POINT('Ctrl Pts',(47.6997310412066,5.08101260776241,-0.730964575669896));
#30002=CARTESIAN_POINT('Ctrl Pts',(47.8186400402016,4.81287903290352,1.78527133673356));
#30003=CARTESIAN_POINT('Ctrl Pts',(47.9375490391965,3.37520741733752,3.86768318519946));
#30004=CARTESIAN_POINT('Ctrl Pts',(48.0564580381915,1.11735448350728,5.01024124063013));
#30005=CARTESIAN_POINT('Ctrl Pts',(48.1753670371864,-1.41201754824387,4.93530189295206));
#30006=CARTESIAN_POINT('Ctrl Pts',(48.2942760361814,-3.59826684087623,3.66107553499997));
#30007=CARTESIAN_POINT('Ctrl Pts',(48.4131850351763,-4.91013098435995,1.49720140514004));
#30008=CARTESIAN_POINT('Ctrl Pts',(48.5320940341713,-5.02882469247548,-1.03049529036943));
#30009=CARTESIAN_POINT('Ctrl Pts',(48.6510030331663,-3.92550518611198,-3.30777982413168));
#30010=CARTESIAN_POINT('Ctrl Pts',(48.7699120321612,-1.86828103914462,-4.78126806296179));
#30011=CARTESIAN_POINT('Ctrl Pts',(48.8888210311562,0.642938674940074,-5.09289978218584));
#30012=CARTESIAN_POINT('Ctrl Pts',(49.0077300301511,2.99792316411244,-4.1669479278254));
#30013=CARTESIAN_POINT('Ctrl Pts',(49.1266390291461,4.62440706983327,-2.22842042343719));
#30014=CARTESIAN_POINT('Ctrl Pts',(49.2455480281411,5.12715195221699,0.251617149677375));
#30015=CARTESIAN_POINT('Ctrl Pts',(49.3644570271361,4.38398992365829,2.67051131440959));
#30016=CARTESIAN_POINT('Ctrl Pts',(49.483366026131,2.57551065967751,4.44046654902013));
#30017=CARTESIAN_POINT('Ctrl Pts',(49.602275025126,0.141177791184851,5.13138062928017));
#30018=CARTESIAN_POINT('Ctrl Pts',(49.7211840241209,-2.32746152797901,4.57536022260056));
#30019=CARTESIAN_POINT('Ctrl Pts',(49.8400930231159,-4.23052361648418,2.90751926255194));
#30020=CARTESIAN_POINT('Ctrl Pts',(49.9590020221109,-5.10556105105169,0.533146025334083));
#30021=CARTESIAN_POINT('Ctrl Pts',(50.0779110211058,-4.73993820177943,-1.97078263000154));
#30022=CARTESIAN_POINT('Ctrl Pts',(50.1968200201008,-3.22250206106676,-3.99580765298676));
#30023=CARTESIAN_POINT('Ctrl Pts',(50.3157290190957,-0.921992272398132,
-5.04984441069379));
#30024=CARTESIAN_POINT('Ctrl Pts',(50.4346380180907,1.60256325663182,-4.87676012954613));
#30025=CARTESIAN_POINT('Ctrl Pts',(50.5535470170856,3.73769310112268,-3.51861458127488));
#30026=CARTESIAN_POINT('Ctrl Pts',(50.6724560160806,4.96455697943528,-1.30543953843589));
#30027=CARTESIAN_POINT('Ctrl Pts',(50.7913650150756,4.98502479305234,1.22495963202668));
#30028=CARTESIAN_POINT('Ctrl Pts',(50.9102740140705,3.79412287868718,3.45769140166195));
#30029=CARTESIAN_POINT('Ctrl Pts',(51.0291830130655,1.68124238654991,4.85019822635541));
#30030=CARTESIAN_POINT('Ctrl Pts',(51.1480920120605,-0.840182816358251,
5.06409812942702));
#30031=CARTESIAN_POINT('Ctrl Pts',(51.2670010110554,-3.15744239341537,4.04741381265562));
#30032=CARTESIAN_POINT('Ctrl Pts',(51.3859100100504,-4.70743739387435,2.04719984476848));
#30033=CARTESIAN_POINT('Ctrl Pts',(51.5048190090453,-5.11351793548239,-0.450485277794991));
#30034=CARTESIAN_POINT('Ctrl Pts',(51.6237280080403,-4.27700250438477,-2.83870566917055));
#30035=CARTESIAN_POINT('Ctrl Pts',(51.7426370070352,-2.40117226017362,-4.53710766699985));
#30036=CARTESIAN_POINT('Ctrl Pts',(51.8615460060303,0.0581556126824071,
-5.13300038769059));
#30037=CARTESIAN_POINT('Ctrl Pts',(51.9804550050251,2.50333449393975,-4.48153342508255));
#30038=CARTESIAN_POINT('Ctrl Pts',(52.0993640040202,4.34023276718783,-2.74110900935533));
#30039=CARTESIAN_POINT('Ctrl Pts',(52.2182730030151,5.12237890697843,-0.334464472617914));
#30040=CARTESIAN_POINT('Ctrl Pts',(52.3371820020101,4.65991385425871,2.15320299679786));
#30041=CARTESIAN_POINT('Ctrl Pts',(52.456091001005,3.06480663880283,4.11816046437608));
#30042=CARTESIAN_POINT('Ctrl Pts',(52.5353636670017,1.50529535683805,4.76007633060593));
#30043=CARTESIAN_POINT('Ctrl Pts',(52.575,0.695807839646318,4.87560011181052));
#30044=CARTESIAN_POINT('Ctrl Pts',(29.6711027966516,2.69291261530786,-3.77880514723374));
#30045=CARTESIAN_POINT('Ctrl Pts',(29.71073912965,3.32030114727046,-3.33170548832215));
#30046=CARTESIAN_POINT('Ctrl Pts',(29.7900117956466,4.34745291142099,-2.11942347200215));
#30047=CARTESIAN_POINT('Ctrl Pts',(29.9089207946416,4.83164844421304,0.215421147562834));
#30048=CARTESIAN_POINT('Ctrl Pts',(30.0278297936365,4.14174088649117,2.49736212811731));
#30049=CARTESIAN_POINT('Ctrl Pts',(30.1467387926315,2.44538740905453,4.17270986321025));
#30050=CARTESIAN_POINT('Ctrl Pts',(30.2656477916265,0.154798101940727,4.83394707110692));
#30051=CARTESIAN_POINT('Ctrl Pts',(30.3845567906213,-2.17340619470699,4.32059415348399));
#30052=CARTESIAN_POINT('Ctrl Pts',(30.5034657896164,-3.97346958978086,2.7572954544128));
#30053=CARTESIAN_POINT('Ctrl Pts',(30.6223747886113,-4.80797260259568,0.523986086940263));
#30054=CARTESIAN_POINT('Ctrl Pts',(30.7412837876063,-4.47413000003635,-1.83666132078074));
#30055=CARTESIAN_POINT('Ctrl Pts',(30.8601927866012,-3.05306588820233,-3.75099254557286));
#30056=CARTESIAN_POINT('Ctrl Pts',(30.9791017855962,-0.890101453063521,
-4.75382814441996));
#30057=CARTESIAN_POINT('Ctrl Pts',(31.0980107845912,1.48915921471079,-4.60147410052008));
#30058=CARTESIAN_POINT('Ctrl Pts',(31.2169197835862,3.50655157346604,-3.33095432218219));
#30059=CARTESIAN_POINT('Ctrl Pts',(31.3358287825811,4.67184575868903,-1.25100653596273));
#30060=CARTESIAN_POINT('Ctrl Pts',(31.4547377815761,4.7018732335852,1.1329378961668));
#30061=CARTESIAN_POINT('Ctrl Pts',(31.573646780571,3.58933727279988,3.24157650147442));
#30062=CARTESIAN_POINT('Ctrl Pts',(31.692555779566,1.60458606294434,4.56250630135687));
#30063=CARTESIAN_POINT('Ctrl Pts',(31.8114647785609,-0.770082372315719,
4.77473909014902));
#30064=CARTESIAN_POINT('Ctrl Pts',(31.9303737775559,-2.95761944150577,3.82670190264306));
#30065=CARTESIAN_POINT('Ctrl Pts',(32.0492827765509,-4.42644980240309,1.94876944986877));
#30066=CARTESIAN_POINT('Ctrl Pts',(32.1681917755458,-4.8196451029526,-0.402717397048015));
#30067=CARTESIAN_POINT('Ctrl Pts',(32.2871007745408,-4.04165819589442,-2.65634320954958));
#30068=CARTESIAN_POINT('Ctrl Pts',(32.4060097735358,-2.28154126327945,-4.2644729667982));
#30069=CARTESIAN_POINT('Ctrl Pts',(32.5249187725307,0.0329941952593177,
-4.83632831834477));
#30070=CARTESIAN_POINT('Ctrl Pts',(32.6438277715257,2.33951200651746,-4.232947411857));
#30071=CARTESIAN_POINT('Ctrl Pts',(32.7627367705207,4.07752429964364,-2.60095286497615));
#30072=CARTESIAN_POINT('Ctrl Pts',(32.8816457695156,4.82469104112772,-0.336922213153589));
#30073=CARTESIAN_POINT('Ctrl Pts',(33.0005547685106,4.39944940320316,2.00898112701842));
#30074=CARTESIAN_POINT('Ctrl Pts',(33.1194637675055,2.90513384922194,3.86669853210067));
#30075=CARTESIAN_POINT('Ctrl Pts',(33.2383727665005,0.704865677944022,4.78480141658081));
#30076=CARTESIAN_POINT('Ctrl Pts',(33.3572817654954,-1.66668608851854,4.54018917033078));
#30077=CARTESIAN_POINT('Ctrl Pts',(33.4761907644904,-3.63323021420857,3.1923029979335));
#30078=CARTESIAN_POINT('Ctrl Pts',(33.5950997634854,-4.71689302974857,1.06868160176998));
#30079=CARTESIAN_POINT('Ctrl Pts',(33.7140087624803,-4.65434257158632,-1.31463129674126));
#30080=CARTESIAN_POINT('Ctrl Pts',(33.8329177614753,-3.46077871068974,-3.37848648594147));
#30081=CARTESIAN_POINT('Ctrl Pts',(33.9518267604703,-1.42623955726036,-4.62136353745928));
#30082=CARTESIAN_POINT('Ctrl Pts',(34.0707357594652,0.954878308406255,-4.74124114933924));
#30083=CARTESIAN_POINT('Ctrl Pts',(34.1896447584602,3.10395907147953,-3.70898885178054));
#30084=CARTESIAN_POINT('Ctrl Pts',(34.3085537574551,4.49877233975909,-1.77544576235687));
#30085=CARTESIAN_POINT('Ctrl Pts',(34.4274627564501,4.80037604431206,0.589533759209166));
#30086=CARTESIAN_POINT('Ctrl Pts',(34.546371755445,3.93547995630008,2.81125554398968));
#30087=CARTESIAN_POINT('Ctrl Pts',(34.66528075444,2.11425534104551,4.34983730418886));
#30088=CARTESIAN_POINT('Ctrl Pts',(34.784189753435,-0.22073702781689,4.83140097534898));
#30089=CARTESIAN_POINT('Ctrl Pts',(34.9030987524299,-2.50208991202581,4.1389257413236));
#30090=CARTESIAN_POINT('Ctrl Pts',(35.0220077514249,-4.17543056210665,2.44068429770795));
#30091=CARTESIAN_POINT('Ctrl Pts',(35.1409167504199,-4.83413426716358,0.149352291871387));
#30092=CARTESIAN_POINT('Ctrl Pts',(35.2598257494149,-4.31813487233336,-2.17827258266522));
#30093=CARTESIAN_POINT('Ctrl Pts',(35.3787347484098,-2.75282113497098,-3.97657340167505));
#30094=CARTESIAN_POINT('Ctrl Pts',(35.4976437474048,-0.518567036838953,
-4.80855991419017));
#30095=CARTESIAN_POINT('Ctrl Pts',(35.6165527463997,1.84169976015662,-4.47205793941574));
#30096=CARTESIAN_POINT('Ctrl Pts',(35.7354617453947,3.75443028741865,-3.04883804702151));
#30097=CARTESIAN_POINT('Ctrl Pts',(35.8543707443897,4.75482767430874,-0.884745165389519));
#30098=CARTESIAN_POINT('Ctrl Pts',(35.9732797433846,4.59979360237901,1.49434234215777));
#30099=CARTESIAN_POINT('Ctrl Pts',(36.0921887423796,3.32700162284231,3.51030204137153));
#30100=CARTESIAN_POINT('Ctrl Pts',(36.2110977413745,1.24574241759582,4.67325219189535));
#30101=CARTESIAN_POINT('Ctrl Pts',(36.3300067403695,-1.13823437858544,4.70059386880629));
#30102=CARTESIAN_POINT('Ctrl Pts',(36.4489157393644,-3.24561822574471,3.58568299669183));
#30103=CARTESIAN_POINT('Ctrl Pts',(36.5678247383594,-4.5643111553328,1.59944487162223));
#30104=CARTESIAN_POINT('Ctrl Pts',(36.6867337373544,-4.77386847413717,-0.775461160658975));
#30105=CARTESIAN_POINT('Ctrl Pts',(36.8056427363493,-3.82336738639071,-2.96192877171846));
#30106=CARTESIAN_POINT('Ctrl Pts',(36.9245517353443,-1.9437813223918,-4.42864249977205));
#30107=CARTESIAN_POINT('Ctrl Pts',(37.0434607343393,0.408147009882566,-4.81918833812686));
#30108=CARTESIAN_POINT('Ctrl Pts',(37.1623697333342,2.66089490338775,-4.03866296356309));
#30109=CARTESIAN_POINT('Ctrl Pts',(37.2812787323291,4.26704067150719,-2.27673541010649));
#30110=CARTESIAN_POINT('Ctrl Pts',(37.4001877313242,4.83628807747657,0.0384428384595121));
#30111=CARTESIAN_POINT('Ctrl Pts',(37.5190967303191,4.23030900382455,2.34427941002946));
#30112=CARTESIAN_POINT('Ctrl Pts',(37.6380057293141,2.59635742772959,4.08045197579788));
#30113=CARTESIAN_POINT('Ctrl Pts',(37.756914728309,0.33148644575315,4.82506756000429));
#30114=CARTESIAN_POINT('Ctrl Pts',(37.875823727304,-2.01393632312853,4.39718326902481));
#30115=CARTESIAN_POINT('Ctrl Pts',(37.9947327262989,-3.86996903642957,2.90077573862057));
#30116=CARTESIAN_POINT('Ctrl Pts',(38.1136417252939,-4.78559248916355,0.6994746153364));
#30117=CARTESIAN_POINT('Ctrl Pts',(38.2325507242889,-4.53830858248917,-1.67180005729582));
#30118=CARTESIAN_POINT('Ctrl Pts',(38.3514597232838,-3.18820772913842,-3.6368244020829));
#30119=CARTESIAN_POINT('Ctrl Pts',(38.4703687222788,-1.0633668228208,-4.71809401024689));
#30120=CARTESIAN_POINT('Ctrl Pts',(38.5892777212738,1.31987411178072,-4.65285856920785));
#30121=CARTESIAN_POINT('Ctrl Pts',(38.7081867202687,3.38238327089769,-3.4569702112311));
#30122=CARTESIAN_POINT('Ctrl Pts',(38.8270957192637,4.62296747233291,-1.42103229083564));
#30123=CARTESIAN_POINT('Ctrl Pts',(38.9460047182586,4.74016226456139,0.960219481684352));
#30124=CARTESIAN_POINT('Ctrl Pts',(39.0649137172536,3.70548973827946,3.10813521039484));
#30125=CARTESIAN_POINT('Ctrl Pts',(39.1838227162485,1.77037587302855,4.50077068322006));
#30126=CARTESIAN_POINT('Ctrl Pts',(39.3027317152435,-0.59494076123329,4.79970690637895));
#30127=CARTESIAN_POINT('Ctrl Pts',(39.4216407142385,-2.81568908104751,3.93231408668901));
#30128=CARTESIAN_POINT('Ctrl Pts',(39.5405497132334,-4.35221337028301,2.10934579930564));
#30129=CARTESIAN_POINT('Ctrl Pts',(39.6594587122284,-4.83115544400883,-0.226164797044103));
#30130=CARTESIAN_POINT('Ctrl Pts',(39.7783677112234,-4.13609182477006,-2.50678161208584));
#30131=CARTESIAN_POINT('Ctrl Pts',(39.8972767102183,-2.43600340529342,-4.17811712717936));
#30132=CARTESIAN_POINT('Ctrl Pts',(40.0161857092132,-0.143856646546919,
-4.83442011386536));
#30133=CARTESIAN_POINT('Ctrl Pts',(40.1350947082083,2.18303761018033,-4.31543740745708));
#30134=CARTESIAN_POINT('Ctrl Pts',(40.2540037072032,3.97986861256082,-2.74881935098085));
#30135=CARTESIAN_POINT('Ctrl Pts',(40.3729127061982,4.80874939862473,-0.512191935771164));
#30136=CARTESIAN_POINT('Ctrl Pts',(40.4918217051931,4.47076141337881,1.84482806791161));
#30137=CARTESIAN_POINT('Ctrl Pts',(40.6107307041881,3.04304919662576,3.76165904263012));
#30138=CARTESIAN_POINT('Ctrl Pts',(40.7296397031831,0.88248142554386,4.74838604768767));
#30139=CARTESIAN_POINT('Ctrl Pts',(40.8881850351763,-2.30143085677862,4.56497397532002));
#30140=CARTESIAN_POINT('Ctrl Pts',(41.086366700168,-5.29935496361248,1.41599913878779));
#30141=CARTESIAN_POINT('Ctrl Pts',(41.3241846981578,-4.05623198338425,-3.69258699130876));
#30142=CARTESIAN_POINT('Ctrl Pts',(41.5223663631495,0.0533675592095104,
-5.11201753591534));
#30143=CARTESIAN_POINT('Ctrl Pts',(41.6809116951428,2.96556576247672,-3.81200252265534));
#30144=CARTESIAN_POINT('Ctrl Pts',(41.7998206941377,4.43119083216643,-1.94287801341456));
#30145=CARTESIAN_POINT('Ctrl Pts',(41.9187296931327,4.81854226610599,0.415630419076423));
#30146=CARTESIAN_POINT('Ctrl Pts',(42.0376386921276,4.03575460661519,2.66441290212816));
#30147=CARTESIAN_POINT('Ctrl Pts',(42.1565476911226,2.27188053027963,4.27011953623197));
#30148=CARTESIAN_POINT('Ctrl Pts',(42.2754566901176,-0.0438683014249705,
4.83598271267297));
#30149=CARTESIAN_POINT('Ctrl Pts',(42.3943656891125,-2.34905543488218,4.22779506787547));
#30150=CARTESIAN_POINT('Ctrl Pts',(42.5132746881075,-4.08336865897898,2.59169359954044));
#30151=CARTESIAN_POINT('Ctrl Pts',(42.6321836871024,-4.82544086902409,0.326082893101593));
#30152=CARTESIAN_POINT('Ctrl Pts',(42.7510926860974,-4.39491009331357,-2.01890532499388));
#30153=CARTESIAN_POINT('Ctrl Pts',(42.8700016850924,-2.89641467691355,-3.87322642520138));
#30154=CARTESIAN_POINT('Ctrl Pts',(42.9889106840873,-0.694082301453685,
-4.78638160161846));
#30155=CARTESIAN_POINT('Ctrl Pts',(43.1078196830823,1.67691172765244,-4.53642016949271));
#30156=CARTESIAN_POINT('Ctrl Pts',(43.2267286820773,3.64041405093096,-3.18410945360226));
#30157=CARTESIAN_POINT('Ctrl Pts',(43.3456376810722,4.7192889865021,-1.05805016349441));
#30158=CARTESIAN_POINT('Ctrl Pts',(43.4645466800672,4.65136862352993,1.32511496686864));
#30159=CARTESIAN_POINT('Ctrl Pts',(43.5834556790621,3.45315743372404,3.3862759426488));
#30160=CARTESIAN_POINT('Ctrl Pts',(43.7023646780571,1.41582298452372,4.62456537515495));
#30161=CARTESIAN_POINT('Ctrl Pts',(43.8212736770521,-0.965558956286676,
4.73907759357604));
#30162=CARTESIAN_POINT('Ctrl Pts',(43.940182676047,-3.11230836591239,3.70198551116498));
#30163=CARTESIAN_POINT('Ctrl Pts',(44.059091675042,-4.50276139379784,1.76530453073892));
#30164=CARTESIAN_POINT('Ctrl Pts',(44.1780006740369,-4.79903550770774,-0.600348579768053));
#30165=CARTESIAN_POINT('Ctrl Pts',(44.2969096730319,-3.92913558336424,-2.82011591559274));
#30166=CARTESIAN_POINT('Ctrl Pts',(44.4158186720268,-2.10444882473593,-4.35459014980295));
#30167=CARTESIAN_POINT('Ctrl Pts',(44.5347276710218,0.231622686454836,-4.83089134074941));
#30168=CARTESIAN_POINT('Ctrl Pts',(44.6536366700168,2.51140947906087,-4.13327747082228));
#30169=CARTESIAN_POINT('Ctrl Pts',(44.7725456690117,4.1809193663156,-2.43126992982818));
#30170=CARTESIAN_POINT('Ctrl Pts',(44.8914546680067,4.83445851955282,-0.138459535064545));
#30171=CARTESIAN_POINT('Ctrl Pts',(45.0103636670017,4.31321577897907,2.18799676968153));
#30172=CARTESIAN_POINT('Ctrl Pts',(45.1292726659966,2.74385404419261,3.98276602427223));
#30173=CARTESIAN_POINT('Ctrl Pts',(45.2481816649916,0.507730967406337,4.80971615429307));
#30174=CARTESIAN_POINT('Ctrl Pts',(45.3670906639865,-1.85177162437543,4.46789682861769));
#30175=CARTESIAN_POINT('Ctrl Pts',(45.4859996629815,-3.76129046576673,3.04037074255735));
#30176=CARTESIAN_POINT('Ctrl Pts',(45.6049086619765,-4.75680913142263,0.874029237076196));
#30177=CARTESIAN_POINT('Ctrl Pts',(45.7238176609714,-4.59641484070745,-1.50470290495351));
#30178=CARTESIAN_POINT('Ctrl Pts',(45.8427266599664,-3.31908368739342,-3.51778960373314));
#30179=CARTESIAN_POINT('Ctrl Pts',(45.9616356589614,-1.2352093805618,-4.67604726304423));
#30180=CARTESIAN_POINT('Ctrl Pts',(46.0805446579563,1.1488229707437,-4.69801724155464));
#30181=CARTESIAN_POINT('Ctrl Pts',(46.1994536569513,3.2536893265738,-3.57836079597794));
#30182=CARTESIAN_POINT('Ctrl Pts',(46.3183626559463,4.56790347318454,-1.58915640505304));
#30183=CARTESIAN_POINT('Ctrl Pts',(46.4372716549412,4.77210906947758,0.786215777673183));
#30184=CARTESIAN_POINT('Ctrl Pts',(46.5561806539362,3.81668379763501,2.97053614839524));
#30185=CARTESIAN_POINT('Ctrl Pts',(46.6750896529311,1.9337976733239,4.43301102848837));
#30186=CARTESIAN_POINT('Ctrl Pts',(46.7939986519261,-0.419004675043817,
4.81825645875599));
#30187=CARTESIAN_POINT('Ctrl Pts',(46.9129076509211,-2.66998815297085,4.03265712440913));
#30188=CARTESIAN_POINT('Ctrl Pts',(47.031816649916,-4.27215982993872,2.26711504064315));
#30189=CARTESIAN_POINT('Ctrl Pts',(47.150725648911,-4.83618918025851,-0.049339971655738));
#30190=CARTESIAN_POINT('Ctrl Pts',(47.2696346479059,-4.22501608320733,-2.35380528436229));
#30191=CARTESIAN_POINT('Ctrl Pts',(47.3885436469008,-2.58715667259437,-4.08629178736698));
#30192=CARTESIAN_POINT('Ctrl Pts',(47.5074526458959,-0.320613655935554,
-4.82580222384631));
#30193=CARTESIAN_POINT('Ctrl Pts',(47.6263616448908,2.02383904106705,-4.39263426156847));
#30194=CARTESIAN_POINT('Ctrl Pts',(47.7452706438858,3.87649530383263,-2.8920484745965));
#30195=CARTESIAN_POINT('Ctrl Pts',(47.8641796428807,4.78715641328979,-0.688689839296955));
#30196=CARTESIAN_POINT('Ctrl Pts',(47.9830886418758,4.53453012369092,1.68202163404398));
#30197=CARTESIAN_POINT('Ctrl Pts',(48.1019976408707,3.18000506619605,3.64399890217051));
#30198=CARTESIAN_POINT('Ctrl Pts',(48.2209066398657,1.05273320390273,4.72047805009758));
#30199=CARTESIAN_POINT('Ctrl Pts',(48.3398156388606,-1.33035467210349,4.64987275809402));
#30200=CARTESIAN_POINT('Ctrl Pts',(48.4587246378556,-3.39016403102658,3.44934023586916));
#30201=CARTESIAN_POINT('Ctrl Pts',(48.5776336368505,-4.62615758834401,1.41061199054156));
#30202=CARTESIAN_POINT('Ctrl Pts',(48.6965426358455,-4.73798674325583,-0.97089744091966));
#30203=CARTESIAN_POINT('Ctrl Pts',(48.8154516348404,-3.69847681511145,-3.11647709250932));
#30204=CARTESIAN_POINT('Ctrl Pts',(48.9343606338354,-1.76023053843739,-4.50474734825446));
#30205=CARTESIAN_POINT('Ctrl Pts',(49.0532696328304,0.605754844298045,-4.79835610273556));
#30206=CARTESIAN_POINT('Ctrl Pts',(49.1721786318254,2.8245407381406,-3.92595591399616));
#30207=CARTESIAN_POINT('Ctrl Pts',(49.2910876308202,4.35695828193666,-2.09954155698525));
#30208=CARTESIAN_POINT('Ctrl Pts',(49.4099966298153,4.83062732662176,0.23706507831365));
#30209=CARTESIAN_POINT('Ctrl Pts',(49.5289056288102,4.13044546411404,2.51606448407709));
#30210=CARTESIAN_POINT('Ctrl Pts',(49.6478146278052,2.42655811424978,4.18365581019525));
#30211=CARTESIAN_POINT('Ctrl Pts',(49.7667236268001,0.133012889488217,4.83461144161723));
#30212=CARTESIAN_POINT('Ctrl Pts',(49.8856326257951,-2.19285470052332,4.31074801886369));
#30213=CARTESIAN_POINT('Ctrl Pts',(50.0045416247901,-3.98585475487434,2.7393652720375));
#30214=CARTESIAN_POINT('Ctrl Pts',(50.123450623785,-4.81028511750694,0.502311962481408));
#30215=CARTESIAN_POINT('Ctrl Pts',(50.24235962278,-4.46580776567652,-1.85680403390435));
#30216=CARTESIAN_POINT('Ctrl Pts',(50.361268621775,-3.03613129888863,-3.76471339650777));
#30217=CARTESIAN_POINT('Ctrl Pts',(50.4801776207699,-0.868669605950452,
-4.75779080332068));
#30218=CARTESIAN_POINT('Ctrl Pts',(50.5990866197649,1.50988032581682,-4.59471670953278));
#30219=CARTESIAN_POINT('Ctrl Pts',(50.7179956187599,3.52152668793086,-3.31511839449318));
#30220=CARTESIAN_POINT('Ctrl Pts',(50.8369046177548,4.67743590065847,-1.22994051403022));
#30221=CARTESIAN_POINT('Ctrl Pts',(50.9558136167497,4.69671997507175,1.15411509696296));
#30222=CARTESIAN_POINT('Ctrl Pts',(51.0747226157447,3.57469289561859,3.25771865697702));
#30223=CARTESIAN_POINT('Ctrl Pts',(51.1936316147397,1.58400911282353,4.56969099221527));
#30224=CARTESIAN_POINT('Ctrl Pts',(51.3125406137346,-0.791591532664319,
4.77122016992817));
#30225=CARTESIAN_POINT('Ctrl Pts',(51.4314496127296,-2.97483430372514,3.81333495628239));
#30226=CARTESIAN_POINT('Ctrl Pts',(51.5503586117245,-4.43518661532507,1.92880172176646));
#30227=CARTESIAN_POINT('Ctrl Pts',(51.6692676107195,-4.81778182205635,-0.424431831441317));
#30228=CARTESIAN_POINT('Ctrl Pts',(51.7881766097145,-4.02964557443573,-2.67453145635796));
#30229=CARTESIAN_POINT('Ctrl Pts',(51.9070856087094,-2.26230243301161,-4.27470776842447));
#30230=CARTESIAN_POINT('Ctrl Pts',(52.0259946077044,0.0547922305479365,
-4.83613752262923));
#30231=CARTESIAN_POINT('Ctrl Pts',(52.1449036066994,2.35855619782664,-4.22234761718183));
#30232=CARTESIAN_POINT('Ctrl Pts',(52.2638126056944,4.08921896687908,-2.58257921927111));
#30233=CARTESIAN_POINT('Ctrl Pts',(52.3827216046893,4.82613032653762,-0.315120994319956));
#30234=CARTESIAN_POINT('Ctrl Pts',(52.5016306036843,4.39041156062324,2.02867426848899));
#30235=CARTESIAN_POINT('Ctrl Pts',(52.6205396026792,2.8875560619597,3.87999003345837));
#30236=CARTESIAN_POINT('Ctrl Pts',(52.6998122686759,1.41823783518537,4.48478122234856));
#30237=CARTESIAN_POINT('Ctrl Pts',(52.7394486016742,0.655566364250171,4.59362378047095));
#30238=CARTESIAN_POINT('Ctrl Pts',(29.8355513983258,2.52761008811556,-3.54684587865062));
#30239=CARTESIAN_POINT('Ctrl Pts',(29.8751877313241,3.11648682089265,-3.12719111457326));
#30240=CARTESIAN_POINT('Ctrl Pts',(29.9544603973208,4.08058760393856,-1.98932416832584));
#30241=CARTESIAN_POINT('Ctrl Pts',(30.0733693963157,4.53506113804012,0.202197673507152));
#30242=CARTESIAN_POINT('Ctrl Pts',(30.1922783953107,3.88750306547132,2.34406332861471));
#30243=CARTESIAN_POINT('Ctrl Pts',(30.3111873943056,2.29527904074611,3.9165710335624));
#30244=CARTESIAN_POINT('Ctrl Pts',(30.4300963933006,0.145295930459194,4.53721866535562));
#30245=CARTESIAN_POINT('Ctrl Pts',(30.5490053922956,-2.0399931999599,4.05537755177054));
#30246=CARTESIAN_POINT('Ctrl Pts',(30.6679143912905,-3.72956098272885,2.5880408323952));
#30247=CARTESIAN_POINT('Ctrl Pts',(30.7868233902855,-4.51283862113539,0.491821573360237));
#30248=CARTESIAN_POINT('Ctrl Pts',(30.9057323892805,-4.19948870949138,-1.72391917081437));
#30249=CARTESIAN_POINT('Ctrl Pts',(31.0246413882754,-2.86565560829363,-3.5207405337779));
#30250=CARTESIAN_POINT('Ctrl Pts',(31.1435503872704,-0.835463207911184,
-4.46201778204743));
#30251=CARTESIAN_POINT('Ctrl Pts',(31.2624593862653,1.39774823457573,-4.31901588286307));
#30252=CARTESIAN_POINT('Ctrl Pts',(31.3813683852603,3.29130439703369,-3.12648605823298));
#30253=CARTESIAN_POINT('Ctrl Pts',(31.5002773842552,4.38506782680442,-1.17421438877115));
#30254=CARTESIAN_POINT('Ctrl Pts',(31.6191863832503,4.41325208649288,1.06339330852454));
#30255=CARTESIAN_POINT('Ctrl Pts',(31.7380953822452,3.36900835504494,3.0425946315337));
#30256=CARTESIAN_POINT('Ctrl Pts',(31.8570043812402,1.50608968775765,4.28244009435932));
#30257=CARTESIAN_POINT('Ctrl Pts',(31.9759133802351,-0.722811413144461,
4.48164512423311));
#30258=CARTESIAN_POINT('Ctrl Pts',(32.0948223792301,-2.77606807389926,3.5918025257666));
#30259=CARTESIAN_POINT('Ctrl Pts',(32.213731378225,-4.15473532690629,1.8291456220671));
#30260=CARTESIAN_POINT('Ctrl Pts',(32.33264037722,-4.52379461335287,-0.377996875818372));
#30261=CARTESIAN_POINT('Ctrl Pts',(32.451549376215,-3.79356387971383,-2.49328546934199));
#30262=CARTESIAN_POINT('Ctrl Pts',(32.5704583752099,-2.14149047419338,-4.00270132424737));
#30263=CARTESIAN_POINT('Ctrl Pts',(32.6893673742049,0.0309688700304269,
-4.539453741424));
#30264=CARTESIAN_POINT('Ctrl Pts',(32.8082763731999,2.19590272455425,-3.9731109430928));
#30265=CARTESIAN_POINT('Ctrl Pts',(32.9271853721948,3.82722836817241,-2.44129522170742));
#30266=CARTESIAN_POINT('Ctrl Pts',(33.0460943711898,4.52853081019897,-0.316240482530403));
#30267=CARTESIAN_POINT('Ctrl Pts',(33.1650033701847,4.12939232802359,1.88566124820393));
#30268=CARTESIAN_POINT('Ctrl Pts',(33.2839123691797,2.72680427239924,3.62934399054829));
#30269=CARTESIAN_POINT('Ctrl Pts',(33.4028213681747,0.66159799921097,4.49108978190761));
#30270=CARTESIAN_POINT('Ctrl Pts',(33.5217303671696,-1.56437774739295,4.26149288456175));
#30271=CARTESIAN_POINT('Ctrl Pts',(33.6406393661646,-3.41020695943747,2.99634574699176));
#30272=CARTESIAN_POINT('Ctrl Pts',(33.7595483651595,-4.42734990314248,1.00308134109595));
#30273=CARTESIAN_POINT('Ctrl Pts',(33.8784573641545,-4.36863906040348,-1.23393358882379));
#30274=CARTESIAN_POINT('Ctrl Pts',(33.9973663631495,-3.24834126891074,-3.17110049389832));
#30275=CARTESIAN_POINT('Ctrl Pts',(34.1162753621444,-1.33869085558447,-4.33768442085004));
#30276=CARTESIAN_POINT('Ctrl Pts',(34.2351843611394,0.896263782021944,-4.45020343071488));
#30277=CARTESIAN_POINT('Ctrl Pts',(34.3540933601343,2.91342474968224,-3.48131520687938));
#30278=CARTESIAN_POINT('Ctrl Pts',(34.4730023591293,4.22261839670216,-1.66646128594193));
#30279=CARTESIAN_POINT('Ctrl Pts',(34.5919113581243,4.50570837218357,0.553345648347923));
#30280=CARTESIAN_POINT('Ctrl Pts',(34.7108203571193,3.69390331590221,2.63868862021977));
#30281=CARTESIAN_POINT('Ctrl Pts',(34.8297293561142,1.98447327941527,4.08282563245083));
#30282=CARTESIAN_POINT('Ctrl Pts',(34.9486383551092,-0.207187242229502,
4.53482885987642));
#30283=CARTESIAN_POINT('Ctrl Pts',(35.0675473541041,-2.34850090086774,3.88486072598929));
#30284=CARTESIAN_POINT('Ctrl Pts',(35.1864563530991,-3.91912472429048,2.29086462654731));
#30285=CARTESIAN_POINT('Ctrl Pts',(35.305365352094,-4.53739437051538,0.140184407570935));
#30286=CARTESIAN_POINT('Ctrl Pts',(35.424274351089,-4.05306923184566,-2.04456086815158));
#30287=CARTESIAN_POINT('Ctrl Pts',(35.543183350084,-2.58384116587268,-3.73247426933561));
#30288=CARTESIAN_POINT('Ctrl Pts',(35.6620923490789,-0.486735167798389,
-4.51338988102501));
#30289=CARTESIAN_POINT('Ctrl Pts',(35.7810013480739,1.72864832916969,-4.19754384083949));
#30290=CARTESIAN_POINT('Ctrl Pts',(35.8999103470689,3.52396725228349,-2.8616872901392));
#30291=CARTESIAN_POINT('Ctrl Pts',(36.0188193460638,4.46295595650429,-0.830435712149652));
#30292=CARTESIAN_POINT('Ctrl Pts',(36.1377283450588,4.31743854090615,1.40261319942774));
#30293=CARTESIAN_POINT('Ctrl Pts',(36.2566373440538,3.12277599253313,3.29482464513204));
#30294=CARTESIAN_POINT('Ctrl Pts',(36.3755463430487,1.16927340456928,4.38638792710784));
#30295=CARTESIAN_POINT('Ctrl Pts',(36.4944553420437,-1.06836467013381,4.41205125461175));
#30296=CARTESIAN_POINT('Ctrl Pts',(36.6133643410386,-3.04638825743189,3.3655783940789));
#30297=CARTESIAN_POINT('Ctrl Pts',(36.7322733400336,-4.28413415865655,1.5012640848113));
#30298=CARTESIAN_POINT('Ctrl Pts',(36.8511823390286,-4.48082795036645,-0.727860028387663));
#30299=CARTESIAN_POINT('Ctrl Pts',(36.9700913380235,-3.58867269642476,-2.78011287893923));
#30300=CARTESIAN_POINT('Ctrl Pts',(37.0890003370185,-1.82446368725053,-4.15679342710547));
#30301=CARTESIAN_POINT('Ctrl Pts',(37.2079093360134,0.383093195727588,-4.52336588671137));
#30302=CARTESIAN_POINT('Ctrl Pts',(37.3268183350084,2.49755776068852,-3.79075250759061));
#30303=CARTESIAN_POINT('Ctrl Pts',(37.4457273340033,4.00511141222751,-2.13697962490221));
#30304=CARTESIAN_POINT('Ctrl Pts',(37.5646363329983,4.5394159707129,0.036083052139815));
#30305=CARTESIAN_POINT('Ctrl Pts',(37.6835453319933,3.97063449186246,2.20037748438958));
#30306=CARTESIAN_POINT('Ctrl Pts',(37.8024543309883,2.43698187211053,3.82997633100645));
#30307=CARTESIAN_POINT('Ctrl Pts',(37.9213633299832,0.31113838584895,4.52888421673187));
#30308=CARTESIAN_POINT('Ctrl Pts',(38.0402723289782,-1.8903122731222,4.12726529888137));
#30309=CARTESIAN_POINT('Ctrl Pts',(38.1591813279731,-3.63241373729313,2.72271368132007));
#30310=CARTESIAN_POINT('Ctrl Pts',(38.2780903269681,-4.49183229506202,0.6565378631504));
#30311=CARTESIAN_POINT('Ctrl Pts',(38.3969993259631,-4.25972773526838,-1.56917779883104));
#30312=CARTESIAN_POINT('Ctrl Pts',(38.515908324958,-2.9925018633614,-3.41358052064332));
#30313=CARTESIAN_POINT('Ctrl Pts',(38.634817323953,-0.998092806075667,-4.42847716230638));
#30314=CARTESIAN_POINT('Ctrl Pts',(38.753726322948,1.23885457738782,-4.36724615245642));
#30315=CARTESIAN_POINT('Ctrl Pts',(38.8726353219429,3.17475807747922,-3.24476655148489));
#30316=CARTESIAN_POINT('Ctrl Pts',(38.9915443209379,4.33918989932127,-1.33380323350872));
#30317=CARTESIAN_POINT('Ctrl Pts',(39.1104533199328,4.44919077251242,0.901277091174026));
#30318=CARTESIAN_POINT('Ctrl Pts',(39.2293623189278,3.47803088397395,2.91734453927799));
#30319=CARTESIAN_POINT('Ctrl Pts',(39.3482713179227,1.66170260816715,4.22449407326989));
#30320=CARTESIAN_POINT('Ctrl Pts',(39.4671803169177,-0.558420745395243,
4.50508030880696));
#30321=CARTESIAN_POINT('Ctrl Pts',(39.5860893159126,-2.64285000775597,3.69093178094741));
#30322=CARTESIAN_POINT('Ctrl Pts',(39.7049983149076,-4.08505584541632,1.97986510640618));
#30323=CARTESIAN_POINT('Ctrl Pts',(39.8239073139026,-4.53459840030311,-0.212281831699906));
#30324=CARTESIAN_POINT('Ctrl Pts',(39.9428163128976,-3.88220076738949,-2.35290460425372));
#30325=CARTESIAN_POINT('Ctrl Pts',(40.0617253118925,-2.2864710673872,-3.92164637647539));
#30326=CARTESIAN_POINT('Ctrl Pts',(40.1806343108875,-0.135026108529271,
-4.5376626707205));
#30327=CARTESIAN_POINT('Ctrl Pts',(40.2995433098824,2.0490333978389,-4.05053734893388));
#30328=CARTESIAN_POINT('Ctrl Pts',(40.4184523088774,3.73556720604287,-2.58008502854894));
#30329=CARTESIAN_POINT('Ctrl Pts',(40.5373613078723,4.51356773409222,-0.480751397779228));
#30330=CARTESIAN_POINT('Ctrl Pts',(40.6562703068674,4.19632690113196,1.73158460797626));
#30331=CARTESIAN_POINT('Ctrl Pts',(40.7751793058622,2.8562537842112,3.53075227549335));
#30332=CARTESIAN_POINT('Ctrl Pts',(40.8940883048572,0.828310930365704,4.45690974455567));
#30333=CARTESIAN_POINT('Ctrl Pts',(41.0526336368505,-2.16015915913004,4.28475629190986));
#30334=CARTESIAN_POINT('Ctrl Pts',(41.2508153018422,-4.9740578251184,1.32907903792256));
#30335=CARTESIAN_POINT('Ctrl Pts',(41.488633299832,-3.80724306561534,-3.46592016295684));
#30336=CARTESIAN_POINT('Ctrl Pts',(41.6868149648236,0.0500916295127203,
-4.79821997229049));
#30337=CARTESIAN_POINT('Ctrl Pts',(41.845360296817,2.7835266156044,-3.57800545677343));
#30338=CARTESIAN_POINT('Ctrl Pts',(41.9642692958118,4.15918533192678,-1.82361582725293));
#30339=CARTESIAN_POINT('Ctrl Pts',(42.0831782948069,4.52275947336236,0.390117241166111));
#30340=CARTESIAN_POINT('Ctrl Pts',(42.2020872938018,3.78802267806716,2.5008598095763));
#30341=CARTESIAN_POINT('Ctrl Pts',(42.3209962927968,2.13242275842343,4.00800128302914));
#30342=CARTESIAN_POINT('Ctrl Pts',(42.4399052917917,-0.0411754769167031,
4.53912935051075));
#30343=CARTESIAN_POINT('Ctrl Pts',(42.5588142907867,-2.20486033635077,3.96827487208511));
#30344=CARTESIAN_POINT('Ctrl Pts',(42.6777232897817,-3.8327139756632,2.43260432970045));
#30345=CARTESIAN_POINT('Ctrl Pts',(42.7966322887766,-4.52923461044278,0.306066526436917));
#30346=CARTESIAN_POINT('Ctrl Pts',(42.9155412877716,-4.12513166044574,-1.89497625633923));
#30347=CARTESIAN_POINT('Ctrl Pts',(43.0344502867665,-2.71862032028679,-3.63547117357001));
#30348=CARTESIAN_POINT('Ctrl Pts',(43.1533592857615,-0.651476552623365,
-4.49257296840967));
#30349=CARTESIAN_POINT('Ctrl Pts',(43.2722682847565,1.57397569293539,-4.25795524116172));
#30350=CARTESIAN_POINT('Ctrl Pts',(43.3911772837514,3.4169498214478,-2.98865515755662));
#30351=CARTESIAN_POINT('Ctrl Pts',(43.5100862827464,4.42959878579337,-0.993102506103781));
#30352=CARTESIAN_POINT('Ctrl Pts',(43.6289952817414,4.36584766603513,1.24377372631055));
#30353=CARTESIAN_POINT('Ctrl Pts',(43.7479042807363,3.24118781861557,3.17841180034119));
#30354=CARTESIAN_POINT('Ctrl Pts',(43.8668132797312,1.32891369676281,4.34068971601413));
#30355=CARTESIAN_POINT('Ctrl Pts',(43.9857222787263,-0.906288805922349,
4.44817268328468));
#30356=CARTESIAN_POINT('Ctrl Pts',(44.1046312777211,-2.92126152860971,3.47474176135063));
#30357=CARTESIAN_POINT('Ctrl Pts',(44.2235402767162,-4.22636258549353,1.65694256662005));
#30358=CARTESIAN_POINT('Ctrl Pts',(44.3424492757111,-4.50445012346606,-0.563496608832273));
#30359=CARTESIAN_POINT('Ctrl Pts',(44.4613582747061,-3.68794838779045,-2.64700510420854));
#30360=CARTESIAN_POINT('Ctrl Pts',(44.580267273701,-1.97526872914043,-4.08728672801447));
#30361=CARTESIAN_POINT('Ctrl Pts',(44.699176272696,0.217404692447769,-4.53435050883458));
#30362=CARTESIAN_POINT('Ctrl Pts',(44.818085271691,2.35724839290324,-3.8795591705588));
#30363=CARTESIAN_POINT('Ctrl Pts',(44.9369942706859,3.92427660215364,-2.28202815294958));
#30364=CARTESIAN_POINT('Ctrl Pts',(45.0559032696809,4.53769871890213,-0.129960294899828));
#30365=CARTESIAN_POINT('Ctrl Pts',(45.1748122686759,4.04845209354121,2.05368814285831));
#30366=CARTESIAN_POINT('Ctrl Pts',(45.2937212676708,2.57542451358934,3.7382867621954));
#30367=CARTESIAN_POINT('Ctrl Pts',(45.4126302666658,0.476564262787324,4.51447514615088));
#30368=CARTESIAN_POINT('Ctrl Pts',(45.5315392656607,-1.73810193916093,4.1936381568707));
#30369=CARTESIAN_POINT('Ctrl Pts',(45.6504482646557,-3.5304063234588,2.85373974514235));
#30370=CARTESIAN_POINT('Ctrl Pts',(45.7693572636506,-4.46481578328136,0.820377573480641));
#30371=CARTESIAN_POINT('Ctrl Pts',(45.8882662626457,-4.31426718211871,-1.41233778643891));
#30372=CARTESIAN_POINT('Ctrl Pts',(46.0071752616405,-3.11534409392495,-3.30185258879907));
#30373=CARTESIAN_POINT('Ctrl Pts',(46.1260842606356,-1.15938693052836,-4.38901142480054));
#30374=CARTESIAN_POINT('Ctrl Pts',(46.2449932596305,1.07830328908713,-4.40963279179289));
#30375=CARTESIAN_POINT('Ctrl Pts',(46.3639022586255,3.05396391947226,-3.35870566145235));
#30376=CARTESIAN_POINT('Ctrl Pts',(46.4828112576204,4.28750596462981,-1.49160716845105));
#30377=CARTESIAN_POINT('Ctrl Pts',(46.6017202566154,4.47917654551159,0.737954480879145));
#30378=CARTESIAN_POINT('Ctrl Pts',(46.7206292556103,3.58239937501518,2.78819189791547));
#30379=CARTESIAN_POINT('Ctrl Pts',(46.8395382546053,1.81509287738585,4.160893796791));
#30380=CARTESIAN_POINT('Ctrl Pts',(46.9584472536003,-0.393284370828836,
4.52249121009344));
#30381=CARTESIAN_POINT('Ctrl Pts',(47.0773562525952,-2.50609282760802,3.78511533260512));
#30382=CARTESIAN_POINT('Ctrl Pts',(47.1962652515902,-4.00991633475661,2.12794979498173));
#30383=CARTESIAN_POINT('Ctrl Pts',(47.3151742505851,-4.53932314423028,-0.0463112725587562));
#30384=CARTESIAN_POINT('Ctrl Pts',(47.4340832495801,-3.96566647341596,-2.20931861969599));
#30385=CARTESIAN_POINT('Ctrl Pts',(47.5529922485751,-2.42834589879083,-3.83545766989239));
#30386=CARTESIAN_POINT('Ctrl Pts',(47.67190124757,-0.300933014507645,-4.52957378375604));
#30387=CARTESIAN_POINT('Ctrl Pts',(47.790810246565,1.89960711975736,-4.12299552901502));
#30388=CARTESIAN_POINT('Ctrl Pts',(47.90971924556,3.63853939440949,-2.71452213419616));
#30389=CARTESIAN_POINT('Ctrl Pts',(48.0286282445549,4.49330021881717,-0.646415102924012));
#30390=CARTESIAN_POINT('Ctrl Pts',(48.1475372435499,4.25618121447832,1.5787719313544));
#30391=CARTESIAN_POINT('Ctrl Pts',(48.2664462425448,2.98480271505459,3.42031461914156));
#30392=CARTESIAN_POINT('Ctrl Pts',(48.3853552415398,0.988111924298174,4.43071485956504));
#30393=CARTESIAN_POINT('Ctrl Pts',(48.5042642405347,-1.24869179596311,4.36444362323597));
#30394=CARTESIAN_POINT('Ctrl Pts',(48.6231732395298,-3.18206122117694,3.23760493673836));
#30395=CARTESIAN_POINT('Ctrl Pts',(48.7420822385247,-4.34218419232808,1.32402257594309));
#30396=CARTESIAN_POINT('Ctrl Pts',(48.8609912375196,-4.44714879403618,-0.911299591469888));
#30397=CARTESIAN_POINT('Ctrl Pts',(48.9799002365147,-3.47144844411091,-2.92517436088697));
#30398=CARTESIAN_POINT('Ctrl Pts',(49.0988092355095,-1.65218003773015,-4.22822663354714));
#30399=CARTESIAN_POINT('Ctrl Pts',(49.2177182345046,0.568571013656015,-4.50381242328528));
#30400=CARTESIAN_POINT('Ctrl Pts',(49.3366272334995,2.65115831216877,-3.68496390016692));
#30401=CARTESIAN_POINT('Ctrl Pts',(49.4555362324945,4.08950949404005,-1.97066269053332));
#30402=CARTESIAN_POINT('Ctrl Pts',(49.5744452314894,4.53410270102655,0.222513006949929));
#30403=CARTESIAN_POINT('Ctrl Pts',(49.6933542304844,3.8769010045698,2.36161765374458));
#30404=CARTESIAN_POINT('Ctrl Pts',(49.8122632294793,2.27760556882206,3.92684507137038));
#30405=CARTESIAN_POINT('Ctrl Pts',(49.9311722284743,0.124847987791581,4.53784225395429));
#30406=CARTESIAN_POINT('Ctrl Pts',(50.0500812274693,-2.05824787306763,4.04613581512682));
#30407=CARTESIAN_POINT('Ctrl Pts',(50.1689902264642,-3.74118589326448,2.57121128152305));
#30408=CARTESIAN_POINT('Ctrl Pts',(50.2878992254592,-4.5150091839622,0.471477899628734));
#30409=CARTESIAN_POINT('Ctrl Pts',(50.4068082244542,-4.19167732957359,-1.74282543780715));
#30410=CARTESIAN_POINT('Ctrl Pts',(50.5257172234491,-2.84976053671051,-3.53361914002879));
#30411=CARTESIAN_POINT('Ctrl Pts',(50.6446262224441,-0.815346939502767,
-4.46573719594757));
#30412=CARTESIAN_POINT('Ctrl Pts',(50.763535221439,1.41719739500182,-4.31267328951943));
#30413=CARTESIAN_POINT('Ctrl Pts',(50.882444220434,3.30536027473904,-3.11162220771148));
#30414=CARTESIAN_POINT('Ctrl Pts',(51.001353219429,4.39031482188165,-1.15444148962456));
#30415=CARTESIAN_POINT('Ctrl Pts',(51.1202622184239,4.40841515709115,1.08327056189923));
#30416=CARTESIAN_POINT('Ctrl Pts',(51.2391712174189,3.35526291255,3.05774591229208));
#30417=CARTESIAN_POINT('Ctrl Pts',(51.3580802164139,1.48677583909716,4.28918375807513));
#30418=CARTESIAN_POINT('Ctrl Pts',(51.4769892154088,-0.74300024897039,4.47834221042933));
#30419=CARTESIAN_POINT('Ctrl Pts',(51.5958982144038,-2.7922262140349,3.57925609990917));
#30420=CARTESIAN_POINT('Ctrl Pts',(51.7148072133987,-4.1629358367758,1.81040359876443));
#30421=CARTESIAN_POINT('Ctrl Pts',(51.8337162123937,-4.52204570863031,-0.398378385087645));
#30422=CARTESIAN_POINT('Ctrl Pts',(51.9526252113887,-3.7822886444867,-2.51035724354537));
#30423=CARTESIAN_POINT('Ctrl Pts',(52.0715342103836,-2.12343260584961,-4.01230786984909));
#30424=CARTESIAN_POINT('Ctrl Pts',(52.1904432093786,0.0514288484134658,
-4.53927465756786));
#30425=CARTESIAN_POINT('Ctrl Pts',(52.3093522083735,2.21377790171352,-3.96316180928111));
#30426=CARTESIAN_POINT('Ctrl Pts',(52.4282612073685,3.83820516657033,-2.42404942918688));
#30427=CARTESIAN_POINT('Ctrl Pts',(52.5471702063634,4.5298817460968,-0.295777516022001));
#30428=CARTESIAN_POINT('Ctrl Pts',(52.6660792053584,4.12090926698776,1.90414554018012));
#30429=CARTESIAN_POINT('Ctrl Pts',(52.7849882043534,2.71030548511656,3.64181960254066));
#30430=CARTESIAN_POINT('Ctrl Pts',(52.86426087035,1.33118031353268,4.20948611409119));
#30431=CARTESIAN_POINT('Ctrl Pts',(52.9038972033484,0.615324888854025,4.31164744913139));
#30432=CARTESIAN_POINT('Ctrl Pts',(30.,2.36230756092327,-3.31488661006749));
#30433=CARTESIAN_POINT('Ctrl Pts',(30.0396363329983,2.91267249451483,-2.92267674082436));
#30434=CARTESIAN_POINT('Ctrl Pts',(30.118908998995,3.81372229645613,-1.85922486464953));
#30435=CARTESIAN_POINT('Ctrl Pts',(30.2378179979899,4.23847383186721,0.18897419945147));
#30436=CARTESIAN_POINT('Ctrl Pts',(30.3567269969849,3.63326524445147,2.1907645291121));
#30437=CARTESIAN_POINT('Ctrl Pts',(30.4756359959799,2.14517067243769,3.66043220391454));
#30438=CARTESIAN_POINT('Ctrl Pts',(30.5945449949748,0.135793758977664,4.24049025960433));
#30439=CARTESIAN_POINT('Ctrl Pts',(30.7134539939698,-1.90658020521281,3.79016095005708));
#30440=CARTESIAN_POINT('Ctrl Pts',(30.8323629929647,-3.48565237567683,2.4187862103776));
#30441=CARTESIAN_POINT('Ctrl Pts',(30.9512719919597,-4.21770463967511,0.459657059780211));
#30442=CARTESIAN_POINT('Ctrl Pts',(31.0701809909547,-3.92484741894642,-1.611177020848));
#30443=CARTESIAN_POINT('Ctrl Pts',(31.1890899899496,-2.67824532838493,-3.29048852198293));
#30444=CARTESIAN_POINT('Ctrl Pts',(31.3079989889446,-0.780824962758849,
-4.1702074196749));
#30445=CARTESIAN_POINT('Ctrl Pts',(31.4269079879395,1.30633725444068,-4.03655766520605));
#30446=CARTESIAN_POINT('Ctrl Pts',(31.5458169869345,3.07605722060134,-2.92201779428377));
#30447=CARTESIAN_POINT('Ctrl Pts',(31.6647259859295,4.09828989491981,-1.09742224157957));
#30448=CARTESIAN_POINT('Ctrl Pts',(31.7836349849244,4.12463093940056,0.993848720882264));
#30449=CARTESIAN_POINT('Ctrl Pts',(31.9025439839194,3.14867943729,2.84361276159299));
#30450=CARTESIAN_POINT('Ctrl Pts',(32.0214529829143,1.40759331257097,4.00237388736178));
#30451=CARTESIAN_POINT('Ctrl Pts',(32.1403619819093,-0.675540453973202,
4.18855115831721));
#30452=CARTESIAN_POINT('Ctrl Pts',(32.2592709809043,-2.59451670629275,3.35690314889015));
#30453=CARTESIAN_POINT('Ctrl Pts',(32.3781799798992,-3.88302085140948,1.70952179426543));
#30454=CARTESIAN_POINT('Ctrl Pts',(32.4970889788942,-4.22794412375315,-0.353276354588732));
#30455=CARTESIAN_POINT('Ctrl Pts',(32.6159979778891,-3.54546956353323,-2.33022772913439));
#30456=CARTESIAN_POINT('Ctrl Pts',(32.7349069768841,-2.00143968510732,-3.74092968169653));
#30457=CARTESIAN_POINT('Ctrl Pts',(32.8538159758791,0.0289435448015357,
-4.24257916450323));
#30458=CARTESIAN_POINT('Ctrl Pts',(32.972724974874,2.05229344259103,-3.71327447432861));
#30459=CARTESIAN_POINT('Ctrl Pts',(33.091633973869,3.57693243670117,-2.28163757843869));
#30460=CARTESIAN_POINT('Ctrl Pts',(33.2105429728639,4.23237057927023,-0.295558751907219));
#30461=CARTESIAN_POINT('Ctrl Pts',(33.3294519718589,3.85933525284402,1.76234136938946));
#30462=CARTESIAN_POINT('Ctrl Pts',(33.4483609708539,2.54847469557654,3.39198944899592));
#30463=CARTESIAN_POINT('Ctrl Pts',(33.5672699698489,0.618330320477916,4.19737814723441));
#30464=CARTESIAN_POINT('Ctrl Pts',(33.6861789688438,-1.46206940626736,3.98279659879273));
#30465=CARTESIAN_POINT('Ctrl Pts',(33.8050879678388,-3.18718370466638,2.80038849605003));
#30466=CARTESIAN_POINT('Ctrl Pts',(33.9239969668337,-4.13780677653638,0.937481080421928));
#30467=CARTESIAN_POINT('Ctrl Pts',(34.0429059658287,-4.08293554922066,-1.15323588090632));
#30468=CARTESIAN_POINT('Ctrl Pts',(34.1618149648236,-3.03590382713174,-2.96371450185516));
#30469=CARTESIAN_POINT('Ctrl Pts',(34.2807239638186,-1.25114215390858,-4.05400530424081));
#30470=CARTESIAN_POINT('Ctrl Pts',(34.3996329628135,0.837649255637629,-4.15916571209051));
#30471=CARTESIAN_POINT('Ctrl Pts',(34.5185419618086,2.72289042788497,-3.25364156197822));
#30472=CARTESIAN_POINT('Ctrl Pts',(34.6374509608034,3.94646445364522,-1.55747680952698));
#30473=CARTESIAN_POINT('Ctrl Pts',(34.7563599597985,4.21104070005508,0.517157537486679));
#30474=CARTESIAN_POINT('Ctrl Pts',(34.8752689587934,3.45232667550434,2.46612169644987));
#30475=CARTESIAN_POINT('Ctrl Pts',(34.9941779577884,1.85469121778504,3.8158139607128));
#30476=CARTESIAN_POINT('Ctrl Pts',(35.1130869567833,-0.193637456642115,
4.23825674440386));
#30477=CARTESIAN_POINT('Ctrl Pts',(35.2319959557783,-2.19491188970968,3.63079571065499));
#30478=CARTESIAN_POINT('Ctrl Pts',(35.3509049547733,-3.66281888647431,2.14104495538666));
#30479=CARTESIAN_POINT('Ctrl Pts',(35.4698139537682,-4.24065447386718,0.131016523270486));
#30480=CARTESIAN_POINT('Ctrl Pts',(35.5887229527632,-3.78800359135796,-1.91084915363794));
#30481=CARTESIAN_POINT('Ctrl Pts',(35.7076319517581,-2.41486119677437,-3.48837513699617));
#30482=CARTESIAN_POINT('Ctrl Pts',(35.8265409507531,-0.454903298757822,
-4.21821984785987));
#30483=CARTESIAN_POINT('Ctrl Pts',(35.9454499497481,1.61559689818276,-3.92302974226322));
#30484=CARTESIAN_POINT('Ctrl Pts',(36.064358948743,3.29350421714833,-2.6745365332569));
#30485=CARTESIAN_POINT('Ctrl Pts',(36.183267947738,4.17108423869985,-0.776126258909775));
#30486=CARTESIAN_POINT('Ctrl Pts',(36.3021769467329,4.03508347943329,1.31088405669769));
#30487=CARTESIAN_POINT('Ctrl Pts',(36.4210859457279,2.91855036222394,3.07934724889256));
#30488=CARTESIAN_POINT('Ctrl Pts',(36.5399949447229,1.09280439154274,4.09952366232033));
#30489=CARTESIAN_POINT('Ctrl Pts',(36.6589039437179,-0.998494961682174,
4.12350864041721));
#30490=CARTESIAN_POINT('Ctrl Pts',(36.7778129427128,-2.84715828911907,3.14547379146596));
#30491=CARTESIAN_POINT('Ctrl Pts',(36.8967219417078,-4.0039571619803,1.40308329800038));
#30492=CARTESIAN_POINT('Ctrl Pts',(37.0156309407027,-4.18778742659573,-0.680258896116352));
#30493=CARTESIAN_POINT('Ctrl Pts',(37.1345399396977,-3.35397800645881,-2.59829698616001));
#30494=CARTESIAN_POINT('Ctrl Pts',(37.2534489386926,-1.70514605210925,-3.88494435443889));
#30495=CARTESIAN_POINT('Ctrl Pts',(37.3723579376876,0.358039381572612,-4.22754343529587));
#30496=CARTESIAN_POINT('Ctrl Pts',(37.4912669366826,2.3342206179893,-3.54284205161814));
#30497=CARTESIAN_POINT('Ctrl Pts',(37.6101759356776,3.74318215294784,-1.99722383969792));
#30498=CARTESIAN_POINT('Ctrl Pts',(37.7290849346725,4.24254386394922,0.0337232658201172));
#30499=CARTESIAN_POINT('Ctrl Pts',(37.8479939336675,3.71095997990038,2.05647555874971));
#30500=CARTESIAN_POINT('Ctrl Pts',(37.9669029326624,2.27760631649146,3.57950068621502));
#30501=CARTESIAN_POINT('Ctrl Pts',(38.0858119316574,0.290790325944755,4.23270087345946));
#30502=CARTESIAN_POINT('Ctrl Pts',(38.2047209306524,-1.76668822311588,3.85734732873792));
#30503=CARTESIAN_POINT('Ctrl Pts',(38.3236299296473,-3.39485843815668,2.54465162401958));
#30504=CARTESIAN_POINT('Ctrl Pts',(38.4425389286423,-4.19807210096051,0.613601110964395));
#30505=CARTESIAN_POINT('Ctrl Pts',(38.5614479276372,-3.98114688804759,-1.46655554036626));
#30506=CARTESIAN_POINT('Ctrl Pts',(38.6803569266322,-2.79679599758437,-3.19033663920374));
#30507=CARTESIAN_POINT('Ctrl Pts',(38.7992659256271,-0.932818789330533,
-4.13886031436587));
#30508=CARTESIAN_POINT('Ctrl Pts',(38.9181749246222,1.15783504299492,-4.081633735705));
#30509=CARTESIAN_POINT('Ctrl Pts',(39.037083923617,2.96713288406074,-3.03256289173867));
#30510=CARTESIAN_POINT('Ctrl Pts',(39.1559929226121,4.05541232630964,-1.24657417618181));
#30511=CARTESIAN_POINT('Ctrl Pts',(39.274901921607,4.15821928046345,0.8423347006637));
#30512=CARTESIAN_POINT('Ctrl Pts',(39.393810920602,3.25057202966842,2.72655386816114));
#30513=CARTESIAN_POINT('Ctrl Pts',(39.5127199195969,1.55302934330574,3.94821746331971));
#30514=CARTESIAN_POINT('Ctrl Pts',(39.631628918592,-0.521900729557193,4.21045371123498));
#30515=CARTESIAN_POINT('Ctrl Pts',(39.7505379175868,-2.47001093446444,3.44954947520581));
#30516=CARTESIAN_POINT('Ctrl Pts',(39.8694469165819,-3.81789832054964,1.85038441350672));
#30517=CARTESIAN_POINT('Ctrl Pts',(39.9883559155767,-4.23804135659737,-0.198398866355711));
#30518=CARTESIAN_POINT('Ctrl Pts',(40.1072649145718,-3.62830971000893,-2.19902759642159));
#30519=CARTESIAN_POINT('Ctrl Pts',(40.2261739135667,-2.13693872948098,-3.66517562577142));
#30520=CARTESIAN_POINT('Ctrl Pts',(40.3450829125617,-0.126195570511627,
-4.24090522757565));
#30521=CARTESIAN_POINT('Ctrl Pts',(40.4639919115566,1.91502918549748,-3.78563729041068));
#30522=CARTESIAN_POINT('Ctrl Pts',(40.5829009105516,3.49126579952493,-2.41135070611703));
#30523=CARTESIAN_POINT('Ctrl Pts',(40.7018099095465,4.21838606955971,-0.449310859787289));
#30524=CARTESIAN_POINT('Ctrl Pts',(40.8207189085415,3.92189238888511,1.61834114804089));
#30525=CARTESIAN_POINT('Ctrl Pts',(40.9396279075364,2.66945837179664,3.2998455083566));
#30526=CARTESIAN_POINT('Ctrl Pts',(41.0585369065315,0.774140435187547,4.16543344142367));
#30527=CARTESIAN_POINT('Ctrl Pts',(41.2170822385247,-2.01888746148146,4.0045386084997));
#30528=CARTESIAN_POINT('Ctrl Pts',(41.4152639035163,-4.64876068662433,1.24215893705732));
#30529=CARTESIAN_POINT('Ctrl Pts',(41.6530819015062,-3.55825414784644,-3.23925333460491));
#30530=CARTESIAN_POINT('Ctrl Pts',(41.8512635664978,0.0468156998159277,
-4.48442240866564));
#30531=CARTESIAN_POINT('Ctrl Pts',(42.0098088984911,2.60148746873208,-3.34400839089152));
#30532=CARTESIAN_POINT('Ctrl Pts',(42.1287178974861,3.88717983168713,-1.70435364109129));
#30533=CARTESIAN_POINT('Ctrl Pts',(42.247626896481,4.22697668061874,0.364604063255797));
#30534=CARTESIAN_POINT('Ctrl Pts',(42.366535895476,3.54029074951913,2.33730671702443));
#30535=CARTESIAN_POINT('Ctrl Pts',(42.485444894471,1.99296498656723,3.7458830298263));
#30536=CARTESIAN_POINT('Ctrl Pts',(42.6043538934659,-0.0384826524084342,
4.24227598834855));
#30537=CARTESIAN_POINT('Ctrl Pts',(42.7232628924609,-2.06066523781936,3.70875467629474));
#30538=CARTESIAN_POINT('Ctrl Pts',(42.8421718914558,-3.58205929234741,2.27351505986046));
#30539=CARTESIAN_POINT('Ctrl Pts',(42.9610808904508,-4.23302835186148,0.28605015977224));
#30540=CARTESIAN_POINT('Ctrl Pts',(43.0799898894457,-3.85535322757791,-1.77104718768459));
#30541=CARTESIAN_POINT('Ctrl Pts',(43.1988988884408,-2.54082596366002,-3.39771592193865));
#30542=CARTESIAN_POINT('Ctrl Pts',(43.3178078874356,-0.608870803793044,
-4.19876433520088));
#30543=CARTESIAN_POINT('Ctrl Pts',(43.4367168864306,1.47103965821834,-3.97949031283073));
#30544=CARTESIAN_POINT('Ctrl Pts',(43.5556258854256,3.19348559196464,-2.79320086151097));
#30545=CARTESIAN_POINT('Ctrl Pts',(43.6745348844206,4.13990858508463,-0.928154848713153));
#30546=CARTESIAN_POINT('Ctrl Pts',(43.7934438834155,4.08032670854032,1.16243248575246));
#30547=CARTESIAN_POINT('Ctrl Pts',(43.9123528824105,3.0292182035071,2.97054765803357));
#30548=CARTESIAN_POINT('Ctrl Pts',(44.0312618814054,1.2420044090019,4.05681405687331));
#30549=CARTESIAN_POINT('Ctrl Pts',(44.1501708804004,-0.847018655558019,
4.15726777299333));
#30550=CARTESIAN_POINT('Ctrl Pts',(44.2690798793954,-2.73021469130703,3.24749801153628));
#30551=CARTESIAN_POINT('Ctrl Pts',(44.3879888783904,-3.94996377718922,1.54858060250118));
#30552=CARTESIAN_POINT('Ctrl Pts',(44.5068978773853,-4.20986473922438,-0.526644637896498));
#30553=CARTESIAN_POINT('Ctrl Pts',(44.6258068763802,-3.44676119221666,-2.47389429282434));
#30554=CARTESIAN_POINT('Ctrl Pts',(44.7447158753752,-1.84608863354493,-3.819983306226));
#30555=CARTESIAN_POINT('Ctrl Pts',(44.8636248743702,0.203186698440704,-4.23780967691975));
#30556=CARTESIAN_POINT('Ctrl Pts',(44.9825338733652,2.20308730674562,-3.62584087029532));
#30557=CARTESIAN_POINT('Ctrl Pts',(45.1014428723601,3.66763383799168,-2.13278637607099));
#30558=CARTESIAN_POINT('Ctrl Pts',(45.2203518713551,4.24093891825145,-0.12146105473511));
#30559=CARTESIAN_POINT('Ctrl Pts',(45.33926087035,3.78368840810334,1.91937951603509));
#30560=CARTESIAN_POINT('Ctrl Pts',(45.458169869345,2.40699498298607,3.49380750011858));
#30561=CARTESIAN_POINT('Ctrl Pts',(45.5770788683399,0.445397558168305,4.21923413800868));
#30562=CARTESIAN_POINT('Ctrl Pts',(45.6959878673349,-1.62443225394642,3.91937948512372));
#30563=CARTESIAN_POINT('Ctrl Pts',(45.8148968663298,-3.29952218115088,2.66710874772735));
#30564=CARTESIAN_POINT('Ctrl Pts',(45.9338058653249,-4.17282243514008,0.766725909885086));
#30565=CARTESIAN_POINT('Ctrl Pts',(46.0527148643198,-4.03211952352997,-1.31997266792431));
#30566=CARTESIAN_POINT('Ctrl Pts',(46.1716238633148,-2.91160450045647,-3.085915573865));
#30567=CARTESIAN_POINT('Ctrl Pts',(46.2905328623097,-1.08356448049494,-4.10197558655686));
#30568=CARTESIAN_POINT('Ctrl Pts',(46.4094418613047,1.00778360743057,-4.12124834203113));
#30569=CARTESIAN_POINT('Ctrl Pts',(46.5283508602997,2.85423851237071,-3.13905052692677));
#30570=CARTESIAN_POINT('Ctrl Pts',(46.6472598592946,4.00710845607509,-1.39405793184905));
#30571=CARTESIAN_POINT('Ctrl Pts',(46.7661688582896,4.18624402154559,0.689693184085104));
#30572=CARTESIAN_POINT('Ctrl Pts',(46.8850778572845,3.34811495239536,2.60584764743572));
#30573=CARTESIAN_POINT('Ctrl Pts',(47.0039868562795,1.6963880814478,3.88877656509363));
#30574=CARTESIAN_POINT('Ctrl Pts',(47.1228958552745,-0.367564066613851,
4.22672596143089));
#30575=CARTESIAN_POINT('Ctrl Pts',(47.2418048542694,-2.34219750224519,3.5375735408011));
#30576=CARTESIAN_POINT('Ctrl Pts',(47.3607138532643,-3.7476728395745,1.98878454932031));
#30577=CARTESIAN_POINT('Ctrl Pts',(47.4796228522594,-4.24245710820207,-0.0432825734617755));
#30578=CARTESIAN_POINT('Ctrl Pts',(47.5985318512543,-3.70631686362458,-2.06483195502968));
#30579=CARTESIAN_POINT('Ctrl Pts',(47.7174408502492,-2.2695351249873,-3.58462355241781));
#30580=CARTESIAN_POINT('Ctrl Pts',(47.8363498492442,-0.281252373079731,
-4.23334534366577));
#30581=CARTESIAN_POINT('Ctrl Pts',(47.9552588482392,1.77537519844767,-3.85335679646156));
#30582=CARTESIAN_POINT('Ctrl Pts',(48.0741678472341,3.40058348498636,-2.53699579379582));
#30583=CARTESIAN_POINT('Ctrl Pts',(48.1930768462292,4.19944402434456,-0.604140366551068));
#30584=CARTESIAN_POINT('Ctrl Pts',(48.311985845224,3.97783230526572,1.47552222866482));
#30585=CARTESIAN_POINT('Ctrl Pts',(48.4308948442191,2.78960036391312,3.19663033611261));
#30586=CARTESIAN_POINT('Ctrl Pts',(48.549803843214,0.923490644693623,4.14095166903249));
#30587=CARTESIAN_POINT('Ctrl Pts',(48.6687128422089,-1.16702891982273,4.07901448837793));
#30588=CARTESIAN_POINT('Ctrl Pts',(48.787621841204,-2.97395841132729,3.02586963760755));
#30589=CARTESIAN_POINT('Ctrl Pts',(48.9065308401988,-4.05821079631214,1.23743316134462));
#30590=CARTESIAN_POINT('Ctrl Pts',(49.0254398391939,-4.15631084481653,-0.851701742020117));
#30591=CARTESIAN_POINT('Ctrl Pts',(49.1443488381888,-3.24442007311038,-2.73387162926461));
#30592=CARTESIAN_POINT('Ctrl Pts',(49.2632578371838,-1.54412953702292,-3.95170591883982));
#30593=CARTESIAN_POINT('Ctrl Pts',(49.3821668361787,0.531387183013984,-4.209268743835));
#30594=CARTESIAN_POINT('Ctrl Pts',(49.5010758351737,2.47777588619694,-3.44397188633769));
#30595=CARTESIAN_POINT('Ctrl Pts',(49.6199848341686,3.82206070614344,-1.84178382408138));
#30596=CARTESIAN_POINT('Ctrl Pts',(49.7388938331636,4.23757807543132,0.207960935586202));
#30597=CARTESIAN_POINT('Ctrl Pts',(49.8578028321586,3.62335654502556,2.20717082341209));
#30598=CARTESIAN_POINT('Ctrl Pts',(49.9767118311535,2.12865302339433,3.6700343325455));
#30599=CARTESIAN_POINT('Ctrl Pts',(50.0956208301485,0.11668308609495,4.24107306629136));
#30600=CARTESIAN_POINT('Ctrl Pts',(50.2145298291435,-1.92364104561195,3.78152361138994));
#30601=CARTESIAN_POINT('Ctrl Pts',(50.3334388281384,-3.49651703165463,2.40305729100861));
#30602=CARTESIAN_POINT('Ctrl Pts',(50.4523478271334,-4.21973325041745,0.440643836776059));
#30603=CARTESIAN_POINT('Ctrl Pts',(50.5712568261283,-3.91754689347067,-1.62884684170996));
#30604=CARTESIAN_POINT('Ctrl Pts',(50.6901658251233,-2.66338977453238,-3.3025248835498));
#30605=CARTESIAN_POINT('Ctrl Pts',(50.8090748241182,-0.762024273055086,
-4.17368358857445));
#30606=CARTESIAN_POINT('Ctrl Pts',(50.9279838231132,1.32451446418683,-4.03062986950608));
#30607=CARTESIAN_POINT('Ctrl Pts',(51.0468928221082,3.08919386154722,-2.90812602092978));
#30608=CARTESIAN_POINT('Ctrl Pts',(51.1658018211032,4.10319374310485,-1.07894246521889));
#30609=CARTESIAN_POINT('Ctrl Pts',(51.2847108200981,4.12011033911056,1.01242602683551));
#30610=CARTESIAN_POINT('Ctrl Pts',(51.4036198190931,3.13583292948141,2.85777316760714));
#30611=CARTESIAN_POINT('Ctrl Pts',(51.522528818088,1.38954256537078,4.00867652393499));
#30612=CARTESIAN_POINT('Ctrl Pts',(51.641437817083,-0.694408965276457,4.18546425093048));
#30613=CARTESIAN_POINT('Ctrl Pts',(51.760346816078,-2.60961812434468,3.34517724353594));
#30614=CARTESIAN_POINT('Ctrl Pts',(51.8792558150729,-3.89068505822652,1.6920054757624));
#30615=CARTESIAN_POINT('Ctrl Pts',(51.9981648140678,-4.22630959520428,-0.372324938733972));
#30616=CARTESIAN_POINT('Ctrl Pts',(52.1170738130629,-3.53493171453767,-2.34618303073278));
#30617=CARTESIAN_POINT('Ctrl Pts',(52.2359828120577,-1.98456277868761,-3.74990797127371));
#30618=CARTESIAN_POINT('Ctrl Pts',(52.3548918110528,0.0480654662789952,
-4.24241179250651));
#30619=CARTESIAN_POINT('Ctrl Pts',(52.4738008100477,2.06899960560041,-3.70397600138038));
#30620=CARTESIAN_POINT('Ctrl Pts',(52.5927098090427,3.58719136626157,-2.26551963910266));
#30621=CARTESIAN_POINT('Ctrl Pts',(52.7116188080376,4.23363316565599,-0.276434037724044));
#30622=CARTESIAN_POINT('Ctrl Pts',(52.8305278070326,3.85140697335228,1.77961681187126));
#30623=CARTESIAN_POINT('Ctrl Pts',(52.9494368060276,2.53305490827344,3.40364917162295));
#30624=CARTESIAN_POINT('Ctrl Pts',(53.0287094720242,1.24412279188,3.93419100583381));
#30625=CARTESIAN_POINT('Ctrl Pts',(53.0683458050225,0.575083413457878,4.02967111779183));
#30626=CARTESIAN_POINT('Ctrl Pts',(30.,2.16858287139687,4.42210505377543));
#30627=CARTESIAN_POINT('Ctrl Pts',(30.,2.2732454182619,4.35954462947136));
#30628=CARTESIAN_POINT('Ctrl Pts',(30.,2.37542044069574,4.2931492164828));
#30629=CARTESIAN_POINT('Ctrl Pts',(30.,2.47486624462474,4.22298839050188));
#30630=CARTESIAN_POINT('Ctrl Pts',(30.,2.59306037040875,4.13960028196972));
#30631=CARTESIAN_POINT('Ctrl Pts',(30.,2.70740050030899,4.05089352415537));
#30632=CARTESIAN_POINT('Ctrl Pts',(30.,2.81758790810149,3.95719317214126));
#30633=CARTESIAN_POINT('Ctrl Pts',(30.,2.88224739785667,3.9022085139803));
#30634=CARTESIAN_POINT('Ctrl Pts',(30.,2.94547615811346,3.84550365503418));
#30635=CARTESIAN_POINT('Ctrl Pts',(30.,3.0072068344334,3.78713968990326));
#30636=CARTESIAN_POINT('Ctrl Pts',(30.,3.05048740679948,3.74621958393636));
#30637=CARTESIAN_POINT('Ctrl Pts',(30.,3.0930314592166,3.70448384550322));
#30638=CARTESIAN_POINT('Ctrl Pts',(30.,3.13481409779582,3.66195276571105));
#30639=CARTESIAN_POINT('Ctrl Pts',(30.,3.15648070225866,3.6398980531661));
#30640=CARTESIAN_POINT('Ctrl Pts',(30.,3.17794569554624,3.61762598377252));
#30641=CARTESIAN_POINT('Ctrl Pts',(30.,3.19918545149066,3.59516091321901));
#30642=CARTESIAN_POINT('Ctrl Pts',(30.,3.29689976460728,3.49180949317459));
#30643=CARTESIAN_POINT('Ctrl Pts',(30.,3.38992792611207,3.38429928307111));
#30644=CARTESIAN_POINT('Ctrl Pts',(30.,3.4779844422932,3.27294397186865));
#30645=CARTESIAN_POINT('Ctrl Pts',(30.,3.56533657345243,3.16247941829234));
#30646=CARTESIAN_POINT('Ctrl Pts',(30.,3.64779665226775,3.048230362205));
#30647=CARTESIAN_POINT('Ctrl Pts',(30.,3.72504020840627,2.93048074794443));
#30648=CARTESIAN_POINT('Ctrl Pts',(30.,3.77864078809121,2.84877234535969));
#30649=CARTESIAN_POINT('Ctrl Pts',(30.,3.82972856206389,2.7653778884916));
#30650=CARTESIAN_POINT('Ctrl Pts',(30.,3.87818055748462,2.6803883971215));
#30651=CARTESIAN_POINT('Ctrl Pts',(30.,3.8882281341706,2.66276397474986));
#30652=CARTESIAN_POINT('Ctrl Pts',(30.,3.89816232090752,2.64507095382542));
#30653=CARTESIAN_POINT('Ctrl Pts',(30.,3.90798195189534,2.62731013620557));
#30654=CARTESIAN_POINT('Ctrl Pts',(30.,3.91756757094579,2.60997257719348));
#30655=CARTESIAN_POINT('Ctrl Pts',(30.,3.92703895771373,2.59257958603053));
#30656=CARTESIAN_POINT('Ctrl Pts',(30.,3.93639534143115,2.57513213522472));
#30657=CARTESIAN_POINT('Ctrl Pts',(30.,3.96367452270595,2.52426289047277));
#30658=CARTESIAN_POINT('Ctrl Pts',(30.,3.98997638010842,2.47293046891162));
#30659=CARTESIAN_POINT('Ctrl Pts',(30.,4.01528229489678,2.42115592843892));
#30660=CARTESIAN_POINT('Ctrl Pts',(30.,4.0761489236766,2.29662607992116));
#30661=CARTESIAN_POINT('Ctrl Pts',(30.,4.13125736838721,2.16953959103647));
#30662=CARTESIAN_POINT('Ctrl Pts',(30.,4.18054374041445,2.04031320922016));
#30663=CARTESIAN_POINT('Ctrl Pts',(30.,4.22997372079626,1.91071029354067));
#30664=CARTESIAN_POINT('Ctrl Pts',(30.,4.27354775694774,1.77895417121864));
#30665=CARTESIAN_POINT('Ctrl Pts',(30.,4.3111501113001,1.6454556625514));
#30666=CARTESIAN_POINT('Ctrl Pts',(30.,4.34817396593327,1.51401098405268));
#30667=CARTESIAN_POINT('Ctrl Pts',(30.,4.37940842315398,1.38087635322608));
#30668=CARTESIAN_POINT('Ctrl Pts',(30.,4.4046931579437,1.24644647155864));
#30669=CARTESIAN_POINT('Ctrl Pts',(30.,4.42089890441132,1.16028632006437));
#30670=CARTESIAN_POINT('Ctrl Pts',(30.,4.43465955561036,1.07359417600813));
#30671=CARTESIAN_POINT('Ctrl Pts',(30.,4.44592197371389,0.986476687916269));
#30672=CARTESIAN_POINT('Ctrl Pts',(30.,4.44839086637678,0.967379214781952));
#30673=CARTESIAN_POINT('Ctrl Pts',(30.,4.45073967281179,0.948261313176081));
#30674=CARTESIAN_POINT('Ctrl Pts',(30.,4.45296777758924,0.929124127526741));
#30675=CARTESIAN_POINT('Ctrl Pts',(30.,4.45503255715034,0.911389741700035));
#30676=CARTESIAN_POINT('Ctrl Pts',(30.,4.45699251705267,0.893648784711569));
#30677=CARTESIAN_POINT('Ctrl Pts',(30.,4.45884747035307,0.875902588838401));
#30678=CARTESIAN_POINT('Ctrl Pts',(30.,4.47288215368143,0.741633850477624));
#30679=CARTESIAN_POINT('Ctrl Pts',(30.,4.4809109307611,0.607056772754871));
#30680=CARTESIAN_POINT('Ctrl Pts',(30.,4.48284622078689,0.472553103246923));
#30681=CARTESIAN_POINT('Ctrl Pts',(30.,4.4841564920511,0.381488564733919));
#30682=CARTESIAN_POINT('Ctrl Pts',(30.,4.48267253782096,0.290457568449046));
#30683=CARTESIAN_POINT('Ctrl Pts',(30.,4.47835364427375,0.199579870531098));
#30684=CARTESIAN_POINT('Ctrl Pts',(30.,4.47194672265211,0.0647661083135189));
#30685=CARTESIAN_POINT('Ctrl Pts',(30.,4.45930307443608,-0.0697114630799221));
#30686=CARTESIAN_POINT('Ctrl Pts',(30.,4.44051793519591,-0.203434213073621));
#30687=CARTESIAN_POINT('Ctrl Pts',(30.,4.42188441330993,-0.336077668988553));
#30688=CARTESIAN_POINT('Ctrl Pts',(30.,4.39720776531948,-0.467979164954463));
#30689=CARTESIAN_POINT('Ctrl Pts',(30.,4.36653661631927,-0.598704850027088));
#30690=CARTESIAN_POINT('Ctrl Pts',(30.,4.35826921191622,-0.633941942199734));
#30691=CARTESIAN_POINT('Ctrl Pts',(30.,4.34956603093133,-0.669093426449049));
#30692=CARTESIAN_POINT('Ctrl Pts',(30.,4.34042752155899,-0.704150383578858));
#30693=CARTESIAN_POINT('Ctrl Pts',(30.,4.33455297624871,-0.726686190536959));
#30694=CARTESIAN_POINT('Ctrl Pts',(30.,4.32849853352323,-0.749182931588532));
#30695=CARTESIAN_POINT('Ctrl Pts',(30.,4.32226426812988,-0.771638192356437));
#30696=CARTESIAN_POINT('Ctrl Pts',(30.,4.31754067405252,-0.788652151512211));
#30697=CARTESIAN_POINT('Ctrl Pts',(30.,4.31271393090463,-0.80564179080815));
#30698=CARTESIAN_POINT('Ctrl Pts',(30.,4.3077879772602,-0.822593202800587));
#30699=CARTESIAN_POINT('Ctrl Pts',(30.,4.27100671946256,-0.949166512160226));
#30700=CARTESIAN_POINT('Ctrl Pts',(30.,4.22864672526021,-1.07379766426646));
#30701=CARTESIAN_POINT('Ctrl Pts',(30.,4.1808305106355,-1.19610739677557));
#30702=CARTESIAN_POINT('Ctrl Pts',(30.,4.13354228297351,-1.31706658439766));
#30703=CARTESIAN_POINT('Ctrl Pts',(30.,4.08091725186588,-1.43575600239369));
#30704=CARTESIAN_POINT('Ctrl Pts',(30.,4.02303011908695,-1.55178410876982));
#30705=CARTESIAN_POINT('Ctrl Pts',(30.,3.96819820087205,-1.66168838859898));
#30706=CARTESIAN_POINT('Ctrl Pts',(30.,3.90864442065182,-1.76920516529743));
#30707=CARTESIAN_POINT('Ctrl Pts',(30.,3.84440013420362,-1.87397285765276));
#30708=CARTESIAN_POINT('Ctrl Pts',(30.,3.79893603048459,-1.94811438050221));
#30709=CARTESIAN_POINT('Ctrl Pts',(30.,3.75112211275763,-2.02087850788643));
#30710=CARTESIAN_POINT('Ctrl Pts',(30.,3.70103315780837,-2.09216345552501));
#30711=CARTESIAN_POINT('Ctrl Pts',(30.,3.67453247022062,-2.12987835951916));
#30712=CARTESIAN_POINT('Ctrl Pts',(30.,3.64739487281119,-2.16717906849915));
#30713=CARTESIAN_POINT('Ctrl Pts',(30.,3.61963092738038,-2.20404946355424));
#30714=CARTESIAN_POINT('Ctrl Pts',(30.,3.60474871618731,-2.22381297329565));
#30715=CARTESIAN_POINT('Ctrl Pts',(30.,3.58968653441096,-2.24345283054055));
#30716=CARTESIAN_POINT('Ctrl Pts',(30.,3.57444597381909,-2.26296646152855));
#30717=CARTESIAN_POINT('Ctrl Pts',(30.,3.56382219475439,-2.27656888140787));
#30718=CARTESIAN_POINT('Ctrl Pts',(30.,3.55311488934063,-2.29010588184238));
#30719=CARTESIAN_POINT('Ctrl Pts',(30.,3.54232950699003,-2.30357088580617));
#30720=CARTESIAN_POINT('Ctrl Pts',(30.,3.46063422988411,-2.40556330427549));
#30721=CARTESIAN_POINT('Ctrl Pts',(30.,3.37438073686154,-2.50353329208469));
#30722=CARTESIAN_POINT('Ctrl Pts',(30.,3.28388555158297,-2.59720218594732));
#30723=CARTESIAN_POINT('Ctrl Pts',(30.,3.19548605035865,-2.68870189913318));
#30724=CARTESIAN_POINT('Ctrl Pts',(30.,3.10303822337506,-2.77609776168811));
#30725=CARTESIAN_POINT('Ctrl Pts',(30.,3.00680578566741,-2.85908852120383));
#30726=CARTESIAN_POINT('Ctrl Pts',(30.,2.90715127912884,-2.94503046950951));
#30727=CARTESIAN_POINT('Ctrl Pts',(30.,2.80343761470821,-3.02624930319516));
#30728=CARTESIAN_POINT('Ctrl Pts',(30.,2.69593400653002,-3.10235578897998));
#30729=CARTESIAN_POINT('Ctrl Pts',(30.,2.59557657777575,-3.17340318314957));
#30730=CARTESIAN_POINT('Ctrl Pts',(30.,2.49191560602939,-3.23999516173219));
#30731=CARTESIAN_POINT('Ctrl Pts',(30.,2.38515991446318,-3.30176482420669));
#30732=CARTESIAN_POINT('Ctrl Pts',(30.,2.37755813215443,-3.3061632737931));
#30733=CARTESIAN_POINT('Ctrl Pts',(30.,2.36994065609269,-3.3105372499843));
#30734=CARTESIAN_POINT('Ctrl Pts',(30.,2.36230756092333,-3.31488661006745));
#30735=CARTESIAN_POINT('Ctrl Pts',(52.575,0.695807839646318,4.87560011181051));
#30736=CARTESIAN_POINT('Ctrl Pts',(52.5353636670017,1.50529535683805,4.76007633060593));
#30737=CARTESIAN_POINT('Ctrl Pts',(52.4957273340033,2.28505099782045,4.439118397491));
#30738=CARTESIAN_POINT('Ctrl Pts',(52.456091001005,2.94078002088763,3.95114651967049));
#30739=CARTESIAN_POINT('Ctrl Pts',(52.4164546680067,3.5965090439548,3.46317464184999));
#30740=CARTESIAN_POINT('Ctrl Pts',(52.3768183350084,4.12821144910675,2.80818881932393));
#30741=CARTESIAN_POINT('Ctrl Pts',(52.3371820020101,4.47114016046936,2.06608466315826));
#30742=CARTESIAN_POINT('Ctrl Pts',(52.2975456690118,4.81406887183195,1.3239805069926));
#30743=CARTESIAN_POINT('Ctrl Pts',(52.2579093360134,4.96822388940519,0.494758017187346));
#30744=CARTESIAN_POINT('Ctrl Pts',(52.2182730030151,4.91494370822671,-0.320960650504854));
#30745=CARTESIAN_POINT('Ctrl Pts',(52.1786366700168,4.86166352704823,-1.13667931819705));
#30746=CARTESIAN_POINT('Ctrl Pts',(52.1390003370185,4.60094814711803,-1.93889416377618));
#30747=CARTESIAN_POINT('Ctrl Pts',(52.0993640040202,4.16444074494492,-2.63007232252029));
#30748=CARTESIAN_POINT('Ctrl Pts',(52.0597276710218,3.72793334277182,-3.32125048126438));
#30749=CARTESIAN_POINT('Ctrl Pts',(52.0200913380235,3.11563391835576,-3.90139195317348));
#30750=CARTESIAN_POINT('Ctrl Pts',(51.9804550050252,2.40195439260487,-4.30004051622935));
#30751=CARTESIAN_POINT('Ctrl Pts',(51.9408186720269,1.68827486685394,-4.69868907928524));
#30752=CARTESIAN_POINT('Ctrl Pts',(51.9011823390286,0.873215239768212,-4.91584473348791));
#30753=CARTESIAN_POINT('Ctrl Pts',(51.8615460060302,0.0557974474159643,
-4.9251071071408));
#30754=CARTESIAN_POINT('Ctrl Pts',(51.8219096730319,-0.76162034493626,-4.93436948079368));
#30755=CARTESIAN_POINT('Ctrl Pts',(51.7822733400336,-1.58139630255493,-4.73573857389677));
#30756=CARTESIAN_POINT('Ctrl Pts',(51.7426370070352,-2.30392265539945,-4.3533561208101));
#30757=CARTESIAN_POINT('Ctrl Pts',(51.7030006740369,-3.02644900824399,-3.97097366772342));
#30758=CARTESIAN_POINT('Ctrl Pts',(51.6633643410386,-3.65172575631444,-3.40483966844693));
#30759=CARTESIAN_POINT('Ctrl Pts',(51.6237280080403,-4.1037833688659,-2.72373593691276));
#30760=CARTESIAN_POINT('Ctrl Pts',(51.584091675042,-4.55584098141733,-2.04263220537863));
#30761=CARTESIAN_POINT('Ctrl Pts',(51.5444553420437,-4.83467945844985,-1.24655874158681));
#30762=CARTESIAN_POINT('Ctrl Pts',(51.5048190090453,-4.90641860669811,-0.432241155930334));
#30763=CARTESIAN_POINT('Ctrl Pts',(51.4978265146648,-4.91907456029036,-0.288582277548382));
#30764=CARTESIAN_POINT('Ctrl Pts',(51.4908340202842,-4.92528502287894,-0.14435559277112));
#30765=CARTESIAN_POINT('Ctrl Pts',(51.4838415259036,-4.9251402971202,-0.000116503725961781));
#30766=CARTESIAN_POINT('Origin',(41.25,0.,0.));
#30767=CARTESIAN_POINT('Origin',(52.575,0.,0.));
#30768=CARTESIAN_POINT('Ctrl Pts',(-53.0683458050225,-1.79217368492195,
3.65473442716065));
#30769=CARTESIAN_POINT('Ctrl Pts',(-53.0287094720242,-2.39896296820851,
3.35718290666791));
#30770=CARTESIAN_POINT('Ctrl Pts',(-52.9494368060276,-3.46086376985422,
2.45430560800941));
#30771=CARTESIAN_POINT('Ctrl Pts',(-52.8305278070326,-4.21283755893848,
0.502366005806227));
#30772=CARTESIAN_POINT('Ctrl Pts',(-52.7116188080376,-3.94100158787114,
-1.57116901649836));
#30773=CARTESIAN_POINT('Ctrl Pts',(-52.5927098090427,-2.71153766019247,
-3.26314029666967));
#30774=CARTESIAN_POINT('Ctrl Pts',(-52.4738008100477,-0.823144024575674,
-4.16204656282918));
#30775=CARTESIAN_POINT('Ctrl Pts',(-52.3548918110528,1.26526436602798,-4.04962642367063));
#30776=CARTESIAN_POINT('Ctrl Pts',(-52.2359828120578,3.04621665534188,-2.95311079097194));
#30777=CARTESIAN_POINT('Ctrl Pts',(-52.1170738130628,4.08693027247079,-1.13899868529834));
#30778=CARTESIAN_POINT('Ctrl Pts',(-51.9981648140679,4.13451401645655,0.951899429035897));
#30779=CARTESIAN_POINT('Ctrl Pts',(-51.8792558150729,3.17740293277235,2.81148063819688));
#30780=CARTESIAN_POINT('Ctrl Pts',(-51.760346816078,1.44817770563431,3.98786896704909));
#30781=CARTESIAN_POINT('Ctrl Pts',(-51.641437817083,-0.632957411871854,
4.19519722352873));
#30782=CARTESIAN_POINT('Ctrl Pts',(-51.522528818088,-2.56028268385088,3.38308566467023));
#30783=CARTESIAN_POINT('Ctrl Pts',(-51.403619819093,-3.86545481878031,1.74887812750191));
#30784=CARTESIAN_POINT('Ctrl Pts',(-51.2847108200981,-4.23131463624997,
-0.310309743601171));
#30785=CARTESIAN_POINT('Ctrl Pts',(-51.1658018211031,-3.56895759144185,
-2.29409186145612));
#30786=CARTESIAN_POINT('Ctrl Pts',(-51.0468928221082,-2.03933759109846,
-3.72040560679174));
#30787=CARTESIAN_POINT('Ctrl Pts',(-50.9279838231133,-0.0141549843878351,
-4.24265428344519));
#30788=CARTESIAN_POINT('Ctrl Pts',(-50.8090748241182,2.01446730968869,-3.73393052561418));
#30789=CARTESIAN_POINT('Ctrl Pts',(-50.6901658251233,3.55357051600268,-2.31785510914493));
#30790=CARTESIAN_POINT('Ctrl Pts',(-50.5712568261283,4.22914985879238,-0.338536836715756));
#30791=CARTESIAN_POINT('Ctrl Pts',(-50.4523478271334,3.87703837313768,1.72304647947545));
#30792=CARTESIAN_POINT('Ctrl Pts',(-50.3334388281384,2.58279976746683,3.36592648157085));
#30793=CARTESIAN_POINT('Ctrl Pts',(-50.2145298291435,0.660936291289855,
4.19088044882765));
#30794=CARTESIAN_POINT('Ctrl Pts',(-50.0956208301485,-1.42153586209668,
3.99744312162439));
#30795=CARTESIAN_POINT('Ctrl Pts',(-49.9767118311536,-3.15857230942583,
2.83262010934112));
#30796=CARTESIAN_POINT('Ctrl Pts',(-49.8578028321586,-4.1280701494123,0.979465445678941));
#30797=CARTESIAN_POINT('Ctrl Pts',(-49.7388938331636,-4.09443970767262,
-1.11170103804332));
#30798=CARTESIAN_POINT('Ctrl Pts',(-49.6199848341687,-3.06585324049081,
-2.93272222099405));
#30799=CARTESIAN_POINT('Ctrl Pts',(-49.5010758351736,-1.29225906223574,
-4.04108676395591));
#30800=CARTESIAN_POINT('Ctrl Pts',(-49.3821668361788,0.795356333133346,
-4.167460140312));
#30801=CARTESIAN_POINT('Ctrl Pts',(-49.2632578371837,2.68969874550031,-3.28113339811124));
#30802=CARTESIAN_POINT('Ctrl Pts',(-49.1443488381888,3.93043964837605,-1.59748548920479));
#30803=CARTESIAN_POINT('Ctrl Pts',(-49.0254398391938,4.216076827669,0.474354193550262));
#30804=CARTESIAN_POINT('Ctrl Pts',(-48.9065308401989,3.47719994816421,2.43092497585451));
#30805=CARTESIAN_POINT('Ctrl Pts',(-48.7876218412039,1.89335738663818,3.79677672825371));
#30806=CARTESIAN_POINT('Ctrl Pts',(-48.6687128422089,-0.150574338398622,
4.24000508093589));
#30807=CARTESIAN_POINT('Ctrl Pts',(-48.549803843214,-2.15791623528735,3.65290476733649));
#30808=CARTESIAN_POINT('Ctrl Pts',(-48.430894844219,-3.64088070474142,2.17814219269265));
#30809=CARTESIAN_POINT('Ctrl Pts',(-48.3119858452241,-4.23910478143669,
0.174087247513894));
#30810=CARTESIAN_POINT('Ctrl Pts',(-48.1930768462291,-3.80721896620666,
-1.87227120393991));
#30811=CARTESIAN_POINT('Ctrl Pts',(-48.0741678472342,-2.45017226913454,
-3.46366447123714));
#30812=CARTESIAN_POINT('Ctrl Pts',(-47.9552588482392,-0.497729416154917,
-4.21338120113056));
#30813=CARTESIAN_POINT('Ctrl Pts',(-47.8363498492442,1.57566255733915,-3.93923891419978));
#30814=CARTESIAN_POINT('Ctrl Pts',(-47.7174408502492,3.26616576767762,-2.70785466666829));
#30815=CARTESIAN_POINT('Ctrl Pts',(-47.5985318512543,4.16298497174054,-0.818456988979114));
#30816=CARTESIAN_POINT('Ctrl Pts',(-47.4796228522594,4.04819153105236,1.26982717157192));
#30817=CARTESIAN_POINT('Ctrl Pts',(-47.3607138532644,2.94968045290301,3.04954110375778));
#30818=CARTESIAN_POINT('Ctrl Pts',(-47.2418048542694,1.13439185468392,4.08821120268671));
#30819=CARTESIAN_POINT('Ctrl Pts',(-47.1228958552744,-0.956555952514039,
4.13343881380338));
#30820=CARTESIAN_POINT('Ctrl Pts',(-47.0039868562795,-2.81505898666,3.17423354833433));
#30821=CARTESIAN_POINT('Ctrl Pts',(-46.8850778572845,-3.9894977529893,1.44368396702315));
#30822=CARTESIAN_POINT('Ctrl Pts',(-46.7661688582896,-4.19448157280151,
-0.637683348673077));
#30823=CARTESIAN_POINT('Ctrl Pts',(-46.6472598592946,-3.38019901859953,
-2.5640924929505));
#30824=CARTESIAN_POINT('Ctrl Pts',(-46.5283508602997,-1.74452217827771,
-3.8674226672609));
#30825=CARTESIAN_POINT('Ctrl Pts',(-46.4094418613047,0.315076609054344,
-4.23096235485186));
#30826=CARTESIAN_POINT('Ctrl Pts',(-46.2905328623097,2.29811122813968,-3.56637077444897));
#30827=CARTESIAN_POINT('Ctrl Pts',(-46.1716238633148,3.72270079080243,-2.03514484494512));
#30828=CARTESIAN_POINT('Ctrl Pts',(-46.0527148643198,4.2426675363842,-0.00937515104479359));
#30829=CARTESIAN_POINT('Ctrl Pts',(-45.9338058653248,3.7316586343443,2.01867272098968));
#30830=CARTESIAN_POINT('Ctrl Pts',(-45.8148968663299,2.31385014354139,3.5561795836249));
#30831=CARTESIAN_POINT('Ctrl Pts',(-45.6959878673349,0.333772012288686,
4.22952857438387));
#30832=CARTESIAN_POINT('Ctrl Pts',(-45.57707886834,-1.7274133029682,3.87509470833104));
#30833=CARTESIAN_POINT('Ctrl Pts',(-45.458169869345,-3.36883415789558,2.57900603610148));
#30834=CARTESIAN_POINT('Ctrl Pts',(-45.33926087035,-4.19162240778749,0.656214376839717));
#30835=CARTESIAN_POINT('Ctrl Pts',(-45.2203518713551,-3.99583906574759,
-1.42603852628503));
#30836=CARTESIAN_POINT('Ctrl Pts',(-45.1014428723601,-2.82905982713036,
-3.16176156781322));
#30837=CARTESIAN_POINT('Ctrl Pts',(-44.9825338733652,-0.974814091813329,
-4.12917100710215));
#30838=CARTESIAN_POINT('Ctrl Pts',(-44.8636248743702,1.11631317618967,-4.09318465336435));
#30839=CARTESIAN_POINT('Ctrl Pts',(-44.7447158753752,2.93617438620888,-3.06254725647695));
#30840=CARTESIAN_POINT('Ctrl Pts',(-44.6258068763803,4.04254007317222,-1.28770550464645));
#30841=CARTESIAN_POINT('Ctrl Pts',(-44.5068978773853,4.16656143857104,0.800050934283993));
#30842=CARTESIAN_POINT('Ctrl Pts',(-44.3879888783903,3.27810106806685,2.69339360894175));
#30843=CARTESIAN_POINT('Ctrl Pts',(-44.2690798793954,1.59305639924211,3.93223688581989));
#30844=CARTESIAN_POINT('Ctrl Pts',(-44.1501708804004,-0.479103780509667,
4.21553976710139));
#30845=CARTESIAN_POINT('Ctrl Pts',(-44.0312618814054,-2.4348408745219,3.47445897688703));
#30846=CARTESIAN_POINT('Ctrl Pts',(-43.9123528824105,-3.79890742291198,
1.88907880356681));
#30847=CARTESIAN_POINT('Ctrl Pts',(-43.7934438834155,-4.23983270028836,
-0.155351305015692));
#30848=CARTESIAN_POINT('Ctrl Pts',(-43.6745348844206,-3.65047141713449,
-2.16202982679776));
#30849=CARTESIAN_POINT('Ctrl Pts',(-43.5556258854256,-2.17403874853064,
-3.64333320102936));
#30850=CARTESIAN_POINT('Ctrl Pts',(-43.4367168864307,-0.169311716792706,
-4.23929645182126));
#30851=CARTESIAN_POINT('Ctrl Pts',(-43.3178078874356,1.87656008092686,-3.80511075431245));
#30852=CARTESIAN_POINT('Ctrl Pts',(-43.1988988884407,3.46642105478168,-2.44626147372541));
#30853=CARTESIAN_POINT('Ctrl Pts',(-43.0799898894457,4.21394248881074,-0.492996289805673));
#30854=CARTESIAN_POINT('Ctrl Pts',(-42.9610808904508,3.9374548435202,1.58012754509629));
#30855=CARTESIAN_POINT('Ctrl Pts',(-42.8421718914559,2.70418603569597,3.26915855205306));
#30856=CARTESIAN_POINT('Ctrl Pts',(-42.7232628924609,0.813740892457039,
4.16401580837881));
#30857=CARTESIAN_POINT('Ctrl Pts',(-42.6043538934659,-1.2743362201606,4.04653615170507));
#30858=CARTESIAN_POINT('Ctrl Pts',(-42.485444894471,-3.05296381848078,2.94668618241789));
#30859=CARTESIAN_POINT('Ctrl Pts',(-42.366535895476,-4.08928414300699,1.12890118224142));
#30860=CARTESIAN_POINT('Ctrl Pts',(-42.247626896481,-4.13276248524086,-0.959449239315854));
#30861=CARTESIAN_POINT('Ctrl Pts',(-42.1287178974861,-3.17025358567157,
-2.82214018180611));
#30862=CARTESIAN_POINT('Ctrl Pts',(-42.0098088984911,-1.44080606975949,
-3.98424622002752));
#30863=CARTESIAN_POINT('Ctrl Pts',(-41.8512635664978,1.34123824569469,-4.27940453375867));
#30864=CARTESIAN_POINT('Ctrl Pts',(-41.6530819015062,4.38508519896316,-1.98115288915087));
#30865=CARTESIAN_POINT('Ctrl Pts',(-41.4152639035164,4.03738586191726,2.61791030678041));
#30866=CARTESIAN_POINT('Ctrl Pts',(-41.2170822385246,0.682605700869055,
4.43241160683543));
#30867=CARTESIAN_POINT('Ctrl Pts',(-41.0585369065315,-2.02344112387514,
3.7223414795892));
#30868=CARTESIAN_POINT('Ctrl Pts',(-40.9396279075364,-3.55851407251,2.3134304828493));
#30869=CARTESIAN_POINT('Ctrl Pts',(-40.8207189085415,-4.23003625048233,
0.327203181285681));
#30870=CARTESIAN_POINT('Ctrl Pts',(-40.7018099095465,-3.87307886616663,
-1.73087341477296));
#30871=CARTESIAN_POINT('Ctrl Pts',(-40.5829009105516,-2.57524274258496,
-3.37219103126866));
#30872=CARTESIAN_POINT('Ctrl Pts',(-40.4639919115566,-0.651474730133847,
-4.1921317137068));
#30873=CARTESIAN_POINT('Ctrl Pts',(-40.3450829125617,1.43053090860402,-3.99434390257198));
#30874=CARTESIAN_POINT('Ctrl Pts',(-40.2261739135667,3.1649510603171,-2.82543882253934));
#30875=CARTESIAN_POINT('Ctrl Pts',(-40.1072649145718,4.13026449432683,-0.970190141382548));
#30876=CARTESIAN_POINT('Ctrl Pts',(-39.9883559155767,4.09192547196896,1.12093825548876));
#30877=CARTESIAN_POINT('Ctrl Pts',(-39.8694469165819,3.0592368484789,2.93961562653621));
#30878=CARTESIAN_POINT('Ctrl Pts',(-39.7505379175868,1.28315058440506,4.04399186048308));
#30879=CARTESIAN_POINT('Ctrl Pts',(-39.6316289185919,-0.804744661503545,
4.16565563790974));
#30880=CARTESIAN_POINT('Ctrl Pts',(-39.5127199195969,-2.69708497226697,
3.27506548731581));
#30881=CARTESIAN_POINT('Ctrl Pts',(-39.393810920602,-3.93402919418496,1.58862482625052));
#30882=CARTESIAN_POINT('Ctrl Pts',(-39.274901921607,-4.21499728287336,-0.48385251861988));
#30883=CARTESIAN_POINT('Ctrl Pts',(-39.155992922612,-3.47171371609164,-2.43875382264022));
#30884=CARTESIAN_POINT('Ctrl Pts',(-39.0370839236171,-1.88479759517879,
-3.80103318737441));
#30885=CARTESIAN_POINT('Ctrl Pts',(-38.9181749246221,0.160127626810078,
-4.23965506894654));
#30886=CARTESIAN_POINT('Ctrl Pts',(-38.7992659256272,2.16614156389975,-3.64803321565397));
#30887=CARTESIAN_POINT('Ctrl Pts',(-38.6803569266322,3.6457792997346,-2.16993295812935));
#30888=CARTESIAN_POINT('Ctrl Pts',(-38.5614479276372,4.23948627792256,-0.164535157769628));
#30889=CARTESIAN_POINT('Ctrl Pts',(-38.4425389286423,3.80299065872691,1.88084495893092));
#30890=CARTESIAN_POINT('Ctrl Pts',(-38.3236299296473,2.44236164439116,3.46917646169672));
#30891=CARTESIAN_POINT('Ctrl Pts',(-38.2047209306524,0.488234469363121,
4.21449199984978));
#30892=CARTESIAN_POINT('Ctrl Pts',(-38.0858119316573,-1.58453453732273,
3.93567859708109));
#30893=CARTESIAN_POINT('Ctrl Pts',(-37.9669029326625,-3.27225887423897,
2.70048839604023));
#30894=CARTESIAN_POINT('Ctrl Pts',(-37.8479939336674,-4.16481856926941,
0.809074782002492));
#30895=CARTESIAN_POINT('Ctrl Pts',(-37.7290849346726,-4.04532005215358,
-1.2789454224014));
#30896=CARTESIAN_POINT('Ctrl Pts',(-37.6101759356775,-2.94280167197283,
-3.05617964738425));
#30897=CARTESIAN_POINT('Ctrl Pts',(-37.4912669366826,-1.12517732754963,
-4.09075686143469));
#30898=CARTESIAN_POINT('Ctrl Pts',(-37.3723579376876,0.965867079610468,
-4.13127298810448));
#30899=CARTESIAN_POINT('Ctrl Pts',(-37.2534489386927,2.82220409351303,-3.1678825376449));
#30900=CARTESIAN_POINT('Ctrl Pts',(-37.1345399396977,3.99274056611069,-1.43469107806466));
#30901=CARTESIAN_POINT('Ctrl Pts',(-37.0156309407027,4.19303408291871,0.647132828117663));
#30902=CARTESIAN_POINT('Ctrl Pts',(-36.8967219417077,3.37441296829128,2.57170232281563));
#30903=CARTESIAN_POINT('Ctrl Pts',(-36.7778129427128,1.73580358791025,3.87134364555039));
#30904=CARTESIAN_POINT('Ctrl Pts',(-36.6589039437178,-0.324609106740258,
4.23024167696931));
#30905=CARTESIAN_POINT('Ctrl Pts',(-36.5399949447229,-2.3061412194985,3.56118356638298));
#30906=CARTESIAN_POINT('Ctrl Pts',(-36.4210859457279,-3.72727697385935,
2.02675160734717));
#30907=CARTESIAN_POINT('Ctrl Pts',(-36.302176946733,-4.24267789063578,-0.00018454463676528));
#30908=CARTESIAN_POINT('Ctrl Pts',(-36.183267947738,-3.72710064368882,-2.02707585195046));
#30909=CARTESIAN_POINT('Ctrl Pts',(-36.064358948743,-2.30583140769797,-3.56138417430919));
#30910=CARTESIAN_POINT('Ctrl Pts',(-35.9454499497481,-0.324241098120267,
-4.23026990014066));
#30911=CARTESIAN_POINT('Ctrl Pts',(-35.8265409507531,1.73614036661006,-3.87119262568701));
#30912=CARTESIAN_POINT('Ctrl Pts',(-35.7076319517581,3.37463667925653,-2.5714087580085));
#30913=CARTESIAN_POINT('Ctrl Pts',(-35.5887229527632,4.19309036399278,-0.646768055130456));
#30914=CARTESIAN_POINT('Ctrl Pts',(-35.4698139537682,3.99261574089381,1.43503841875865));
#30915=CARTESIAN_POINT('Ctrl Pts',(-35.3509049547733,2.82192849475196,3.16812804164435));
#30916=CARTESIAN_POINT('Ctrl Pts',(-35.2319959557783,0.96550767828667,4.13135699751496));
#30917=CARTESIAN_POINT('Ctrl Pts',(-35.1130869567833,-1.12553319628343,
4.09065896180682));
#30918=CARTESIAN_POINT('Ctrl Pts',(-34.9941779577884,-2.94306753139286,
3.05592362852992));
#30919=CARTESIAN_POINT('Ctrl Pts',(-34.8752689587934,-4.04543129795022,
1.27859349728957));
#30920=CARTESIAN_POINT('Ctrl Pts',(-34.7563599597985,-4.16474816852819,
-0.809437094830369));
#30921=CARTESIAN_POINT('Ctrl Pts',(-34.6374509608035,-3.27202393444525,
-2.70077305417611));
#30922=CARTESIAN_POINT('Ctrl Pts',(-34.5185419618086,-1.5841921492944,-3.93581642761199));
#30923=CARTESIAN_POINT('Ctrl Pts',(-34.3996329628135,0.488601104807327,
-4.21444951068671));
#30924=CARTESIAN_POINT('Ctrl Pts',(-34.2807239638187,2.44266343405159,-3.46896397584259));
#30925=CARTESIAN_POINT('Ctrl Pts',(-34.1618149648236,3.80315426747452,-1.88051411468693));
#30926=CARTESIAN_POINT('Ctrl Pts',(-34.0429059658287,4.2394719479716,0.164903972384525));
#30927=CARTESIAN_POINT('Ctrl Pts',(-33.9239969668337,3.64559051443191,2.17025010513313));
#30928=CARTESIAN_POINT('Ctrl Pts',(-33.8050879678388,2.1658241961235,3.64822165845675));
#30929=CARTESIAN_POINT('Ctrl Pts',(-33.6861789688438,0.159758802036821,
4.23966895440156));
#30930=CARTESIAN_POINT('Ctrl Pts',(-33.5672699698489,-1.88512826096029,
3.80086926340264));
#30931=CARTESIAN_POINT('Ctrl Pts',(-33.4483609708539,-3.47192585240921,
2.43845167947057));
#30932=CARTESIAN_POINT('Ctrl Pts',(-33.3294519718589,-4.21503937635071,
0.483486063466008));
#30933=CARTESIAN_POINT('Ctrl Pts',(-33.210542972864,-3.93389094398069,-1.58896751339184));
#30934=CARTESIAN_POINT('Ctrl Pts',(-33.091633973869,-2.69680011715167,-3.27529919943904));
#30935=CARTESIAN_POINT('Ctrl Pts',(-32.9727249748741,-0.804382135063499,
-4.16572743931235));
#30936=CARTESIAN_POINT('Ctrl Pts',(-32.853815975879,1.28350211569609,-4.04387660995158));
#30937=CARTESIAN_POINT('Ctrl Pts',(-32.7349069768842,3.05949310273849,-2.93935667663218));
#30938=CARTESIAN_POINT('Ctrl Pts',(-32.6159979778891,4.09202190325118,-1.12056791874808));
#30939=CARTESIAN_POINT('Ctrl Pts',(-32.4970889788942,4.13018220918936,0.970520807006677));
#30940=CARTESIAN_POINT('Ctrl Pts',(-32.3781799798992,3.16470099886364,2.82577127648086));
#30941=CARTESIAN_POINT('Ctrl Pts',(-32.2592709809043,1.43019189953828,3.99435437116099));
#30942=CARTESIAN_POINT('Ctrl Pts',(-32.1403619819093,-0.651856339348117,
4.19230235613684));
#30943=CARTESIAN_POINT('Ctrl Pts',(-32.0214529829143,-2.57550234280079,
3.37151351350433));
#30944=CARTESIAN_POINT('Ctrl Pts',(-31.9025439839194,-3.87329676764037,
1.73144099180317));
#30945=CARTESIAN_POINT('Ctrl Pts',(-31.7836349849244,-4.22987327936596,
-0.329374753772751));
#30946=CARTESIAN_POINT('Ctrl Pts',(-31.6647259859294,-3.55858318971203,
-2.31015180080996));
#30947=CARTESIAN_POINT('Ctrl Pts',(-31.5458169869345,-2.02255110907419,
-3.72955802299772));
#30948=CARTESIAN_POINT('Ctrl Pts',(-31.4269079879395,0.00496435902457082,
-4.24267488557468));
#30949=CARTESIAN_POINT('Ctrl Pts',(-31.3079989889446,2.03127363286532,-3.72481475967269));
#30950=CARTESIAN_POINT('Ctrl Pts',(-31.1890899899496,3.56397954706214,-2.30181723085673));
#30951=CARTESIAN_POINT('Ctrl Pts',(-31.0701809909547,4.23063279613937,-0.319475851207252));
#30952=CARTESIAN_POINT('Ctrl Pts',(-30.9512719919596,3.86923364069296,1.74050225247754));
#30953=CARTESIAN_POINT('Ctrl Pts',(-30.8323629929648,2.56760636218215,3.37752821215737));
#30954=CARTESIAN_POINT('Ctrl Pts',(-30.7134539939697,0.642041383293453,
4.19382295160038));
#30955=CARTESIAN_POINT('Ctrl Pts',(-30.5945449949749,-1.43953109436157,
3.99098332553759));
#30956=CARTESIAN_POINT('Ctrl Pts',(-30.4756359959798,-3.17131430799793,
2.8183836925229));
#30957=CARTESIAN_POINT('Ctrl Pts',(-30.3567269969849,-4.13242405408636,
0.960800203588555));
#30958=CARTESIAN_POINT('Ctrl Pts',(-30.2378179979899,-4.08942441038536,
-1.1300353505695));
#30959=CARTESIAN_POINT('Ctrl Pts',(-30.118908998995,-3.05253333388674,-2.94673281729211));
#30960=CARTESIAN_POINT('Ctrl Pts',(-30.0396363329983,-1.86695937376294,
-3.67969605923881));
#30961=CARTESIAN_POINT('Ctrl Pts',(-30.,-1.22233170237264,-3.88263769354994));
#30962=CARTESIAN_POINT('Ctrl Pts',(-52.9038972033484,-1.91758108071817,
3.91047455474603));
#30963=CARTESIAN_POINT('Ctrl Pts',(-52.86426087035,-2.56683045838858,3.59210185960144));
#30964=CARTESIAN_POINT('Ctrl Pts',(-52.7849882043534,-3.70303779363018,
2.62604570071254));
#30965=CARTESIAN_POINT('Ctrl Pts',(-52.6660792053585,-4.50763096630964,
0.537519078889939));
#30966=CARTESIAN_POINT('Ctrl Pts',(-52.5471702063634,-4.21677326676694,
-1.68111160541844));
#30967=CARTESIAN_POINT('Ctrl Pts',(-52.4282612073685,-2.90127757180321,
-3.49147861575446));
#30968=CARTESIAN_POINT('Ctrl Pts',(-52.3093522083735,-0.880743547074977,
-4.45328586905181));
#30969=CARTESIAN_POINT('Ctrl Pts',(-52.1904432093786,1.35380126982937,-4.33299912800889));
#30970=CARTESIAN_POINT('Ctrl Pts',(-52.0715342103836,3.25937573751765,-3.15975478809644));
#30971=CARTESIAN_POINT('Ctrl Pts',(-51.9526252113886,4.37291331450708,-1.21870014511799));
#30972=CARTESIAN_POINT('Ctrl Pts',(-51.8337162123937,4.42382673209854,1.01850861399359));
#30973=CARTESIAN_POINT('Ctrl Pts',(-51.7148072133987,3.39974177779992,3.00821406204645));
#30974=CARTESIAN_POINT('Ctrl Pts',(-51.5958982144038,1.5495139746811,4.26692019190625));
#30975=CARTESIAN_POINT('Ctrl Pts',(-51.4769892154088,-0.677248621669522,
4.48875624801429));
#30976=CARTESIAN_POINT('Ctrl Pts',(-51.3580802164138,-2.73943852493104,
3.61981716370482));
#30977=CARTESIAN_POINT('Ctrl Pts',(-51.2391712174189,-4.13594011073033,
1.87125591564839));
#30978=CARTESIAN_POINT('Ctrl Pts',(-51.1202622184239,-4.52740097754102,
-0.332023675215382));
#30979=CARTESIAN_POINT('Ctrl Pts',(-51.001353219429,-3.81869548292833,-2.45462099347217));
#30980=CARTESIAN_POINT('Ctrl Pts',(-50.882444220434,-2.1820402870485,-3.98074107671791));
#30981=CARTESIAN_POINT('Ctrl Pts',(-50.7635352214391,-0.0151454797536541,
-4.53953411681569));
#30982=CARTESIAN_POINT('Ctrl Pts',(-50.6446262224441,2.1554297071115,-3.9952124020534));
#30983=CARTESIAN_POINT('Ctrl Pts',(-50.5257172234491,3.80223169652302,-2.48004707497751));
#30984=CARTESIAN_POINT('Ctrl Pts',(-50.4068082244542,4.52508471972987,-0.36222595983527));
#30985=CARTESIAN_POINT('Ctrl Pts',(-50.2878992254591,4.14833422457659,1.84361669744306));
#30986=CARTESIAN_POINT('Ctrl Pts',(-50.1689902264643,2.76353124200318,3.60145726636404));
#30987=CARTESIAN_POINT('Ctrl Pts',(-50.0500812274693,0.707185323833562,
4.48413740690186));
#30988=CARTESIAN_POINT('Ctrl Pts',(-49.9311722284743,-1.52100786751463,
4.27716429817339));
#30989=CARTESIAN_POINT('Ctrl Pts',(-49.8122632294794,-3.37959348114136,
3.03083276818174));
#30990=CARTESIAN_POINT('Ctrl Pts',(-49.6933542304844,-4.41693195530615,
1.04800356330028));
#30991=CARTESIAN_POINT('Ctrl Pts',(-49.5744452314894,-4.38094822261397,
-1.18949234435358));
#30992=CARTESIAN_POINT('Ctrl Pts',(-49.4555362324945,-3.28038639317473,
-3.13793952745429));
#30993=CARTESIAN_POINT('Ctrl Pts',(-49.3366272334995,-1.38268492053985,
-4.32386190540457));
#30994=CARTESIAN_POINT('Ctrl Pts',(-49.2177182345045,0.851011411269701,
-4.45907826174644));
#30995=CARTESIAN_POINT('Ctrl Pts',(-49.0988092355096,2.87791047854129,-3.51073078489306));
#30996=CARTESIAN_POINT('Ctrl Pts',(-48.9799002365147,4.20547225530699,-1.70926957392212));
#30997=CARTESIAN_POINT('Ctrl Pts',(-48.8609912375196,4.51109690294586,0.507547139411817));
#30998=CARTESIAN_POINT('Ctrl Pts',(-48.7420822385247,3.72051709640205,2.60102900827211));
#30999=CARTESIAN_POINT('Ctrl Pts',(-48.6231732395297,2.02584511434425,4.06245626920221));
#31000=CARTESIAN_POINT('Ctrl Pts',(-48.5042642405348,-0.161110781273072,
4.53669953629844));
#31001=CARTESIAN_POINT('Ctrl Pts',(-48.3853552415398,-2.3089164746562,3.9085168644326));
#31002=CARTESIAN_POINT('Ctrl Pts',(-48.2664462425448,-3.89565141777433,
2.33055774390717));
#31003=CARTESIAN_POINT('Ctrl Pts',(-48.1475372435499,-4.53573623832059,
0.186269006757307));
#31004=CARTESIAN_POINT('Ctrl Pts',(-48.0286282445549,-4.07362920300179,
-2.00328342551518));
#31005=CARTESIAN_POINT('Ctrl Pts',(-47.9097192455599,-2.62162313135259,
-3.70603447415832));
#31006=CARTESIAN_POINT('Ctrl Pts',(-47.7908102465651,-0.532558043768616,
-4.50821264987691));
#31007=CARTESIAN_POINT('Ctrl Pts',(-47.67190124757,1.68591958188536,-4.21488724996391));
#31008=CARTESIAN_POINT('Ctrl Pts',(-47.5529922485751,3.49471579416743,-2.89733686072048));
#31009=CARTESIAN_POINT('Ctrl Pts',(-47.4340832495801,4.45428994314883,-0.875728536052195));
#31010=CARTESIAN_POINT('Ctrl Pts',(-47.3151742505852,4.33146382874587,1.35868335779866));
#31011=CARTESIAN_POINT('Ctrl Pts',(-47.1962652515901,3.15608441204037,3.26293281428972));
#31012=CARTESIAN_POINT('Ctrl Pts',(-47.0773562525953,1.21377095142287,4.37428387784502));
#31013=CARTESIAN_POINT('Ctrl Pts',(-46.9584472536002,-1.02349097781175,
4.4226762921144));
#31014=CARTESIAN_POINT('Ctrl Pts',(-46.8395382546053,-3.01204280552752,
3.39635061561123));
#31015=CARTESIAN_POINT('Ctrl Pts',(-46.7206292556103,-4.26866295218099,
1.54470578660482));
#31016=CARTESIAN_POINT('Ctrl Pts',(-46.6017202566154,-4.48799051961058,
-0.682305256009673));
#31017=CARTESIAN_POINT('Ctrl Pts',(-46.4828112576204,-3.61672852450737,
-2.7435149255121));
#31018=CARTESIAN_POINT('Ctrl Pts',(-46.3639022586255,-1.86659515877466,
-4.13804565945467));
#31019=CARTESIAN_POINT('Ctrl Pts',(-46.2449932596305,0.33712410219086,-4.52702404524379));
#31020=CARTESIAN_POINT('Ctrl Pts',(-46.1260842606355,2.45892161543405,-3.81592765335548));
#31021=CARTESIAN_POINT('Ctrl Pts',(-46.0071752616406,3.98319686628377,-2.17755415338436));
#31022=CARTESIAN_POINT('Ctrl Pts',(-45.8882662626456,4.53954829712943,-0.0100311774599003));
#31023=CARTESIAN_POINT('Ctrl Pts',(-45.7693572636507,3.99278153513842,2.15992939216729));
#31024=CARTESIAN_POINT('Ctrl Pts',(-45.6504482646557,2.47576186181158,3.80502333371354));
#31025=CARTESIAN_POINT('Ctrl Pts',(-45.5315392656607,0.357127716706735,
4.52548993595379));
#31026=CARTESIAN_POINT('Ctrl Pts',(-45.4126302666659,-1.84828908951253,
4.14625455177934));
#31027=CARTESIAN_POINT('Ctrl Pts',(-45.2937212676707,-3.60456840740805,
2.75947204419623));
#31028=CARTESIAN_POINT('Ctrl Pts',(-45.1748122686759,-4.48493128445738,
0.702132993308606));
#31029=CARTESIAN_POINT('Ctrl Pts',(-45.0559032696808,-4.27544799844884,
-1.52582560573556));
#31030=CARTESIAN_POINT('Ctrl Pts',(-44.936994270686,-3.02702335513946,-3.38300590795949));
#31031=CARTESIAN_POINT('Ctrl Pts',(-44.8180852716909,-1.04302673083841,
-4.41810984553875));
#31032=CARTESIAN_POINT('Ctrl Pts',(-44.699176272696,1.1944272169753,-4.37960534585094));
#31033=CARTESIAN_POINT('Ctrl Pts',(-44.580267273701,3.14163325801131,-3.27684907285165));
#31034=CARTESIAN_POINT('Ctrl Pts',(-44.4613582747062,4.32541690996749,-1.37781272765106));
#31035=CARTESIAN_POINT('Ctrl Pts',(-44.342449275711,4.45811667333,0.856034517246394));
#31036=CARTESIAN_POINT('Ctrl Pts',(-44.2235402767162,3.50748626748243,2.88186389013902));
#31037=CARTESIAN_POINT('Ctrl Pts',(-44.1046312777212,1.70453055828503,4.20739525448328));
#31038=CARTESIAN_POINT('Ctrl Pts',(-43.9857222787262,-0.51262907883053,
4.51052226155237));
#31039=CARTESIAN_POINT('Ctrl Pts',(-43.8668132797313,-2.60521892204093,
3.71758432559523));
#31040=CARTESIAN_POINT('Ctrl Pts',(-43.7479042807363,-4.06473605926936,
2.02126713732172));
#31041=CARTESIAN_POINT('Ctrl Pts',(-43.6289952817413,-4.53651509331103,
-0.166222016241634));
#31042=CARTESIAN_POINT('Ctrl Pts',(-43.5100862827464,-3.90591324049294,
-2.3133179148294));
#31043=CARTESIAN_POINT('Ctrl Pts',(-43.3911772837514,-2.32616716114331,
-3.89827552754776));
#31044=CARTESIAN_POINT('Ctrl Pts',(-43.2722682847565,-0.181159308161473,
-4.53594132084483));
#31045=CARTESIAN_POINT('Ctrl Pts',(-43.1533592857615,2.00787241677026,-4.07137346893065));
#31046=CARTESIAN_POINT('Ctrl Pts',(-43.0344502867666,3.70898394970129,-2.61743867794264));
#31047=CARTESIAN_POINT('Ctrl Pts',(-42.9155412877716,4.50881321367573,-0.527493716791647));
#31048=CARTESIAN_POINT('Ctrl Pts',(-42.7966322887766,4.21297833889654,1.69069700726593));
#31049=CARTESIAN_POINT('Ctrl Pts',(-42.6777232897817,2.8934115172095,3.49791799870001));
#31050=CARTESIAN_POINT('Ctrl Pts',(-42.5588142907867,0.870682430564956,
4.45539291260512));
#31051=CARTESIAN_POINT('Ctrl Pts',(-42.4399052917917,-1.36350792716849,
4.32969261418979));
#31052=CARTESIAN_POINT('Ctrl Pts',(-42.3209962927968,-3.26659503355605,
3.15288061740756));
#31053=CARTESIAN_POINT('Ctrl Pts',(-42.2020872938018,-4.37543189718947,
1.20789606904693));
#31054=CARTESIAN_POINT('Ctrl Pts',(-42.0831782948068,-4.4219526374448,-1.02658672242564));
#31055=CARTESIAN_POINT('Ctrl Pts',(-41.9642692958119,-3.39209215496744,
-3.01961950747069));
#31056=CARTESIAN_POINT('Ctrl Pts',(-41.8453602968169,-1.54162650841238,
-4.26304394307656));
#31057=CARTESIAN_POINT('Ctrl Pts',(-41.6868149648237,1.43509142351444,-4.57885596676009));
#31058=CARTESIAN_POINT('Ctrl Pts',(-41.488633299832,4.69193163900032,-2.11978410921226));
#31059=CARTESIAN_POINT('Ctrl Pts',(-41.2508153018422,4.31990203265866,2.8010986421318));
#31060=CARTESIAN_POINT('Ctrl Pts',(-41.0526336368504,0.730371050858233,
4.7425697133777));
#31061=CARTESIAN_POINT('Ctrl Pts',(-40.8940883048573,-2.16503146415692,
3.98281241225996));
#31062=CARTESIAN_POINT('Ctrl Pts',(-40.7751793058622,-3.80752117851334,
2.47531283535268));
#31063=CARTESIAN_POINT('Ctrl Pts',(-40.6562703068674,-4.52603313669918,
0.35009923159964));
#31064=CARTESIAN_POINT('Ctrl Pts',(-40.5373613078723,-4.14409765101203,
-1.85199132272229));
#31065=CARTESIAN_POINT('Ctrl Pts',(-40.4184523088774,-2.75544541412728,
-3.60816017807445));
#31066=CARTESIAN_POINT('Ctrl Pts',(-40.2995433098824,-0.697061689712906,
-4.48547622907039));
#31067=CARTESIAN_POINT('Ctrl Pts',(-40.1806343108875,1.5306323426131,-4.27384821119483));
#31068=CARTESIAN_POINT('Ctrl Pts',(-40.0617253118924,3.38641858527642,-3.02314897066693));
#31069=CARTESIAN_POINT('Ctrl Pts',(-39.9428163128976,4.41927984955773,-1.03807921936737));
#31070=CARTESIAN_POINT('Ctrl Pts',(-39.8239073139026,4.37825805320775,1.19937593630724));
#31071=CARTESIAN_POINT('Ctrl Pts',(-39.7049983149076,3.27330701897601,3.14531529921155));
#31072=CARTESIAN_POINT('Ctrl Pts',(-39.5860893159126,1.37293907675853,4.32697028612962));
#31073=CARTESIAN_POINT('Ctrl Pts',(-39.4671803169177,-0.861056688138638,
4.4571474892461));
#31074=CARTESIAN_POINT('Ctrl Pts',(-39.3482713179227,-2.88581355669983,
3.50423827189687));
#31075=CARTESIAN_POINT('Ctrl Pts',(-39.2293623189278,-4.20931297966839,
1.69978888586903));
#31076=CARTESIAN_POINT('Ctrl Pts',(-39.1104533199328,-4.50994181697772,
-0.517710110001807));
#31077=CARTESIAN_POINT('Ctrl Pts',(-38.9915443209379,-3.71464696511105,
-2.60940567879596));
#31078=CARTESIAN_POINT('Ctrl Pts',(-38.8726353219429,-2.01668635127596,
-4.0670105741501));
#31079=CARTESIAN_POINT('Ctrl Pts',(-38.7537263229479,0.171332561266035,
-4.53632503221188));
#31080=CARTESIAN_POINT('Ctrl Pts',(-38.634817323953,2.31771737083191,-3.90330442580641));
#31081=CARTESIAN_POINT('Ctrl Pts',(-38.515908324958,3.90089279206749,-2.32177406796203));
#31082=CARTESIAN_POINT('Ctrl Pts',(-38.396999325963,4.53614443003203,-0.176048509308297));
#31083=CARTESIAN_POINT('Ctrl Pts',(-38.2780903269681,4.06910501960659,2.01245712921353));
#31084=CARTESIAN_POINT('Ctrl Pts',(-38.1591813279731,2.6132659579589,3.71193216628008));
#31085=CARTESIAN_POINT('Ctrl Pts',(-38.0402723289782,0.522398687851519,
4.50940117676266));
#31086=CARTESIAN_POINT('Ctrl Pts',(-37.9213633299832,-1.69541237887717,
4.21107779957103));
#31087=CARTESIAN_POINT('Ctrl Pts',(-37.8024543309883,-3.50123526600386,
2.88945513513179));
#31088=CARTESIAN_POINT('Ctrl Pts',(-37.6835453319932,-4.45625184670795,
0.865689808921497));
#31089=CARTESIAN_POINT('Ctrl Pts',(-37.5646363329983,-4.32839141804354,
-1.36843965844462));
#31090=CARTESIAN_POINT('Ctrl Pts',(-37.4457273340033,-3.14872428825265,
-3.27003589016275));
#31091=CARTESIAN_POINT('Ctrl Pts',(-37.3268183350084,-1.20391163753542,
-4.37700766912383));
#31092=CARTESIAN_POINT('Ctrl Pts',(-37.2079093360134,1.03345365124596,-4.42035891271123));
#31093=CARTESIAN_POINT('Ctrl Pts',(-37.0890003370185,3.0196878914008,-3.38955519279929));
#31094=CARTESIAN_POINT('Ctrl Pts',(-36.9700913380235,4.27213268122689,-1.53508362002973));
#31095=CARTESIAN_POINT('Ctrl Pts',(-36.8511823390285,4.48644174158915,0.692415963000866));
#31096=CARTESIAN_POINT('Ctrl Pts',(-36.7322733400336,3.61053759519256,2.7516572534012));
#31097=CARTESIAN_POINT('Ctrl Pts',(-36.6133643410387,1.85726648484098,4.14224100829228));
#31098=CARTESIAN_POINT('Ctrl Pts',(-36.4944553420436,-0.347323636626779,
4.52625293790943));
#31099=CARTESIAN_POINT('Ctrl Pts',(-36.3755463430487,-2.46751350562725,
3.81037747028294));
#31100=CARTESIAN_POINT('Ctrl Pts',(-36.2566373440537,-3.98809326785784,
2.1685735987879));
#31101=CARTESIAN_POINT('Ctrl Pts',(-36.1377283450588,-4.53955937592,-0.000197458152042056));
#31102=CARTESIAN_POINT('Ctrl Pts',(-36.0188193460638,-3.98790459897951,
-2.1689205324149));
#31103=CARTESIAN_POINT('Ctrl Pts',(-35.8999103470689,-2.46718201473872,
-3.81059211575349));
#31104=CARTESIAN_POINT('Ctrl Pts',(-35.7810013480739,-0.346929876594992,
-4.52628313599787));
#31105=CARTESIAN_POINT('Ctrl Pts',(-35.662092349079,1.85762682963819,-4.14207942081043));
#31106=CARTESIAN_POINT('Ctrl Pts',(-35.543183350084,3.61077696033784,-2.75134314638983));
#31107=CARTESIAN_POINT('Ctrl Pts',(-35.424274351089,4.4865019609327,-0.69202566501534));
#31108=CARTESIAN_POINT('Ctrl Pts',(-35.3053653520941,4.27199912136254,1.53545526589692));
#31109=CARTESIAN_POINT('Ctrl Pts',(-35.1864563530991,3.01939300760999,3.38981787594685));
#31110=CARTESIAN_POINT('Ctrl Pts',(-35.0675473541041,1.03306910080612,4.42044880068217));
#31111=CARTESIAN_POINT('Ctrl Pts',(-34.9486383551092,-1.20429240819219,
4.3769029189672));
#31112=CARTESIAN_POINT('Ctrl Pts',(-34.8297293561142,-3.14900875119183,
3.2697619563831));
#31113=CARTESIAN_POINT('Ctrl Pts',(-34.7108203571192,-4.32851044826741,
1.36806310736485));
#31114=CARTESIAN_POINT('Ctrl Pts',(-34.5919113581243,-4.45617651967321,
-0.866077474597983));
#31115=CARTESIAN_POINT('Ctrl Pts',(-34.4730023591293,-3.50098388629258,
-2.8897597122274));
#31116=CARTESIAN_POINT('Ctrl Pts',(-34.3540933601343,-1.69504603223854,
-4.21122527479655));
#31117=CARTESIAN_POINT('Ctrl Pts',(-34.2351843611394,0.52279097861952,-4.50935571441941));
#31118=CARTESIAN_POINT('Ctrl Pts',(-34.1162753621444,2.61358886535788,-3.71170481172332));
#31119=CARTESIAN_POINT('Ctrl Pts',(-33.9973663631495,4.06928007688015,-2.01210313413584));
#31120=CARTESIAN_POINT('Ctrl Pts',(-33.8784573641545,4.53612909734241,0.176443131734507));
#31121=CARTESIAN_POINT('Ctrl Pts',(-33.7595483651596,3.90069079650883,2.32211340733482));
#31122=CARTESIAN_POINT('Ctrl Pts',(-33.6406393661646,2.31737779523808,3.90350605489873));
#31123=CARTESIAN_POINT('Ctrl Pts',(-33.5217303671696,0.170937927970636,
4.53633988930195));
#31124=CARTESIAN_POINT('Ctrl Pts',(-33.4028213681746,-2.01704015540326,
4.06683517959457));
#31125=CARTESIAN_POINT('Ctrl Pts',(-33.2839123691797,-3.71487394567241,
2.60908239315094));
#31126=CARTESIAN_POINT('Ctrl Pts',(-33.1650033701847,-4.50998685594713,
0.517318012139963));
#31127=CARTESIAN_POINT('Ctrl Pts',(-33.0460943711898,-4.20916505540284,
-1.70015555255108));
#31128=CARTESIAN_POINT('Ctrl Pts',(-32.9271853721948,-2.88550876884117,
-3.50448833803139));
#31129=CARTESIAN_POINT('Ctrl Pts',(-32.8082763731999,-0.86066879390247,
-4.45722431495354));
#31130=CARTESIAN_POINT('Ctrl Pts',(-32.6893673742049,1.37331520645988,-4.32684697093947));
#31131=CARTESIAN_POINT('Ctrl Pts',(-32.57045837521,3.27358120463341,-3.14503822928193));
#31132=CARTESIAN_POINT('Ctrl Pts',(-32.451549376215,4.37836123227121,-1.19897968524445));
#31133=CARTESIAN_POINT('Ctrl Pts',(-32.33264037722,4.41919180651584,1.03843302332628));
#31134=CARTESIAN_POINT('Ctrl Pts',(-32.213731378225,3.3861510257669,3.02350468808081));
#31135=CARTESIAN_POINT('Ctrl Pts',(-32.0948223792301,1.53026961138005,4.27385941232357));
#31136=CARTESIAN_POINT('Ctrl Pts',(-31.9759133802351,-0.697470002040879,
4.48565881220849));
#31137=CARTESIAN_POINT('Ctrl Pts',(-31.8570043812402,-2.75572317987429,
3.60743525098863));
#31138=CARTESIAN_POINT('Ctrl Pts',(-31.7380953822452,-4.1443308001465,1.85259861596859));
#31139=CARTESIAN_POINT('Ctrl Pts',(-31.6191863832503,-4.52585876167512,
-0.352422759922571));
#31140=CARTESIAN_POINT('Ctrl Pts',(-31.5002773842552,-3.80759513219323,
-2.4718047274604));
#31141=CARTESIAN_POINT('Ctrl Pts',(-31.3813683852603,-2.16407917054937,
-3.99053393346338));
#31142=CARTESIAN_POINT('Ctrl Pts',(-31.2624593862654,0.00531174016416774,
-4.53955616057968));
#31143=CARTESIAN_POINT('Ctrl Pts',(-31.1435503872704,2.1734120531481,-3.98545876017553));
#31144=CARTESIAN_POINT('Ctrl Pts',(-31.0246413882754,3.81336909977593,-2.46288694577852));
#31145=CARTESIAN_POINT('Ctrl Pts',(-30.9057323892805,4.52667142565262,-0.341831181417046));
#31146=CARTESIAN_POINT('Ctrl Pts',(-30.7868233902855,4.1399833557953,1.86229393857194));
#31147=CARTESIAN_POINT('Ctrl Pts',(-30.6679143912906,2.747274677826,3.6138708283215));
#31148=CARTESIAN_POINT('Ctrl Pts',(-30.5490053922956,0.68696824420526,4.48728581137539));
#31149=CARTESIAN_POINT('Ctrl Pts',(-30.4300963933006,-1.54026231658092,
4.27025247770333));
#31150=CARTESIAN_POINT('Ctrl Pts',(-30.3111873943057,-3.39322710136354,
3.01560015776149));
#31151=CARTESIAN_POINT('Ctrl Pts',(-30.1922783953107,-4.42159052456228,
1.02803222045517));
#31152=CARTESIAN_POINT('Ctrl Pts',(-30.0733693963157,-4.37558197978096,
-1.20910960083043));
#31153=CARTESIAN_POINT('Ctrl Pts',(-29.9544603973208,-3.26613442579243,
-3.15293051555816));
#31154=CARTESIAN_POINT('Ctrl Pts',(-29.8751877313241,-1.99759989989656,
-3.93718287761652));
#31155=CARTESIAN_POINT('Ctrl Pts',(-29.8355513983258,-1.30786439202401,
-4.15432535756651));
#31156=CARTESIAN_POINT('Ctrl Pts',(-52.7394486016742,-2.0429884765144,4.16621468233141));
#31157=CARTESIAN_POINT('Ctrl Pts',(-52.6998122686759,-2.73469794856865,
3.82702081253498));
#31158=CARTESIAN_POINT('Ctrl Pts',(-52.6205396026792,-3.94521181740615,
2.79778579341567));
#31159=CARTESIAN_POINT('Ctrl Pts',(-52.5016306036842,-4.80242437368079,
0.572672151973649));
#31160=CARTESIAN_POINT('Ctrl Pts',(-52.3827216046893,-4.49254494566273,
-1.79105419433853));
#31161=CARTESIAN_POINT('Ctrl Pts',(-52.2638126056943,-3.09101748341397,
-3.71981693483926));
#31162=CARTESIAN_POINT('Ctrl Pts',(-52.1449036066994,-0.938343069574278,
-4.74452517527442));
#31163=CARTESIAN_POINT('Ctrl Pts',(-52.0259946077044,1.44233817363076,-4.61637183234714));
#31164=CARTESIAN_POINT('Ctrl Pts',(-51.9070856087094,3.47253481969342,-3.36639878522093));
#31165=CARTESIAN_POINT('Ctrl Pts',(-51.7881766097145,4.65889635654337,-1.29840160493764));
#31166=CARTESIAN_POINT('Ctrl Pts',(-51.6692676107195,4.71313944774054,1.08511779895128));
#31167=CARTESIAN_POINT('Ctrl Pts',(-51.5503586117246,3.62208062282748,3.20494748589602));
#31168=CARTESIAN_POINT('Ctrl Pts',(-51.4314496127296,1.65085024372788,4.54597141676343));
#31169=CARTESIAN_POINT('Ctrl Pts',(-51.3125406137347,-0.721539831467189,
4.78231527249984));
#31170=CARTESIAN_POINT('Ctrl Pts',(-51.1936316147397,-2.91859436601119,
3.85654866273941));
#31171=CARTESIAN_POINT('Ctrl Pts',(-51.0747226157447,-4.40642540268035,
1.99363370379486));
#31172=CARTESIAN_POINT('Ctrl Pts',(-50.9558136167498,-4.82348731883206,
-0.353737606829587));
#31173=CARTESIAN_POINT('Ctrl Pts',(-50.8369046177547,-4.06843337441483,
-2.61515012548823));
#31174=CARTESIAN_POINT('Ctrl Pts',(-50.7179956187599,-2.32474298299854,
-4.24107654664407));
#31175=CARTESIAN_POINT('Ctrl Pts',(-50.5990866197648,-0.0161359751194769,
-4.8364139501862));
#31176=CARTESIAN_POINT('Ctrl Pts',(-50.4801776207699,2.29639210453432,-4.25649427849261));
#31177=CARTESIAN_POINT('Ctrl Pts',(-50.3612686217749,4.05089287704335,-2.64223904081009));
#31178=CARTESIAN_POINT('Ctrl Pts',(-50.24235962278,4.82101958066735,-0.385915082954782));
#31179=CARTESIAN_POINT('Ctrl Pts',(-50.123450623785,4.4196300760155,1.96418691541067));
#31180=CARTESIAN_POINT('Ctrl Pts',(-50.00454162479,2.94426271653953,3.83698805115724));
#31181=CARTESIAN_POINT('Ctrl Pts',(-49.8856326257952,0.753434356377266,
4.77739436497606));
#31182=CARTESIAN_POINT('Ctrl Pts',(-49.7667236268001,-1.62047987293258,
4.5568854747224));
#31183=CARTESIAN_POINT('Ctrl Pts',(-49.6478146278053,-3.60061465285689,
3.22904542702235));
#31184=CARTESIAN_POINT('Ctrl Pts',(-49.5289056288102,-4.70579376119999,
1.11654168092161));
#31185=CARTESIAN_POINT('Ctrl Pts',(-49.4099966298152,-4.66745673755532,
-1.26728365066384));
#31186=CARTESIAN_POINT('Ctrl Pts',(-49.2910876308203,-3.49491954585864,
-3.34315683391453));
#31187=CARTESIAN_POINT('Ctrl Pts',(-49.1721786318254,-1.47311077884397,
-4.60663704685322));
#31188=CARTESIAN_POINT('Ctrl Pts',(-49.0532696328303,0.90666648940606,-4.75069638318088));
#31189=CARTESIAN_POINT('Ctrl Pts',(-48.9343606338354,3.06612221158225,-3.74032817167489));
#31190=CARTESIAN_POINT('Ctrl Pts',(-48.8154516348404,4.48050486223793,-1.82105365863946));
#31191=CARTESIAN_POINT('Ctrl Pts',(-48.6965426358454,4.8061169782227,0.540740085273374));
#31192=CARTESIAN_POINT('Ctrl Pts',(-48.5776336368505,3.9638342446399,2.7711330406897));
#31193=CARTESIAN_POINT('Ctrl Pts',(-48.4587246378556,2.15833284205031,4.32813581015072));
#31194=CARTESIAN_POINT('Ctrl Pts',(-48.3398156388606,-0.171647224147517,
4.83339399166099));
#31195=CARTESIAN_POINT('Ctrl Pts',(-48.2209066398656,-2.45991671402506,
4.16412896152871));
#31196=CARTESIAN_POINT('Ctrl Pts',(-48.1019976408707,-4.15042213080724,
2.4829732951217));
#31197=CARTESIAN_POINT('Ctrl Pts',(-47.9830886418757,-4.83236769520448,
0.198450766000718));
#31198=CARTESIAN_POINT('Ctrl Pts',(-47.8641796428808,-4.34003943979692,
-2.13429564709045));
#31199=CARTESIAN_POINT('Ctrl Pts',(-47.7452706438857,-2.79307399357064,
-3.9484044770795));
#31200=CARTESIAN_POINT('Ctrl Pts',(-47.6263616448909,-0.567386671382312,
-4.80304409862326));
#31201=CARTESIAN_POINT('Ctrl Pts',(-47.5074526458958,1.79617660643157,-4.49053558572806));
#31202=CARTESIAN_POINT('Ctrl Pts',(-47.3885436469009,3.72326582065724,-3.08681905477267));
#31203=CARTESIAN_POINT('Ctrl Pts',(-47.2696346479059,4.74559491455711,-0.933000083125277));
#31204=CARTESIAN_POINT('Ctrl Pts',(-47.150725648911,4.61473612643938,1.44753954402541));
#31205=CARTESIAN_POINT('Ctrl Pts',(-47.031816649916,3.36248837117773,3.47632452482166));
#31206=CARTESIAN_POINT('Ctrl Pts',(-46.9129076509211,1.29315004816182,4.66035655300334));
#31207=CARTESIAN_POINT('Ctrl Pts',(-46.7939986519261,-1.09042600310945,
4.71191377042543));
#31208=CARTESIAN_POINT('Ctrl Pts',(-46.6750896529311,-3.20902662439505,
3.61846768288813));
#31209=CARTESIAN_POINT('Ctrl Pts',(-46.5561806539363,-4.54782815137267,
1.64572760618649));
#31210=CARTESIAN_POINT('Ctrl Pts',(-46.4372716549411,-4.78149946641965,
-0.726927163346267));
#31211=CARTESIAN_POINT('Ctrl Pts',(-46.3183626559463,-3.8532580304152,-2.9229373580737));
#31212=CARTESIAN_POINT('Ctrl Pts',(-46.1994536569512,-1.98866813927163,
-4.40866865164845));
#31213=CARTESIAN_POINT('Ctrl Pts',(-46.0805446579564,0.359171595327386,
-4.82308573563571));
#31214=CARTESIAN_POINT('Ctrl Pts',(-45.9616356589613,2.61973200272841,-4.06548453226198));
#31215=CARTESIAN_POINT('Ctrl Pts',(-45.8427266599665,4.24369294176513,-2.31996346182361));
#31216=CARTESIAN_POINT('Ctrl Pts',(-45.7238176609714,4.83642905787465,-0.0106872038750072));
#31217=CARTESIAN_POINT('Ctrl Pts',(-45.6049086619765,4.25390443593254,2.3011860633449));
#31218=CARTESIAN_POINT('Ctrl Pts',(-45.4859996629815,2.63767358008176,4.05386708380217));
#31219=CARTESIAN_POINT('Ctrl Pts',(-45.3670906639866,0.380483421124782,
4.8214512975237));
#31220=CARTESIAN_POINT('Ctrl Pts',(-45.2481816649916,-1.96916487605686,
4.41741439522765));
#31221=CARTESIAN_POINT('Ctrl Pts',(-45.1292726659966,-3.84030265692052,
2.93993805229097));
#31222=CARTESIAN_POINT('Ctrl Pts',(-45.0103636670017,-4.77824016112727,
0.748051609777494));
#31223=CARTESIAN_POINT('Ctrl Pts',(-44.8914546680067,-4.5550569311501,-1.6256126851861));
#31224=CARTESIAN_POINT('Ctrl Pts',(-44.7725456690118,-3.22498688314855,
-3.60425024810576));
#31225=CARTESIAN_POINT('Ctrl Pts',(-44.6536366700168,-1.1112393698635,-4.70704868397537));
#31226=CARTESIAN_POINT('Ctrl Pts',(-44.5347276710218,1.27254125776094,-4.66602603833752));
#31227=CARTESIAN_POINT('Ctrl Pts',(-44.4158186720269,3.34709212981373,-3.49115088922637));
#31228=CARTESIAN_POINT('Ctrl Pts',(-44.2969096730319,4.60829374676278,-1.46791995065565));
#31229=CARTESIAN_POINT('Ctrl Pts',(-44.1780006740369,4.74967190808896,0.912018100208794));
#31230=CARTESIAN_POINT('Ctrl Pts',(-44.059091675042,3.736871466898,3.0703341713363));
#31231=CARTESIAN_POINT('Ctrl Pts',(-43.940182676047,1.81600471732796,4.48255362314666));
#31232=CARTESIAN_POINT('Ctrl Pts',(-43.8212736770521,-0.546154377151393,
4.80550475600336));
#31233=CARTESIAN_POINT('Ctrl Pts',(-43.7023646780571,-2.77559696955997,
3.96070967430342));
#31234=CARTESIAN_POINT('Ctrl Pts',(-43.5834556790621,-4.33056469562674,
2.15345547107664));
#31235=CARTESIAN_POINT('Ctrl Pts',(-43.4645466800672,-4.83319748633371,
-0.17709272746758));
#31236=CARTESIAN_POINT('Ctrl Pts',(-43.3456376810722,-4.16135506385137,
-2.46460600286104));
#31237=CARTESIAN_POINT('Ctrl Pts',(-43.2267286820773,-2.47829557375599,
-4.15321785406617));
#31238=CARTESIAN_POINT('Ctrl Pts',(-43.1078196830823,-0.193006899530237,
-4.83258618986839));
#31239=CARTESIAN_POINT('Ctrl Pts',(-42.9889106840873,2.13918475261367,-4.33763618354885));
#31240=CARTESIAN_POINT('Ctrl Pts',(-42.8700016850924,3.95154684462089,-2.78861588215986));
#31241=CARTESIAN_POINT('Ctrl Pts',(-42.7510926860974,4.80368393854071,-0.561991143777627));
#31242=CARTESIAN_POINT('Ctrl Pts',(-42.6321836871025,4.48850183427287,1.80126646943557));
#31243=CARTESIAN_POINT('Ctrl Pts',(-42.5132746881075,3.08263699872303,3.72667744534695));
#31244=CARTESIAN_POINT('Ctrl Pts',(-42.3943656891126,0.927623968672873,
4.74677001683145));
#31245=CARTESIAN_POINT('Ctrl Pts',(-42.2754566901175,-1.45267963417639,
4.6128490766745));
#31246=CARTESIAN_POINT('Ctrl Pts',(-42.1565476911226,-3.48022624863131,
3.35907505239722));
#31247=CARTESIAN_POINT('Ctrl Pts',(-42.0376386921276,-4.66157965137196,
1.28689095585245));
#31248=CARTESIAN_POINT('Ctrl Pts',(-41.9187296931327,-4.71114278964874,
-1.09372420553542));
#31249=CARTESIAN_POINT('Ctrl Pts',(-41.7998206941377,-3.61393072426332,
-3.21709883313528));
#31250=CARTESIAN_POINT('Ctrl Pts',(-41.6809116951427,-1.64244694706527,
-4.54184166612561));
#31251=CARTESIAN_POINT('Ctrl Pts',(-41.5223663631495,1.52894460133419,-4.87830739976151));
#31252=CARTESIAN_POINT('Ctrl Pts',(-41.3241846981579,4.99877807903749,-2.25841532927366));
#31253=CARTESIAN_POINT('Ctrl Pts',(-41.086366700168,4.60241820340005,2.9842869774832));
#31254=CARTESIAN_POINT('Ctrl Pts',(-40.8881850351763,0.778136400847418,
5.05272781991995));
#31255=CARTESIAN_POINT('Ctrl Pts',(-40.7296397031831,-2.30662180443871,
4.24328334493074));
#31256=CARTESIAN_POINT('Ctrl Pts',(-40.6107307041881,-4.05652828451666,
2.63719518785605));
#31257=CARTESIAN_POINT('Ctrl Pts',(-40.4918217051932,-4.82203002291603,
0.372995281913602));
#31258=CARTESIAN_POINT('Ctrl Pts',(-40.3729127061982,-4.41511643585742,
-1.97310923067162));
#31259=CARTESIAN_POINT('Ctrl Pts',(-40.2540037072032,-2.9356480856696,-3.84412932488023));
#31260=CARTESIAN_POINT('Ctrl Pts',(-40.1350947082083,-0.742648649291964,
-4.77882074443397));
#31261=CARTESIAN_POINT('Ctrl Pts',(-40.0161857092133,1.63073377662217,-4.55335251981767));
#31262=CARTESIAN_POINT('Ctrl Pts',(-39.8972767102183,3.60788611023574,-3.22085911879452));
#31263=CARTESIAN_POINT('Ctrl Pts',(-39.7783677112233,4.70829520478864,-1.1059682973522));
#31264=CARTESIAN_POINT('Ctrl Pts',(-39.6594587122285,4.66459063444655,1.27781361712572));
#31265=CARTESIAN_POINT('Ctrl Pts',(-39.5405497132334,3.48737718947312,3.35101497188689));
#31266=CARTESIAN_POINT('Ctrl Pts',(-39.4216407142385,1.462727569112,4.60994871177617));
#31267=CARTESIAN_POINT('Ctrl Pts',(-39.3027317152436,-0.917368714773737,
4.74863934058245));
#31268=CARTESIAN_POINT('Ctrl Pts',(-39.1838227162485,-3.07454214113269,
3.73341105647792));
#31269=CARTESIAN_POINT('Ctrl Pts',(-39.0649137172536,-4.48459676515183,
1.81095294548753));
#31270=CARTESIAN_POINT('Ctrl Pts',(-38.9460047182586,-4.80488635108207,
-0.551567701383731));
#31271=CARTESIAN_POINT('Ctrl Pts',(-38.8270957192637,-3.95758021413045,
-2.7800575349517));
#31272=CARTESIAN_POINT('Ctrl Pts',(-38.7081867202687,-2.14857510737313,
-4.33298796092579));
#31273=CARTESIAN_POINT('Ctrl Pts',(-38.5892777212738,0.18253749572199,-4.83299499547723));
#31274=CARTESIAN_POINT('Ctrl Pts',(-38.4703687222788,2.46929317776407,-4.15857563595885));
#31275=CARTESIAN_POINT('Ctrl Pts',(-38.3514597232838,4.15600628440037,-2.47361517779471));
#31276=CARTESIAN_POINT('Ctrl Pts',(-38.2325507242888,4.8328025821415,-0.187561860846965));
#31277=CARTESIAN_POINT('Ctrl Pts',(-38.1136417252939,4.33521938048628,2.14406929949615));
#31278=CARTESIAN_POINT('Ctrl Pts',(-37.9947327262989,2.78417027152664,3.95468787086344));
#31279=CARTESIAN_POINT('Ctrl Pts',(-37.875823727304,0.556562906339921,4.80431035367553));
#31280=CARTESIAN_POINT('Ctrl Pts',(-37.756914728309,-1.80629022043161,4.48647700206097));
#31281=CARTESIAN_POINT('Ctrl Pts',(-37.6380057293141,-3.73021165776875,
3.07842187422335));
#31282=CARTESIAN_POINT('Ctrl Pts',(-37.5190967303191,-4.74768512414649,
0.922304835840504));
#31283=CARTESIAN_POINT('Ctrl Pts',(-37.4001877313241,-4.6114627839335,-1.45793389448783));
#31284=CARTESIAN_POINT('Ctrl Pts',(-37.2812787323292,-3.35464690453247,
-3.48389213294125));
#31285=CARTESIAN_POINT('Ctrl Pts',(-37.1623697333342,-1.28264594752121,
-4.66325847681296));
#31286=CARTESIAN_POINT('Ctrl Pts',(-37.0434607343393,1.10104022288146,-4.70944483731798));
#31287=CARTESIAN_POINT('Ctrl Pts',(-36.9245517353443,3.21717168928859,-3.61122784795367));
#31288=CARTESIAN_POINT('Ctrl Pts',(-36.8056427363493,4.55152479634309,-1.63547616199481));
#31289=CARTESIAN_POINT('Ctrl Pts',(-36.6867337373544,4.77984940025959,0.737699097884072));
#31290=CARTESIAN_POINT('Ctrl Pts',(-36.5678247383594,3.84666222209386,2.93161218398677));
#31291=CARTESIAN_POINT('Ctrl Pts',(-36.4489157393645,1.9787293817717,4.41313837103418));
#31292=CARTESIAN_POINT('Ctrl Pts',(-36.3300067403695,-0.370038166513298,
4.82226419884955));
#31293=CARTESIAN_POINT('Ctrl Pts',(-36.2110977413745,-2.628885791756,4.05957137418291));
#31294=CARTESIAN_POINT('Ctrl Pts',(-36.0921887423796,-4.24890956185634,
2.31039559022863));
#31295=CARTESIAN_POINT('Ctrl Pts',(-35.9732797433846,-4.83644086120422,
-0.000210371667320702));
#31296=CARTESIAN_POINT('Ctrl Pts',(-35.8543707443896,-4.2487085542702,-2.31076521287933));
#31297=CARTESIAN_POINT('Ctrl Pts',(-35.7354617453947,-2.62853262177948,
-4.05980005719779));
#31298=CARTESIAN_POINT('Ctrl Pts',(-35.6165527463997,-0.369618655069714,
-4.82229637185506));
#31299=CARTESIAN_POINT('Ctrl Pts',(-35.4976437474047,1.97911329266632,-4.41296621593386));
#31300=CARTESIAN_POINT('Ctrl Pts',(-35.3787347484098,3.84691724141916,-2.93127753477115));
#31301=CARTESIAN_POINT('Ctrl Pts',(-35.2598257494148,4.77991355787262,-0.737283274900226));
#31302=CARTESIAN_POINT('Ctrl Pts',(-35.1409167504199,4.55138250183126,1.63587211303519));
#31303=CARTESIAN_POINT('Ctrl Pts',(-35.0220077514249,3.21685752046802,3.61150771024934));
#31304=CARTESIAN_POINT('Ctrl Pts',(-34.9030987524299,1.10063052332557,4.70954060384939));
#31305=CARTESIAN_POINT('Ctrl Pts',(-34.7841897534351,-1.28305162010095,
4.66314687612758));
#31306=CARTESIAN_POINT('Ctrl Pts',(-34.6652807544399,-3.35494997099078,
3.48360028423627));
#31307=CARTESIAN_POINT('Ctrl Pts',(-34.5463717554451,-4.6115895985846,1.45753271744012));
#31308=CARTESIAN_POINT('Ctrl Pts',(-34.4274627564501,-4.74760487081823,
-0.922717854365599));
#31309=CARTESIAN_POINT('Ctrl Pts',(-34.3085537574552,-3.7299438381399,-3.07874637027869));
#31310=CARTESIAN_POINT('Ctrl Pts',(-34.1896447584601,-1.80589991518268,
-4.48663412198111));
#31311=CARTESIAN_POINT('Ctrl Pts',(-34.0707357594653,0.556980852431709,
-4.80426191815211));
#31312=CARTESIAN_POINT('Ctrl Pts',(-33.9518267604702,2.78451429666418,-3.95444564760406));
#31313=CARTESIAN_POINT('Ctrl Pts',(-33.8329177614753,4.33540588628578,-2.14369215358474));
#31314=CARTESIAN_POINT('Ctrl Pts',(-33.7140087624803,4.83278624671323,0.187982291084487));
#31315=CARTESIAN_POINT('Ctrl Pts',(-33.5950997634854,4.15579107858574,2.47397670953652));
#31316=CARTESIAN_POINT('Ctrl Pts',(-33.4761907644904,2.46893139435267,4.1587904513407));
#31317=CARTESIAN_POINT('Ctrl Pts',(-33.3572817654955,0.18211705390445,4.83301082420234));
#31318=CARTESIAN_POINT('Ctrl Pts',(-33.2383727665005,-2.14895204984623,
4.3328010957865));
#31319=CARTESIAN_POINT('Ctrl Pts',(-33.1194637675056,-3.9578220389356,2.77971310683131));
#31320=CARTESIAN_POINT('Ctrl Pts',(-33.0005547685105,-4.80493433554354,
0.55114996081392));
#31321=CARTESIAN_POINT('Ctrl Pts',(-32.8816457695156,-4.48443916682499,
-1.81134359171032));
#31322=CARTESIAN_POINT('Ctrl Pts',(-32.7627367705206,-3.07421742053067,
-3.73367747662374));
#31323=CARTESIAN_POINT('Ctrl Pts',(-32.6438277715257,-0.916955452741436,
-4.74872119059472));
#31324=CARTESIAN_POINT('Ctrl Pts',(-32.5249187725307,1.46312829722367,-4.60981733192737));
#31325=CARTESIAN_POINT('Ctrl Pts',(-32.4060097735358,3.48766930652834,-3.35071978193168));
#31326=CARTESIAN_POINT('Ctrl Pts',(-32.2871007745408,4.66470056129123,-1.27739145174084));
#31327=CARTESIAN_POINT('Ctrl Pts',(-32.1681917755458,4.70820140384233,1.1063452396459));
#31328=CARTESIAN_POINT('Ctrl Pts',(-32.0492827765509,3.60760105267017,3.22123809968074));
#31329=CARTESIAN_POINT('Ctrl Pts',(-31.9303737775559,1.63034732322182,4.55336445348616));
#31330=CARTESIAN_POINT('Ctrl Pts',(-31.811464778561,-0.743083664733639,
4.77901526828014));
#31331=CARTESIAN_POINT('Ctrl Pts',(-31.692555779566,-2.93594401694779,3.84335698847294));
#31332=CARTESIAN_POINT('Ctrl Pts',(-31.573646780571,-4.41536483265262,1.97375624013402));
#31333=CARTESIAN_POINT('Ctrl Pts',(-31.4547377815761,-4.82184424398428,
-0.37547076607239));
#31334=CARTESIAN_POINT('Ctrl Pts',(-31.3358287825811,-4.05660707467442,
-2.63345765411083));
#31335=CARTESIAN_POINT('Ctrl Pts',(-31.2169197835861,-2.30560723202455,
-4.25150984392904));
#31336=CARTESIAN_POINT('Ctrl Pts',(-31.0980107845912,0.00565912130376327,
-4.83643743558468));
#31337=CARTESIAN_POINT('Ctrl Pts',(-30.9791017855962,2.31555047343088,-4.24610276067837));
#31338=CARTESIAN_POINT('Ctrl Pts',(-30.8601927866012,4.06275865248972,-2.6239566607003));
#31339=CARTESIAN_POINT('Ctrl Pts',(-30.7412837876063,4.82271005516587,-0.36418651162684));
#31340=CARTESIAN_POINT('Ctrl Pts',(-30.6223747886113,4.41073307089764,1.98408562466634));
#31341=CARTESIAN_POINT('Ctrl Pts',(-30.5034657896164,2.92694299346985,3.85021344448564));
#31342=CARTESIAN_POINT('Ctrl Pts',(-30.3845567906214,0.731895105117071,
4.78074867115039));
#31343=CARTESIAN_POINT('Ctrl Pts',(-30.2656477916264,-1.64099353880028,
4.54952162986908));
#31344=CARTESIAN_POINT('Ctrl Pts',(-30.1467387926315,-3.61513989472913,
3.21281662300008));
#31345=CARTESIAN_POINT('Ctrl Pts',(-30.0278297936365,-4.7107569950382,1.09526423732179));
#31346=CARTESIAN_POINT('Ctrl Pts',(-29.9089207946416,-4.66173954917656,
-1.28818385109136));
#31347=CARTESIAN_POINT('Ctrl Pts',(-29.7900117956466,-3.47973551769813,
-3.35912821382421));
#31348=CARTESIAN_POINT('Ctrl Pts',(-29.71073912965,-2.12824042603018,-4.19466969599423));
#31349=CARTESIAN_POINT('Ctrl Pts',(-29.6711027966516,-1.39339708167538,
-4.42601302158308));
#31350=CARTESIAN_POINT('Ctrl Pts',(-52.575,-2.16839587231062,4.42195480991679));
#31351=CARTESIAN_POINT('Ctrl Pts',(-52.5353636670017,-2.90256543874872,
4.06193976546852));
#31352=CARTESIAN_POINT('Ctrl Pts',(-52.4560910010051,-4.18738584118213,
2.9695258861188));
#31353=CARTESIAN_POINT('Ctrl Pts',(-52.3371820020101,-5.09721778105195,
0.607825225057359));
#31354=CARTESIAN_POINT('Ctrl Pts',(-52.2182730030151,-4.76831662455853,
-1.90099678325861));
#31355=CARTESIAN_POINT('Ctrl Pts',(-52.0993640040201,-3.28075739502472,
-3.94815525392406));
#31356=CARTESIAN_POINT('Ctrl Pts',(-51.9804550050252,-0.995942592073579,
-5.03576448149704));
#31357=CARTESIAN_POINT('Ctrl Pts',(-51.8615460060302,1.53087507743214,-4.8997445366854));
#31358=CARTESIAN_POINT('Ctrl Pts',(-51.7426370070352,3.68569390186919,-3.57304278234542));
#31359=CARTESIAN_POINT('Ctrl Pts',(-51.6237280080403,4.94487939857967,-1.3781030647573));
#31360=CARTESIAN_POINT('Ctrl Pts',(-51.5048190090453,5.00245216338252,1.15172698390898));
#31361=CARTESIAN_POINT('Ctrl Pts',(-51.3859100100504,3.84441946785506,3.40168090974558));
#31362=CARTESIAN_POINT('Ctrl Pts',(-51.2670010110554,1.75218651277466,4.8250226416206));
#31363=CARTESIAN_POINT('Ctrl Pts',(-51.1480920120605,-0.765831041264851,
5.07587429698539));
#31364=CARTESIAN_POINT('Ctrl Pts',(-51.0291830130655,-3.09775020709136,
4.093280161774));
#31365=CARTESIAN_POINT('Ctrl Pts',(-50.9102740140705,-4.67691069463037,
2.11601149194133));
#31366=CARTESIAN_POINT('Ctrl Pts',(-50.7913650150755,-5.11957366012311,
-0.375451538443796));
#31367=CARTESIAN_POINT('Ctrl Pts',(-50.6724560160806,-4.31817126590131,
-2.77567925750427));
#31368=CARTESIAN_POINT('Ctrl Pts',(-50.5535470170856,-2.46744567894858,
-4.50141201657024));
#31369=CARTESIAN_POINT('Ctrl Pts',(-50.4346380180907,-0.0171264704852943,
-5.1332937835567));
#31370=CARTESIAN_POINT('Ctrl Pts',(-50.3157290190957,2.43735450195713,-4.51777615493182));
#31371=CARTESIAN_POINT('Ctrl Pts',(-50.1968200201007,4.2995540575637,-2.80443100664268));
#31372=CARTESIAN_POINT('Ctrl Pts',(-50.0779110211058,5.11695444160483,-0.409604206074291));
#31373=CARTESIAN_POINT('Ctrl Pts',(-49.9590020221108,4.69092592745442,2.08475713337828));
#31374=CARTESIAN_POINT('Ctrl Pts',(-49.8400930231159,3.12499419107588,4.07251883595044));
#31375=CARTESIAN_POINT('Ctrl Pts',(-49.7211840241209,0.799683388920974,
5.07065132305026));
#31376=CARTESIAN_POINT('Ctrl Pts',(-49.6022750251259,-1.71995187835053,
4.8366066512714));
#31377=CARTESIAN_POINT('Ctrl Pts',(-49.483366026131,-3.82163582457242,3.42725808586297));
#31378=CARTESIAN_POINT('Ctrl Pts',(-49.3644570271361,-4.99465556709384,
1.18507979854295));
#31379=CARTESIAN_POINT('Ctrl Pts',(-49.245548028141,-4.95396525249667,-1.3450749569741));
#31380=CARTESIAN_POINT('Ctrl Pts',(-49.1266390291462,-3.70945269854255,
-3.54837414037477));
#31381=CARTESIAN_POINT('Ctrl Pts',(-49.0077300301511,-1.56353663714809,
-4.88941218830188));
#31382=CARTESIAN_POINT('Ctrl Pts',(-48.8888210311562,0.962321567542419,
-5.04231450461531));
#31383=CARTESIAN_POINT('Ctrl Pts',(-48.7699120321612,3.25433394462322,-3.96992555845671));
#31384=CARTESIAN_POINT('Ctrl Pts',(-48.6510030331663,4.75553746916888,-1.93283774335679));
#31385=CARTESIAN_POINT('Ctrl Pts',(-48.5320940341713,5.10113705349954,0.573933031134927));
#31386=CARTESIAN_POINT('Ctrl Pts',(-48.4131850351763,4.20715139287775,2.9412370731073));
#31387=CARTESIAN_POINT('Ctrl Pts',(-48.2942760361814,2.29082056975638,4.59381535109922));
#31388=CARTESIAN_POINT('Ctrl Pts',(-48.1753670371864,-0.182183667021966,
5.13008844702354));
#31389=CARTESIAN_POINT('Ctrl Pts',(-48.0564580381915,-2.61091695339391,
4.41974105862483));
#31390=CARTESIAN_POINT('Ctrl Pts',(-47.9375490391964,-4.40519284384016,
2.63538884633622));
#31391=CARTESIAN_POINT('Ctrl Pts',(-47.8186400402016,-5.12899915208836,
0.21063252524413));
#31392=CARTESIAN_POINT('Ctrl Pts',(-47.6997310412066,-4.60644967659206,
-2.26530786866572));
#31393=CARTESIAN_POINT('Ctrl Pts',(-47.5808220422116,-2.96452485578869,
-4.19077448000068));
#31394=CARTESIAN_POINT('Ctrl Pts',(-47.4619130432167,-0.602215298996013,
-5.09787554736961));
#31395=CARTESIAN_POINT('Ctrl Pts',(-47.3430040442217,1.90643363097778,-4.7661839214922));
#31396=CARTESIAN_POINT('Ctrl Pts',(-47.2240950452267,3.95181584714705,-3.27630124882485));
#31397=CARTESIAN_POINT('Ctrl Pts',(-47.1051860462317,5.03689988596539,-0.990271630198361));
#31398=CARTESIAN_POINT('Ctrl Pts',(-46.9862770472368,4.8980084241329,1.53639573025216));
#31399=CARTESIAN_POINT('Ctrl Pts',(-46.8673680482418,3.56889233031509,3.6897162353536));
#31400=CARTESIAN_POINT('Ctrl Pts',(-46.7484590492469,1.37252914490077,4.94642922816165));
#31401=CARTESIAN_POINT('Ctrl Pts',(-46.629550050252,-1.15736102840716,5.00115124873645));
#31402=CARTESIAN_POINT('Ctrl Pts',(-46.5106410512569,-3.40601044326257,
3.84058475016503));
#31403=CARTESIAN_POINT('Ctrl Pts',(-46.391732052262,-4.82699335056435,1.74674942576816));
#31404=CARTESIAN_POINT('Ctrl Pts',(-46.272823053267,-5.07500841322872,-0.771549070682864));
#31405=CARTESIAN_POINT('Ctrl Pts',(-46.1539140542721,-4.08978753632303,
-3.1023597906353));
#31406=CARTESIAN_POINT('Ctrl Pts',(-46.0350050552771,-2.11074111976858,
-4.67929164384222));
#31407=CARTESIAN_POINT('Ctrl Pts',(-45.9160960562821,0.381219088463907,
-5.11914742602763));
#31408=CARTESIAN_POINT('Ctrl Pts',(-45.7971870572872,2.78054239002277,-4.31504141116849));
#31409=CARTESIAN_POINT('Ctrl Pts',(-45.6782780582922,4.50418901724648,-2.46237277026286));
#31410=CARTESIAN_POINT('Ctrl Pts',(-45.5593690592973,5.13330981861987,-0.0113432302901153));
#31411=CARTESIAN_POINT('Ctrl Pts',(-45.4404600603022,4.51502733672665,2.44244273452252));
#31412=CARTESIAN_POINT('Ctrl Pts',(-45.3215510613074,2.79958529835195,4.30271083389079));
#31413=CARTESIAN_POINT('Ctrl Pts',(-45.2026420623123,0.403839125542828,
5.11741265909362));
#31414=CARTESIAN_POINT('Ctrl Pts',(-45.0837330633175,-2.09004066260118,
4.68857423867596));
#31415=CARTESIAN_POINT('Ctrl Pts',(-44.9648240643224,-4.076036906433,3.12040406038571));
#31416=CARTESIAN_POINT('Ctrl Pts',(-44.8459150653275,-5.07154903779715,
0.793970226246384));
#31417=CARTESIAN_POINT('Ctrl Pts',(-44.7270060663325,-4.83466586385136,
-1.72539976463664));
#31418=CARTESIAN_POINT('Ctrl Pts',(-44.6080970673376,-3.42295041115765,
-3.82549458825203));
#31419=CARTESIAN_POINT('Ctrl Pts',(-44.4891880683426,-1.17945200888858,
-4.99598752241199));
#31420=CARTESIAN_POINT('Ctrl Pts',(-44.3702790693476,1.35065529854657,-4.9524467308241));
#31421=CARTESIAN_POINT('Ctrl Pts',(-44.2513700703527,3.55255100161615,-3.70545270560108));
#31422=CARTESIAN_POINT('Ctrl Pts',(-44.1324610713577,4.89117058355806,-1.55802717366026));
#31423=CARTESIAN_POINT('Ctrl Pts',(-44.0135520723628,5.04122714284792,0.968001683171198));
#31424=CARTESIAN_POINT('Ctrl Pts',(-43.8946430733678,3.96625666631358,3.25880445253356));
#31425=CARTESIAN_POINT('Ctrl Pts',(-43.7757340743728,1.92747887637088,4.75771199181005));
#31426=CARTESIAN_POINT('Ctrl Pts',(-43.6568250753779,-0.579679675472256,
5.10048725045433));
#31427=CARTESIAN_POINT('Ctrl Pts',(-43.5379160763829,-2.94597501707901,
4.20383502301162));
#31428=CARTESIAN_POINT('Ctrl Pts',(-43.419007077388,-4.59639333198412,2.28564380483155));
#31429=CARTESIAN_POINT('Ctrl Pts',(-43.300098078393,-5.12987987935639,-0.187963438693522));
#31430=CARTESIAN_POINT('Ctrl Pts',(-43.181189079398,-4.41679688720981,-2.61589409089269));
#31431=CARTESIAN_POINT('Ctrl Pts',(-43.0622800804031,-2.63042398636866,
-4.40816018058456));
#31432=CARTESIAN_POINT('Ctrl Pts',(-42.9433710814082,-0.204854490899003,
-5.12923105889195));
#31433=CARTESIAN_POINT('Ctrl Pts',(-42.8244620824131,2.27049708845707,-4.60389889816705));
#31434=CARTESIAN_POINT('Ctrl Pts',(-42.7055530834182,4.1941097395405,-2.95979308637708));
#31435=CARTESIAN_POINT('Ctrl Pts',(-42.5866440844232,5.09855466340569,-0.596488570763601));
#31436=CARTESIAN_POINT('Ctrl Pts',(-42.4677350854283,4.76402532964921,1.9118359316052));
#31437=CARTESIAN_POINT('Ctrl Pts',(-42.3488260864333,3.27186248023655,3.95543689199389));
#31438=CARTESIAN_POINT('Ctrl Pts',(-42.2299170874383,0.984565506780792,
5.03814712105775));
#31439=CARTESIAN_POINT('Ctrl Pts',(-42.1110080884434,-1.54185134118429,
4.89600553915921));
#31440=CARTESIAN_POINT('Ctrl Pts',(-41.9920990894484,-3.69385746370658,
3.56526948738689));
#31441=CARTESIAN_POINT('Ctrl Pts',(-41.8731900904534,-4.94772740555443,
1.36588584265797));
#31442=CARTESIAN_POINT('Ctrl Pts',(-41.7542810914585,-5.00033294185268,
-1.16086168864519));
#31443=CARTESIAN_POINT('Ctrl Pts',(-41.6353720924635,-3.83576929355919,
-3.41457815879987));
#31444=CARTESIAN_POINT('Ctrl Pts',(-41.5164630934686,-1.74326738571816,
-4.82063938917464));
#31445=CARTESIAN_POINT('Ctrl Pts',(-41.3579177614753,1.62279777915393,-5.17775883276294));
#31446=CARTESIAN_POINT('Ctrl Pts',(-41.1597360964837,5.30562451907466,-2.39704654933505));
#31447=CARTESIAN_POINT('Ctrl Pts',(-40.9219180984938,4.88493437414144,3.16747531283459));
#31448=CARTESIAN_POINT('Ctrl Pts',(-40.7237364335022,0.825901750836606,
5.36288592646222));
#31449=CARTESIAN_POINT('Ctrl Pts',(-40.5651911015089,-2.4482121447205,4.5037542776015));
#31450=CARTESIAN_POINT('Ctrl Pts',(-40.4462821025139,-4.30553539051999,
2.79907754035943));
#31451=CARTESIAN_POINT('Ctrl Pts',(-40.327373103519,-5.11802690913289,0.395891332227557));
#31452=CARTESIAN_POINT('Ctrl Pts',(-40.208464104524,-4.68613522070281,-2.09422713862094));
#31453=CARTESIAN_POINT('Ctrl Pts',(-40.0895551055291,-3.11585075721193,
-4.08009847168603));
#31454=CARTESIAN_POINT('Ctrl Pts',(-39.970646106534,-0.788235608871022,
-5.07216525979755));
#31455=CARTESIAN_POINT('Ctrl Pts',(-39.8517371075391,1.73083521063125,-4.83285682844052));
#31456=CARTESIAN_POINT('Ctrl Pts',(-39.7328281085442,3.82935363519506,-3.41856926692211));
#31457=CARTESIAN_POINT('Ctrl Pts',(-39.6139191095492,4.99731056001954,-1.17385737533702));
#31458=CARTESIAN_POINT('Ctrl Pts',(-39.4950101105542,4.95092321568535,1.3562512979442));
#31459=CARTESIAN_POINT('Ctrl Pts',(-39.3761011115593,3.70144735997023,3.55671464456224));
#31460=CARTESIAN_POINT('Ctrl Pts',(-39.2571921125643,1.55251606146547,4.8929271374227));
#31461=CARTESIAN_POINT('Ctrl Pts',(-39.1382831135694,-0.973680741408834,
5.04013119191881));
#31462=CARTESIAN_POINT('Ctrl Pts',(-39.0193741145743,-3.26327072556555,
3.96258384105897));
#31463=CARTESIAN_POINT('Ctrl Pts',(-38.9004651155794,-4.75988055063526,
1.92211700510603));
#31464=CARTESIAN_POINT('Ctrl Pts',(-38.7815561165845,-5.09983088518642,
-0.585425292765658));
#31465=CARTESIAN_POINT('Ctrl Pts',(-38.6626471175895,-4.20051346314986,
-2.95070939110744));
#31466=CARTESIAN_POINT('Ctrl Pts',(-38.5437381185946,-2.2804638634703,-4.59896534770147));
#31467=CARTESIAN_POINT('Ctrl Pts',(-38.4248291195996,0.193742430177945,
-5.12966495874259));
#31468=CARTESIAN_POINT('Ctrl Pts',(-38.3059201206046,2.62086898469623,-4.41384684611128));
#31469=CARTESIAN_POINT('Ctrl Pts',(-38.1870111216097,4.41111977673326,-2.6254562876274));
#31470=CARTESIAN_POINT('Ctrl Pts',(-38.0681021226147,5.12946073425098,-0.199075212385634));
#31471=CARTESIAN_POINT('Ctrl Pts',(-37.9491931236197,4.60133374136596,2.27568146977877));
#31472=CARTESIAN_POINT('Ctrl Pts',(-37.8302841246248,2.95507458509439,4.19744357544679));
#31473=CARTESIAN_POINT('Ctrl Pts',(-37.7113751256298,0.590727124828317,
5.09921953058841));
#31474=CARTESIAN_POINT('Ctrl Pts',(-37.5924661266348,-1.91716806198604,
4.76187620455091));
#31475=CARTESIAN_POINT('Ctrl Pts',(-37.4735571276399,-3.95918804953365,
3.26738861331491));
#31476=CARTESIAN_POINT('Ctrl Pts',(-37.3546481286449,-5.03911840158502,
0.978919862759506));
#31477=CARTESIAN_POINT('Ctrl Pts',(-37.23573912965,-4.89453414982347,-1.54742813053104));
#31478=CARTESIAN_POINT('Ctrl Pts',(-37.116830130655,-3.56056952081229,-3.69774837571975));
#31479=CARTESIAN_POINT('Ctrl Pts',(-36.99792113166,-1.36138025750699,-4.94950928450209));
#31480=CARTESIAN_POINT('Ctrl Pts',(-36.8790121326651,1.16862679451695,-4.99853076192473));
#31481=CARTESIAN_POINT('Ctrl Pts',(-36.7601031336701,3.41465548717637,-3.83290050310805));
#31482=CARTESIAN_POINT('Ctrl Pts',(-36.6411941346751,4.83091691145929,-1.73586870395989));
#31483=CARTESIAN_POINT('Ctrl Pts',(-36.5222851356802,5.07325705893003,0.782982232767275));
#31484=CARTESIAN_POINT('Ctrl Pts',(-36.4033761366852,4.08278684899514,3.11156711457234));
#31485=CARTESIAN_POINT('Ctrl Pts',(-36.2844671376903,2.10019227870243,4.68403573377608));
#31486=CARTESIAN_POINT('Ctrl Pts',(-36.1655581386953,-0.392752696399822,
5.11827545978968));
#31487=CARTESIAN_POINT('Ctrl Pts',(-36.0466491397004,-2.79025807788474,
4.30876527808287));
#31488=CARTESIAN_POINT('Ctrl Pts',(-35.9277401407054,-4.50972585585484,
2.45221758166935));
#31489=CARTESIAN_POINT('Ctrl Pts',(-35.8088311417104,-5.13332234648844,
-0.000223285182599037));
#31490=CARTESIAN_POINT('Ctrl Pts',(-35.6899221427155,-4.50951250956089,
-2.45260989334375));
#31491=CARTESIAN_POINT('Ctrl Pts',(-35.5710131437205,-2.78988322882023,
-4.30900799864209));
#31492=CARTESIAN_POINT('Ctrl Pts',(-35.4521041447255,-0.392307433544437,
-5.11830960771226));
#31493=CARTESIAN_POINT('Ctrl Pts',(-35.3331951457306,2.10059975569445,-4.68385301105728));
#31494=CARTESIAN_POINT('Ctrl Pts',(-35.2142861467356,4.08305752250047,-3.11121192315247));
#31495=CARTESIAN_POINT('Ctrl Pts',(-35.0953771477407,5.07332515481253,-0.782540884785113));
#31496=CARTESIAN_POINT('Ctrl Pts',(-34.9764681487457,4.83076588229999,1.73628896017346));
#31497=CARTESIAN_POINT('Ctrl Pts',(-34.8575591497507,3.41432203332604,3.83319754455183));
#31498=CARTESIAN_POINT('Ctrl Pts',(-34.7386501507558,1.16819194584502,4.99863240701661));
#31499=CARTESIAN_POINT('Ctrl Pts',(-34.6197411517608,-1.36181083200972,
4.94939083328796));
#31500=CARTESIAN_POINT('Ctrl Pts',(-34.5008321527658,-3.56089119078974,
3.69743861208944));
#31501=CARTESIAN_POINT('Ctrl Pts',(-34.3819231537709,-4.89466874890179,
1.5470023275154));
#31502=CARTESIAN_POINT('Ctrl Pts',(-34.2630141547759,-5.03903322196325,
-0.979358234133216));
#31503=CARTESIAN_POINT('Ctrl Pts',(-34.144105155781,-3.95890378998724,-3.26773302832997));
#31504=CARTESIAN_POINT('Ctrl Pts',(-34.025196156786,-1.91675379812682,-4.76204296916568));
#31505=CARTESIAN_POINT('Ctrl Pts',(-33.906287157791,0.591170726243899,-5.0991681218848));
#31506=CARTESIAN_POINT('Ctrl Pts',(-33.7873781587961,2.95543972797048,-4.19718648348481));
#31507=CARTESIAN_POINT('Ctrl Pts',(-33.6684691598011,4.60153169569141,-2.27528117303364));
#31508=CARTESIAN_POINT('Ctrl Pts',(-33.5495601608061,5.12944339608405,0.199521450434463));
#31509=CARTESIAN_POINT('Ctrl Pts',(-33.4306511618112,4.41089136066265,2.62584001173821));
#31510=CARTESIAN_POINT('Ctrl Pts',(-33.3117421628162,2.62048499346726,4.41407484778267));
#31511=CARTESIAN_POINT('Ctrl Pts',(-33.1928331638213,0.193296179838262,
5.12968175910273));
#31512=CARTESIAN_POINT('Ctrl Pts',(-33.0739241648263,-2.28086394428919,
4.59876701197841));
#31513=CARTESIAN_POINT('Ctrl Pts',(-32.9550151658314,-4.2007701321988,2.95034382051169));
#31514=CARTESIAN_POINT('Ctrl Pts',(-32.8361061668364,-5.09988181513996,
0.584981909487872));
#31515=CARTESIAN_POINT('Ctrl Pts',(-32.7171971678414,-4.75971327824715,
-1.92253163086956));
#31516=CARTESIAN_POINT('Ctrl Pts',(-32.5982881688464,-3.26292607222017,
-3.96286661521608));
#31517=CARTESIAN_POINT('Ctrl Pts',(-32.4793791698515,-0.973242111580406,
-5.04021806623591));
#31518=CARTESIAN_POINT('Ctrl Pts',(-32.3604701708565,1.55294138798746,-4.89278769291527));
#31519=CARTESIAN_POINT('Ctrl Pts',(-32.2415611718616,3.70175740842325,-3.55640133458143));
#31520=CARTESIAN_POINT('Ctrl Pts',(-32.1226521728666,4.95103989031126,-1.35580321823721));
#31521=CARTESIAN_POINT('Ctrl Pts',(-32.0037431738717,4.99721100116881,1.1742574559655));
#31522=CARTESIAN_POINT('Ctrl Pts',(-31.8848341748767,3.82905107957342,3.41897151128069));
#31523=CARTESIAN_POINT('Ctrl Pts',(-31.7659251758817,1.73042503506359,4.83286949464875));
#31524=CARTESIAN_POINT('Ctrl Pts',(-31.6470161768868,-0.788697327426404,
5.0723717243518));
#31525=CARTESIAN_POINT('Ctrl Pts',(-31.5281071778918,-3.11616485402129,
4.07927872595725));
#31526=CARTESIAN_POINT('Ctrl Pts',(-31.4091981788969,-4.68639886515875,
2.09491386429945));
#31527=CARTESIAN_POINT('Ctrl Pts',(-31.2902891799019,-5.11782972629342,
-0.398518772222211));
#31528=CARTESIAN_POINT('Ctrl Pts',(-31.1713801809069,-4.30561901715562,
-2.79511058076127));
#31529=CARTESIAN_POINT('Ctrl Pts',(-31.052471181912,-2.44713529349973,-4.5124857543947));
#31530=CARTESIAN_POINT('Ctrl Pts',(-30.933562182917,0.00600650244336238,
-5.13331871058968));
#31531=CARTESIAN_POINT('Ctrl Pts',(-30.8146531839221,2.45768889371366,-4.50674676118122));
#31532=CARTESIAN_POINT('Ctrl Pts',(-30.6957441849271,4.31214820520351,-2.78502637562208));
#31533=CARTESIAN_POINT('Ctrl Pts',(-30.5768351859322,5.11874868467912,-0.386541841836633));
#31534=CARTESIAN_POINT('Ctrl Pts',(-30.4579261869371,4.68148278599999,2.10587731076074));
#31535=CARTESIAN_POINT('Ctrl Pts',(-30.3390171879422,3.1066113091137,4.08655606064977));
#31536=CARTESIAN_POINT('Ctrl Pts',(-30.2201081889472,0.776821966028881,
5.0742115309254));
#31537=CARTESIAN_POINT('Ctrl Pts',(-30.1011991899523,-1.74172476101964,
4.82879078203482));
#31538=CARTESIAN_POINT('Ctrl Pts',(-29.9822901909573,-3.83705268809473,
3.41003308823867));
#31539=CARTESIAN_POINT('Ctrl Pts',(-29.8633811919624,-4.99992346551413,
1.16249625418841));
#31540=CARTESIAN_POINT('Ctrl Pts',(-29.7444721929674,-4.94789711857216,
-1.3672581013523));
#31541=CARTESIAN_POINT('Ctrl Pts',(-29.6255631939724,-3.69333660960383,
-3.56532591209026));
#31542=CARTESIAN_POINT('Ctrl Pts',(-29.5462905279758,-2.2588809521638,-4.45215651437195));
#31543=CARTESIAN_POINT('Ctrl Pts',(-29.5066541949775,-1.47892977132675,
-4.69770068559965));
#31544=CARTESIAN_POINT('',(-30.,-3.42872620889076,3.53545776165769));
#31545=CARTESIAN_POINT('Ctrl Pts',(-30.,-3.42895048616045,3.53554286219762));
#31546=CARTESIAN_POINT('Ctrl Pts',(-30.,-3.50915824907527,3.44370185733568));
#31547=CARTESIAN_POINT('Ctrl Pts',(-30.,-3.5858151589605,3.34898224904683));
#31548=CARTESIAN_POINT('Ctrl Pts',(-30.,-3.65871285115596,3.25152489539123));
#31549=CARTESIAN_POINT('Ctrl Pts',(-30.,-3.74535380187751,3.1356940985412));
#31550=CARTESIAN_POINT('Ctrl Pts',(-30.,-3.8266858316306,3.01599591628009));
#31551=CARTESIAN_POINT('Ctrl Pts',(-30.,-3.90252528247381,2.89283180563127));
#31552=CARTESIAN_POINT('Ctrl Pts',(-30.,-3.94702891750592,2.82055740796055));
#31553=CARTESIAN_POINT('Ctrl Pts',(-30.,-3.98964027665325,2.74708912193236));
#31554=CARTESIAN_POINT('Ctrl Pts',(-30.,-4.03031418131548,2.67250586558729));
#31555=CARTESIAN_POINT('Ctrl Pts',(-30.,-4.05883144322561,2.62021410080679));
#31556=CARTESIAN_POINT('Ctrl Pts',(-30.,-4.08639618876187,2.56737422065883));
#31557=CARTESIAN_POINT('Ctrl Pts',(-30.,-4.11299101272886,2.51401321575239));
#31558=CARTESIAN_POINT('Ctrl Pts',(-30.,-4.1267818975772,2.48634258800281));
#31559=CARTESIAN_POINT('Ctrl Pts',(-30.,-4.1403138718257,2.45852754287451));
#31560=CARTESIAN_POINT('Ctrl Pts',(-30.,-4.15357199197421,2.43059854489151));
#31561=CARTESIAN_POINT('Ctrl Pts',(-30.,-4.21456648083399,2.30211012140037));
#31562=CARTESIAN_POINT('Ctrl Pts',(-30.,-4.26981903788002,2.17111455395773));
#31563=CARTESIAN_POINT('Ctrl Pts',(-30.,-4.31915507771131,2.03799840069774));
#31564=CARTESIAN_POINT('Ctrl Pts',(-30.,-4.36809646707205,1.90594707454391));
#31565=CARTESIAN_POINT('Ctrl Pts',(-30.,-4.41121576257342,1.77180819965443));
#31566=CARTESIAN_POINT('Ctrl Pts',(-30.,-4.44829211824752,1.63595208979158));
#31567=CARTESIAN_POINT('Ctrl Pts',(-30.,-4.4740200136751,1.54167929182643));
#31568=CARTESIAN_POINT('Ctrl Pts',(-30.,-4.49683706950385,1.44657946040838));
#31569=CARTESIAN_POINT('Ctrl Pts',(-30.,-4.51665445828582,1.35077716111864));
#31570=CARTESIAN_POINT('Ctrl Pts',(-30.,-4.52076402557002,1.33091046731537));
#31571=CARTESIAN_POINT('Ctrl Pts',(-30.,-4.52474455448724,1.31101357182006));
#31572=CARTESIAN_POINT('Ctrl Pts',(-30.,-4.5285951840834,1.29108759749586));
#31573=CARTESIAN_POINT('Ctrl Pts',(-30.,-4.53235404910015,1.2716364802327));
#31574=CARTESIAN_POINT('Ctrl Pts',(-30.,-4.53598714329179,1.25216794356776));
#31575=CARTESIAN_POINT('Ctrl Pts',(-30.,-4.53949403413647,1.23268315058861));
#31576=CARTESIAN_POINT('Ctrl Pts',(-30.,-4.54971861620548,1.17587389311906));
#31577=CARTESIAN_POINT('Ctrl Pts',(-30.,-4.55887057855727,1.11892613790267));
#31578=CARTESIAN_POINT('Ctrl Pts',(-30.,-4.56693872096676,1.06186566568387));
#31579=CARTESIAN_POINT('Ctrl Pts',(-30.,-4.58634448579418,0.924621917542047));
#31580=CARTESIAN_POINT('Ctrl Pts',(-30.,-4.59948384692545,0.78672603593175));
#31581=CARTESIAN_POINT('Ctrl Pts',(-30.,-4.60642482463028,0.648594114271953));
#31582=CARTESIAN_POINT('Ctrl Pts',(-30.,-4.61338602653636,0.510059712169018));
#31583=CARTESIAN_POINT('Ctrl Pts',(-30.,-4.61411251727511,0.371287074813086));
#31584=CARTESIAN_POINT('Ctrl Pts',(-30.,-4.60862117424193,0.232702680772997));
#31585=CARTESIAN_POINT('Ctrl Pts',(-30.,-4.60321431390715,0.0962503668985886));
#31586=CARTESIAN_POINT('Ctrl Pts',(-30.,-4.59177918602515,-0.0400201649351817));
#31587=CARTESIAN_POINT('Ctrl Pts',(-30.,-4.57428528182906,-0.175683987839321));
#31588=CARTESIAN_POINT('Ctrl Pts',(-30.,-4.56307291200204,-0.262635015894491));
#31589=CARTESIAN_POINT('Ctrl Pts',(-30.,-4.54937072347399,-0.349336422774511));
#31590=CARTESIAN_POINT('Ctrl Pts',(-30.,-4.53316113535111,-0.435670359101438));
#31591=CARTESIAN_POINT('Ctrl Pts',(-30.,-4.52960775784034,-0.454596013808723));
#31592=CARTESIAN_POINT('Ctrl Pts',(-30.,-4.52593385944817,-0.473503988545268));
#31593=CARTESIAN_POINT('Ctrl Pts',(-30.,-4.52213920851564,-0.492393004726145));
#31594=CARTESIAN_POINT('Ctrl Pts',(-30.,-4.51862269595122,-0.509897503535277));
#31595=CARTESIAN_POINT('Ctrl Pts',(-30.,-4.51500446283229,-0.527375860827068));
#31596=CARTESIAN_POINT('Ctrl Pts',(-30.,-4.51128474310241,-0.544826751555983));
#31597=CARTESIAN_POINT('Ctrl Pts',(-30.,-4.48314120023153,-0.676860863540087));
#31598=CARTESIAN_POINT('Ctrl Pts',(-30.,-4.44919041908381,-0.807332295944959));
#31599=CARTESIAN_POINT('Ctrl Pts',(-30.,-4.40946707177224,-0.935850920961004));
#31600=CARTESIAN_POINT('Ctrl Pts',(-30.,-4.38257271922611,-1.02286335681679));
#31601=CARTESIAN_POINT('Ctrl Pts',(-30.,-4.35303126425028,-1.10898042810463));
#31602=CARTESIAN_POINT('Ctrl Pts',(-30.,-4.32084099235389,-1.19407565851423));
#31603=CARTESIAN_POINT('Ctrl Pts',(-30.,-4.27308790247552,-1.32031131750617));
#31604=CARTESIAN_POINT('Ctrl Pts',(-30.,-4.21950722125047,-1.44429998404022));
#31605=CARTESIAN_POINT('Ctrl Pts',(-30.,-4.16031888721692,-1.56567294676739));
#31606=CARTESIAN_POINT('Ctrl Pts',(-30.,-4.10160826700295,-1.68606629851947));
#31607=CARTESIAN_POINT('Ctrl Pts',(-30.,-4.03737956959752,-1.80388657460641));
#31608=CARTESIAN_POINT('Ctrl Pts',(-30.,-3.96781310771827,-1.91873618474768));
#31609=CARTESIAN_POINT('Ctrl Pts',(-30.,-3.94906147189672,-1.94969389059385));
#31610=CARTESIAN_POINT('Ctrl Pts',(-30.,-3.92992184197122,-1.98043551594257));
#31611=CARTESIAN_POINT('Ctrl Pts',(-30.,-3.91039740038924,-2.01095271663753));
#31612=CARTESIAN_POINT('Ctrl Pts',(-30.,-3.89784637190895,-2.03057029460784));
#31613=CARTESIAN_POINT('Ctrl Pts',(-30.,-3.88513632143196,-2.05009512650469));
#31614=CARTESIAN_POINT('Ctrl Pts',(-30.,-3.87226806614249,-2.06952493918974));
#31615=CARTESIAN_POINT('Ctrl Pts',(-30.,-3.8625180853102,-2.08424646102723));
#31616=CARTESIAN_POINT('Ctrl Pts',(-30.,-3.85267751973718,-2.09891297868158));
#31617=CARTESIAN_POINT('Ctrl Pts',(-30.,-3.84275441273704,-2.11351248267563));
#31618=CARTESIAN_POINT('Ctrl Pts',(-30.,-3.76866004569854,-2.22252481192893));
#31619=CARTESIAN_POINT('Ctrl Pts',(-30.,-3.68986014466549,-2.32796611537092));
#31620=CARTESIAN_POINT('Ctrl Pts',(-30.,-3.60658842790908,-2.42951355313142));
#31621=CARTESIAN_POINT('Ctrl Pts',(-30.,-3.52423619248041,-2.52993971014333));
#31622=CARTESIAN_POINT('Ctrl Pts',(-30.,-3.43750975231292,-2.62655802487046));
#31623=CARTESIAN_POINT('Ctrl Pts',(-30.,-3.34660114632163,-2.71901920330891));
#31624=CARTESIAN_POINT('Ctrl Pts',(-30.,-3.26049065975227,-2.8066003181802));
#31625=CARTESIAN_POINT('Ctrl Pts',(-30.,-3.1706272005035,-2.8904516534147));
#31626=CARTESIAN_POINT('Ctrl Pts',(-30.,-3.07715232424116,-2.97023901552393));
#31627=CARTESIAN_POINT('Ctrl Pts',(-30.,-3.01100240161384,-3.02670261345746));
#31628=CARTESIAN_POINT('Ctrl Pts',(-30.,-2.94304331188841,-3.0811300988234));
#31629=CARTESIAN_POINT('Ctrl Pts',(-30.,-2.87337762503368,-3.13344777611549));
#31630=CARTESIAN_POINT('Ctrl Pts',(-30.,-2.83651942594881,-3.1611276204169));
#31631=CARTESIAN_POINT('Ctrl Pts',(-30.,-2.79918348293621,-3.18821672602252));
#31632=CARTESIAN_POINT('Ctrl Pts',(-30.,-2.76138482187608,-3.21470302668161));
#31633=CARTESIAN_POINT('Ctrl Pts',(-30.,-2.74112373262897,-3.2289003894037));
#31634=CARTESIAN_POINT('Ctrl Pts',(-30.,-2.72072969185338,-3.24292453759925));
#31635=CARTESIAN_POINT('Ctrl Pts',(-30.,-2.70020500874655,-3.25677351535391));
#31636=CARTESIAN_POINT('Ctrl Pts',(-30.,-2.68589781217084,-3.26642725987592));
#31637=CARTESIAN_POINT('Ctrl Pts',(-30.,-2.67153139302699,-3.27599297571375));
#31638=CARTESIAN_POINT('Ctrl Pts',(-30.,-2.65711296641173,-3.2854660917133));
#31639=CARTESIAN_POINT('Ctrl Pts',(-30.,-2.54789875315275,-3.35722141832476));
#31640=CARTESIAN_POINT('Ctrl Pts',(-30.,-2.43559241880322,-3.42374262101484));
#31641=CARTESIAN_POINT('Ctrl Pts',(-30.,-2.32058110672905,-3.48486248573992));
#31642=CARTESIAN_POINT('Ctrl Pts',(-30.,-2.20823322648152,-3.54456693671123));
#31643=CARTESIAN_POINT('Ctrl Pts',(-30.,-2.09330331962513,-3.599117393161));
#31644=CARTESIAN_POINT('Ctrl Pts',(-30.,-1.97613528593933,-3.64830883882638));
#31645=CARTESIAN_POINT('Ctrl Pts',(-30.,-1.85480069740671,-3.69924955730885));
#31646=CARTESIAN_POINT('Ctrl Pts',(-30.,-1.73106514290719,-3.74444397765563));
#31647=CARTESIAN_POINT('Ctrl Pts',(-30.,-1.60530493978341,-3.7836051080115));
#31648=CARTESIAN_POINT('Ctrl Pts',(-30.,-1.48790451895484,-3.82016304183877));
#31649=CARTESIAN_POINT('Ctrl Pts',(-30.,-1.36873904140857,-3.8514627731731));
#31650=CARTESIAN_POINT('Ctrl Pts',(-30.,-1.24812048797374,-3.87721988828248));
#31651=CARTESIAN_POINT('Ctrl Pts',(-30.,-1.23953155072496,-3.87905398626397));
#31652=CARTESIAN_POINT('Ctrl Pts',(-30.,-1.23093525049353,-3.88085995890718));
#31653=CARTESIAN_POINT('Ctrl Pts',(-30.,-1.22233170237264,-3.88263769354994));
#31654=CARTESIAN_POINT('Ctrl Pts',(-31.3088415259036,-4.9251906134473,-0.000109311167407344));
#31655=CARTESIAN_POINT('Ctrl Pts',(-31.3026574105697,-4.92531380403982,
-0.127669621032252));
#31656=CARTESIAN_POINT('Ctrl Pts',(-31.2964732952358,-4.92045776407975,
-0.255220574660955));
#31657=CARTESIAN_POINT('Ctrl Pts',(-31.2902891799019,-4.91055613124801,
-0.382378634225134));
#31658=CARTESIAN_POINT('Ctrl Pts',(-31.2506528469036,-4.84709282324748,
-1.19738270840192));
#31659=CARTESIAN_POINT('Ctrl Pts',(-31.2110165139052,-4.57635592020155,
-1.99624664458159));
#31660=CARTESIAN_POINT('Ctrl Pts',(-31.1713801809069,-4.1312401814026,-2.681907808277));
#31661=CARTESIAN_POINT('Ctrl Pts',(-31.1317438479086,-3.68612444260365,
-3.36756897197242));
#31662=CARTESIAN_POINT('Ctrl Pts',(-31.0921075149103,-3.06662986805169,
-3.94002736318355));
#31663=CARTESIAN_POINT('Ctrl Pts',(-31.052471181912,-2.3480256147852,-4.32972871815496));
#31664=CARTESIAN_POINT('Ctrl Pts',(-31.0128348489136,-1.6294213615187,-4.71943007312636));
#31665=CARTESIAN_POINT('Ctrl Pts',(-30.9731985159153,-0.811707429537671,
-4.92637439185802));
#31666=CARTESIAN_POINT('Ctrl Pts',(-30.933562182917,0.00576326833122948,
-4.92541789298911));
#31667=CARTESIAN_POINT('Ctrl Pts',(-30.8939258499187,0.823233966200106,
-4.9244613941202));
#31668=CARTESIAN_POINT('Ctrl Pts',(-30.8542895169204,1.64046142995691,-4.71560407765069));
#31669=CARTESIAN_POINT('Ctrl Pts',(-30.814653183922,2.35815171375025,-4.32422202182277));
#31670=CARTESIAN_POINT('Ctrl Pts',(-30.7750168509237,3.07584199754363,-3.93283996599483));
#31671=CARTESIAN_POINT('Ctrl Pts',(-30.7353805179254,3.69399510137354,-3.35893317080848));
#31672=CARTESIAN_POINT('Ctrl Pts',(-30.6957441849271,4.13750506653447,-2.6722323509177));
#31673=CARTESIAN_POINT('Ctrl Pts',(-30.6561078519288,4.58101503169538,-1.98553153102693));
#31674=CARTESIAN_POINT('Ctrl Pts',(-30.6164715189305,4.84988185818724,-1.1860366864318));
#31675=CARTESIAN_POINT('Ctrl Pts',(-30.5768351859321,4.91143762165332,-0.370886072034668));
#31676=CARTESIAN_POINT('Ctrl Pts',(-30.5371988529338,4.97299338511941,0.444264542362484));
#31677=CARTESIAN_POINT('Ctrl Pts',(-30.4975625199355,4.82723808555968,1.27507092656169));
#31678=CARTESIAN_POINT('Ctrl Pts',(-30.4579261869371,4.49188185629875,2.02058724364277));
#31679=CARTESIAN_POINT('Ctrl Pts',(-30.4182898539388,4.15652562703785,2.76610356072381));
#31680=CARTESIAN_POINT('Ctrl Pts',(-30.3786535209405,3.63156846807577,3.42632981068678));
#31681=CARTESIAN_POINT('Ctrl Pts',(-30.3390171879422,2.98079166474727,3.92105218071421));
#31682=CARTESIAN_POINT('Ctrl Pts',(-30.2993808549439,2.33001486141874,4.41577455074166));
#31683=CARTESIAN_POINT('Ctrl Pts',(-30.2597445219456,1.55341841372378,4.74499304083354));
#31684=CARTESIAN_POINT('Ctrl Pts',(-30.2201081889472,0.745362402034862,
4.86869882773104));
#31685=CARTESIAN_POINT('Ctrl Pts',(-30.1804718559489,-0.0626936096540083,
4.99240461462853));
#31686=CARTESIAN_POINT('Ctrl Pts',(-30.1408355229506,-0.902209185336816,
4.91059769833167));
#31687=CARTESIAN_POINT('Ctrl Pts',(-30.1011991899523,-1.6711882943574,4.63323462455056));
#31688=CARTESIAN_POINT('Ctrl Pts',(-30.0674661266349,-2.32563887068767,
4.39718084706891));
#31689=CARTESIAN_POINT('Ctrl Pts',(-30.0337330633174,-2.92899916179811,
4.01948374188552));
#31690=CARTESIAN_POINT('Ctrl Pts',(-30.,-3.42895048616045,3.53554286219762));
#31691=CARTESIAN_POINT('',(-52.575,-2.3624802440062,-3.31498401464311));
#31692=CARTESIAN_POINT('Ctrl Pts',(-52.575,-2.36248024400613,-3.31498401464316));
#31693=CARTESIAN_POINT('Ctrl Pts',(-52.575,-2.45083842515724,-3.26474899095752));
#31694=CARTESIAN_POINT('Ctrl Pts',(-52.575,-2.53718350580222,-3.21123766039523));
#31695=CARTESIAN_POINT('Ctrl Pts',(-52.575,-2.62132193580694,-3.15455696157957));
#31696=CARTESIAN_POINT('Ctrl Pts',(-52.575,-2.72544813390243,-3.08441130194771));
#31697=CARTESIAN_POINT('Ctrl Pts',(-52.575,-2.82619583876697,-3.00941312765807));
#31698=CARTESIAN_POINT('Ctrl Pts',(-52.575,-2.92335409742353,-2.92992007978695));
#31699=CARTESIAN_POINT('Ctrl Pts',(-52.575,-2.97900323996874,-2.884389004884));
#31700=CARTESIAN_POINT('Ctrl Pts',(-52.575,-3.03347452971045,-2.83738238248389));
#31701=CARTESIAN_POINT('Ctrl Pts',(-52.575,-3.08672527840934,-2.78896043733211));
#31702=CARTESIAN_POINT('Ctrl Pts',(-52.575,-3.11397380637268,-2.76418281901225));
#31703=CARTESIAN_POINT('Ctrl Pts',(-52.575,-3.14090270788054,-2.73903453627563));
#31704=CARTESIAN_POINT('Ctrl Pts',(-52.575,-3.16750598016368,-2.71352319283678));
#31705=CARTESIAN_POINT('Ctrl Pts',(-52.575,-3.18459441820031,-2.69713614815498));
#31706=CARTESIAN_POINT('Ctrl Pts',(-52.575,-3.20154849591608,-2.68059929653958));
#31707=CARTESIAN_POINT('Ctrl Pts',(-52.575,-3.21836657574555,-2.66391458876838));
#31708=CARTESIAN_POINT('Ctrl Pts',(-52.575,-3.23304555953287,-2.6493520134118));
#31709=CARTESIAN_POINT('Ctrl Pts',(-52.575,-3.24761411042159,-2.63468357077931));
#31710=CARTESIAN_POINT('Ctrl Pts',(-52.575,-3.26207083882393,-2.61991143683803));
#31711=CARTESIAN_POINT('Ctrl Pts',(-52.575,-3.35252129885386,-2.527487599755));
#31712=CARTESIAN_POINT('Ctrl Pts',(-52.575,-3.43860302817434,-2.43100187945135));
#31713=CARTESIAN_POINT('Ctrl Pts',(-52.575,-3.52009386900591,-2.33082932389395));
#31714=CARTESIAN_POINT('Ctrl Pts',(-52.575,-3.60209138438908,-2.23003393902036));
#31715=CARTESIAN_POINT('Ctrl Pts',(-52.575,-3.67944139370459,-2.12550522054836));
#31716=CARTESIAN_POINT('Ctrl Pts',(-52.575,-3.75189018667931,-2.01758011205502));
#31717=CARTESIAN_POINT('Ctrl Pts',(-52.575,-3.77730845597078,-1.97971516830155));
#31718=CARTESIAN_POINT('Ctrl Pts',(-52.575,-3.80212313369375,-1.94143178856851));
#31719=CARTESIAN_POINT('Ctrl Pts',(-52.575,-3.82632223974423,-1.90274340160315));
#31720=CARTESIAN_POINT('Ctrl Pts',(-52.575,-3.84913245184897,-1.86627551263115));
#31721=CARTESIAN_POINT('Ctrl Pts',(-52.575,-3.87139572307394,-1.82944776587887));
#31722=CARTESIAN_POINT('Ctrl Pts',(-52.575,-3.89310152313127,-1.79227099068793));
#31723=CARTESIAN_POINT('Ctrl Pts',(-52.575,-3.90322370392622,-1.77493414805314));
#31724=CARTESIAN_POINT('Ctrl Pts',(-52.575,-3.91321999890863,-1.75752932486574));
#31725=CARTESIAN_POINT('Ctrl Pts',(-52.575,-3.92308811855202,-1.74006057784368));
#31726=CARTESIAN_POINT('Ctrl Pts',(-52.575,-3.95009373716041,-1.69225467999363));
#31727=CARTESIAN_POINT('Ctrl Pts',(-52.575,-3.97614326297851,-1.643963649635));
#31728=CARTESIAN_POINT('Ctrl Pts',(-52.575,-4.00122119219861,-1.59521504644078));
#31729=CARTESIAN_POINT('Ctrl Pts',(-52.575,-4.06049526868924,-1.47999307539268));
#31730=CARTESIAN_POINT('Ctrl Pts',(-52.575,-4.11434405528511,-1.36221753728262));
#31731=CARTESIAN_POINT('Ctrl Pts',(-52.575,-4.16278066252525,-1.24231802685534));
#31732=CARTESIAN_POINT('Ctrl Pts',(-52.575,-4.21199575328309,-1.12049146583625));
#31733=CARTESIAN_POINT('Ctrl Pts',(-52.575,-4.25562365155741,-0.996471504820113));
#31734=CARTESIAN_POINT('Ctrl Pts',(-52.575,-4.29363801884489,-0.870672911911608));
#31735=CARTESIAN_POINT('Ctrl Pts',(-52.575,-4.32788618697962,-0.757337568764584));
#31736=CARTESIAN_POINT('Ctrl Pts',(-52.575,-4.35757764642574,-0.642557729992402));
#31737=CARTESIAN_POINT('Ctrl Pts',(-52.575,-4.38266242226516,-0.526618827435207));
#31738=CARTESIAN_POINT('Ctrl Pts',(-52.575,-4.40147600414472,-0.43966465051731));
#31739=CARTESIAN_POINT('Ctrl Pts',(-52.575,-4.41769774414857,-0.352058115046802));
#31740=CARTESIAN_POINT('Ctrl Pts',(-52.575,-4.43129495642288,-0.263915699110775));
#31741=CARTESIAN_POINT('Ctrl Pts',(-52.575,-4.43428275677774,-0.244547615690493));
#31742=CARTESIAN_POINT('Ctrl Pts',(-52.575,-4.43714379477229,-0.225153648965712));
#31743=CARTESIAN_POINT('Ctrl Pts',(-52.575,-4.43987765592149,-0.205735021774693));
#31744=CARTESIAN_POINT('Ctrl Pts',(-52.575,-4.44260798913829,-0.186341453502313));
#31745=CARTESIAN_POINT('Ctrl Pts',(-52.575,-4.44521045926173,-0.166930227795076));
#31746=CARTESIAN_POINT('Ctrl Pts',(-52.575,-4.44768395086165,-0.147510951408631));
#31747=CARTESIAN_POINT('Ctrl Pts',(-52.575,-4.46489548234348,-0.0123839564793861));
#31748=CARTESIAN_POINT('Ctrl Pts',(-52.575,-4.47588307079217,0.123253805094162));
#31749=CARTESIAN_POINT('Ctrl Pts',(-52.575,-4.48063897431675,0.258956414548593));
#31750=CARTESIAN_POINT('Ctrl Pts',(-52.575,-4.48385862007716,0.350824201384031));
#31751=CARTESIAN_POINT('Ctrl Pts',(-52.575,-4.48422139979451,0.442722422791573));
#31752=CARTESIAN_POINT('Ctrl Pts',(-52.575,-4.48171295534441,0.534519045515166));
#31753=CARTESIAN_POINT('Ctrl Pts',(-52.575,-4.47802927241361,0.669323566388171));
#31754=CARTESIAN_POINT('Ctrl Pts',(-52.575,-4.46815625725434,0.803908860906131));
#31755=CARTESIAN_POINT('Ctrl Pts',(-52.575,-4.45227140210682,0.937896967744017));
#31756=CARTESIAN_POINT('Ctrl Pts',(-52.575,-4.43625287788906,1.07301256775057));
#31757=CARTESIAN_POINT('Ctrl Pts',(-52.575,-4.41412086946338,1.20752165052657));
#31758=CARTESIAN_POINT('Ctrl Pts',(-52.575,-4.38600460743474,1.3410398419735));
#31759=CARTESIAN_POINT('Ctrl Pts',(-52.575,-4.37816899892792,1.37824949223395));
#31760=CARTESIAN_POINT('Ctrl Pts',(-52.575,-4.36986830738069,1.41538216450086));
#31761=CARTESIAN_POINT('Ctrl Pts',(-52.575,-4.36110461497015,1.45242945648354));
#31762=CARTESIAN_POINT('Ctrl Pts',(-52.575,-4.35581207705533,1.47480292513971));
#31763=CARTESIAN_POINT('Ctrl Pts',(-52.575,-4.35035066978824,1.49714525323282));
#31764=CARTESIAN_POINT('Ctrl Pts',(-52.575,-4.34472079756005,1.51945457780506));
#31765=CARTESIAN_POINT('Ctrl Pts',(-52.575,-4.33978278713431,1.53902228251733));
#31766=CARTESIAN_POINT('Ctrl Pts',(-52.575,-4.33471471620666,1.55856607009609));
#31767=CARTESIAN_POINT('Ctrl Pts',(-52.575,-4.32952186708747,1.57806649096184));
#31768=CARTESIAN_POINT('Ctrl Pts',(-52.575,-4.29379030157313,1.7122472749072));
#31769=CARTESIAN_POINT('Ctrl Pts',(-52.575,-4.25210787632114,1.8445664661999));
#31770=CARTESIAN_POINT('Ctrl Pts',(-52.575,-4.2046945955001,1.97463033236496));
#31771=CARTESIAN_POINT('Ctrl Pts',(-52.575,-4.15669273431461,2.10630878913467));
#31772=CARTESIAN_POINT('Ctrl Pts',(-52.575,-4.10281680514146,2.2356763657865));
#31773=CARTESIAN_POINT('Ctrl Pts',(-52.575,-4.04324167749382,2.36232823147581));
#31774=CARTESIAN_POINT('Ctrl Pts',(-52.575,-3.98430004740198,2.48763333299492));
#31775=CARTESIAN_POINT('Ctrl Pts',(-52.575,-3.91977954437028,2.61028094909734));
#31776=CARTESIAN_POINT('Ctrl Pts',(-52.575,-3.84979995958599,2.72987096421517));
#31777=CARTESIAN_POINT('Ctrl Pts',(-52.575,-3.79916663882266,2.81639962274062));
#31778=CARTESIAN_POINT('Ctrl Pts',(-52.575,-3.74567435543154,2.90132744181084));
#31779=CARTESIAN_POINT('Ctrl Pts',(-52.575,-3.68943437806386,2.98455695852906));
#31780=CARTESIAN_POINT('Ctrl Pts',(-52.575,-3.66455066574735,3.0213823529761));
#31781=CARTESIAN_POINT('Ctrl Pts',(-52.575,-3.63912888080377,3.05787519175057));
#31782=CARTESIAN_POINT('Ctrl Pts',(-52.575,-3.61317791043782,3.09402659330026));
#31783=CARTESIAN_POINT('Ctrl Pts',(-52.575,-3.5984365124608,3.11456232626731));
#31784=CARTESIAN_POINT('Ctrl Pts',(-52.575,-3.58352434957018,3.13498787947549));
#31785=CARTESIAN_POINT('Ctrl Pts',(-52.575,-3.56844298859188,3.15530158081671));
#31786=CARTESIAN_POINT('Ctrl Pts',(-52.575,-3.55715242145521,3.17050930703699));
#31787=CARTESIAN_POINT('Ctrl Pts',(-52.575,-3.54576681267099,3.18565452567972));
#31788=CARTESIAN_POINT('Ctrl Pts',(-52.575,-3.53429612334896,3.20072456181671));
#31789=CARTESIAN_POINT('Ctrl Pts',(-52.575,-3.44911973336135,3.31262814834888));
#31790=CARTESIAN_POINT('Ctrl Pts',(-52.575,-3.35913530229149,3.42055165052906));
#31791=CARTESIAN_POINT('Ctrl Pts',(-52.575,-3.26472470398113,3.5242711902548));
#31792=CARTESIAN_POINT('Ctrl Pts',(-52.575,-3.168304243029,3.63019876627992));
#31793=CARTESIAN_POINT('Ctrl Pts',(-52.575,-3.0672668488026,3.73174212442733));
#31794=CARTESIAN_POINT('Ctrl Pts',(-52.575,-2.9619683093501,3.82864474738118));
#31795=CARTESIAN_POINT('Ctrl Pts',(-52.575,-2.85628308759516,3.92590322075376));
#31796=CARTESIAN_POINT('Ctrl Pts',(-52.575,-2.74630488841782,4.0184874465719));
#31797=CARTESIAN_POINT('Ctrl Pts',(-52.575,-2.63234878081027,4.10611049349789));
#31798=CARTESIAN_POINT('Ctrl Pts',(-52.575,-2.51936354614263,4.1929870175129));
#31799=CARTESIAN_POINT('Ctrl Pts',(-52.575,-2.40246734548989,4.2749871084609));
#31800=CARTESIAN_POINT('Ctrl Pts',(-52.575,-2.28193125768585,4.35179515368219));
#31801=CARTESIAN_POINT('Ctrl Pts',(-52.575,-2.24443605083211,4.3756878616344));
#31802=CARTESIAN_POINT('Ctrl Pts',(-52.575,-2.20658839941422,4.39907786480192));
#31803=CARTESIAN_POINT('Ctrl Pts',(-52.575,-2.16839587231069,4.42195480991676));
#31804=CARTESIAN_POINT('Ctrl Pts',(-52.575,-2.3624802440062,-3.31498401464311));
#31805=CARTESIAN_POINT('Ctrl Pts',(-52.5412669366826,-1.89383403051946,
-3.64828975900151));
#31806=CARTESIAN_POINT('Ctrl Pts',(-52.4678975403668,-0.719464420527365,
-4.15646543436434));
#31807=CARTESIAN_POINT('Ctrl Pts',(-52.3548918110528,1.26526436602798,-4.04962642367063));
#31808=CARTESIAN_POINT('Ctrl Pts',(-52.2359828120578,3.04621665534188,-2.95311079097194));
#31809=CARTESIAN_POINT('Ctrl Pts',(-52.1170738130628,4.08693027247079,-1.13899868529834));
#31810=CARTESIAN_POINT('Ctrl Pts',(-51.9981648140679,4.13451401645655,0.951899429035897));
#31811=CARTESIAN_POINT('Ctrl Pts',(-51.8792558150729,3.17740293277235,2.81148063819688));
#31812=CARTESIAN_POINT('Ctrl Pts',(-51.760346816078,1.44817770563431,3.98786896704909));
#31813=CARTESIAN_POINT('Ctrl Pts',(-51.641437817083,-0.632957411871854,
4.19519722352873));
#31814=CARTESIAN_POINT('Ctrl Pts',(-51.522528818088,-2.56028268385088,3.38308566467023));
#31815=CARTESIAN_POINT('Ctrl Pts',(-51.4094453227024,-3.80151277026337,
1.82894004028097));
#31816=CARTESIAN_POINT('Ctrl Pts',(-51.3359981603151,-4.07013175620066,
0.576320675082573));
#31817=CARTESIAN_POINT('Ctrl Pts',(-51.3021873309261,-4.07067545460402,
-8.70709198036793E-5));
#31818=CARTESIAN_POINT('Origin',(-52.575,-4.52129938221115E-16,0.));
#31819=CARTESIAN_POINT('',(-52.575,-4.925,-6.03138548580072E-16));
#31820=CARTESIAN_POINT('Origin',(-52.575,0.,0.));
#31821=CARTESIAN_POINT('Origin',(-52.575,0.,0.));
#31822=CARTESIAN_POINT('',(-52.575,2.36230756092333,-3.31488661006745));
#31823=CARTESIAN_POINT('Ctrl Pts',(-52.575,2.16858289183278,4.42210503781149));
#31824=CARTESIAN_POINT('Ctrl Pts',(-52.575,2.27324543867332,4.35954461344517));
#31825=CARTESIAN_POINT('Ctrl Pts',(-52.575,2.37542046052859,4.29314920151771));
#31826=CARTESIAN_POINT('Ctrl Pts',(-52.575,2.47486626316976,4.22298837806258));
#31827=CARTESIAN_POINT('Ctrl Pts',(-52.575,2.59306038724079,4.13960027266106));
#31828=CARTESIAN_POINT('Ctrl Pts',(-52.575,2.70740051443753,4.05089352006367));
#31829=CARTESIAN_POINT('Ctrl Pts',(-52.575,2.81758791907416,3.95719317432484));
#31830=CARTESIAN_POINT('Ctrl Pts',(-52.575,2.88224740587185,3.90220852078646));
#31831=CARTESIAN_POINT('Ctrl Pts',(-52.575,2.94547616306427,3.84550366688624));
#31832=CARTESIAN_POINT('Ctrl Pts',(-52.575,3.00720683632612,3.78713970701225));
#31833=CARTESIAN_POINT('Ctrl Pts',(-52.575,3.0504874052719,3.74621960593771));
#31834=CARTESIAN_POINT('Ctrl Pts',(-52.575,3.09303145431524,3.70448387254875));
#31835=CARTESIAN_POINT('Ctrl Pts',(-52.575,3.13481408960903,3.66195279787687));
#31836=CARTESIAN_POINT('Ctrl Pts',(-52.575,3.15648069704987,3.63989808322154));
#31837=CARTESIAN_POINT('Ctrl Pts',(-52.575,3.17794569325268,3.61762601164362));
#31838=CARTESIAN_POINT('Ctrl Pts',(-52.575,3.19918545204692,3.59516093882889));
#31839=CARTESIAN_POINT('Ctrl Pts',(-52.575,3.29689976205027,3.4918095255416));
#31840=CARTESIAN_POINT('Ctrl Pts',(-52.575,3.38992792061982,3.38429932195033));
#31841=CARTESIAN_POINT('Ctrl Pts',(-52.575,3.47798443456353,3.27294401601918));
#31842=CARTESIAN_POINT('Ctrl Pts',(-52.575,3.56533656591254,3.16247946462524));
#31843=CARTESIAN_POINT('Ctrl Pts',(-52.575,3.64779664533402,3.04823040929176));
#31844=CARTESIAN_POINT('Ctrl Pts',(-52.575,3.72504020298562,2.9304807933875));
#31845=CARTESIAN_POINT('Ctrl Pts',(-52.575,3.7786407807849,2.84877239413719));
#31846=CARTESIAN_POINT('Ctrl Pts',(-52.575,3.82972855358387,2.76537793963324));
#31847=CARTESIAN_POINT('Ctrl Pts',(-52.575,3.87818054873119,2.68038844930736));
#31848=CARTESIAN_POINT('Ctrl Pts',(-52.575,3.88822812521621,2.66276402740532));
#31849=CARTESIAN_POINT('Ctrl Pts',(-52.575,3.89816231179414,2.64507100689568));
#31850=CARTESIAN_POINT('Ctrl Pts',(-52.575,3.90798194266676,2.62731018963255));
#31851=CARTESIAN_POINT('Ctrl Pts',(-52.575,3.91756756129971,2.60997263152042));
#31852=CARTESIAN_POINT('Ctrl Pts',(-52.575,3.92703894769771,2.5925796412082));
#31853=CARTESIAN_POINT('Ctrl Pts',(-52.575,3.93639533109687,2.57513219119634));
#31854=CARTESIAN_POINT('Ctrl Pts',(-52.575,3.96367451327325,2.52426294534762));
#31855=CARTESIAN_POINT('Ctrl Pts',(-52.575,3.98997637187834,2.47293052215805));
#31856=CARTESIAN_POINT('Ctrl Pts',(-52.575,4.01528228820605,2.42115597945716));
#31857=CARTESIAN_POINT('Ctrl Pts',(-52.575,4.07614892166724,2.29662612357737));
#31858=CARTESIAN_POINT('Ctrl Pts',(-52.575,4.13125737282119,2.16953962378044));
#31859=CARTESIAN_POINT('Ctrl Pts',(-52.575,4.1805437519518,2.0403132293574));
#31860=CARTESIAN_POINT('Ctrl Pts',(-52.575,4.22997373559905,1.91071031115163));
#31861=CARTESIAN_POINT('Ctrl Pts',(-52.575,4.27354777659503,1.77895418493233));
#31862=CARTESIAN_POINT('Ctrl Pts',(-52.575,4.31115013628448,1.64545567277246));
#31863=CARTESIAN_POINT('Ctrl Pts',(-52.575,4.34817398830438,1.51401101876923));
#31864=CARTESIAN_POINT('Ctrl Pts',(-52.575,4.37940844584972,1.38087641354689));
#31865=CARTESIAN_POINT('Ctrl Pts',(-52.575,4.40469318296196,1.24644656007076));
#31866=CARTESIAN_POINT('Ctrl Pts',(-52.575,4.42089893755181,1.16028639137634));
#31867=CARTESIAN_POINT('Ctrl Pts',(-52.575,4.43465959569322,1.0735942307477));
#31868=CARTESIAN_POINT('Ctrl Pts',(-52.575,4.44592201924774,0.986476727243181));
#31869=CARTESIAN_POINT('Ctrl Pts',(-52.575,4.44839087427289,0.967379551110164));
#31870=CARTESIAN_POINT('Ctrl Pts',(-52.575,4.45073964677597,0.948261947204026));
#31871=CARTESIAN_POINT('Ctrl Pts',(-52.575,4.45296772135315,0.929125059904503));
#31872=CARTESIAN_POINT('Ctrl Pts',(-52.575,4.45503253428023,0.911390423602443));
#31873=CARTESIAN_POINT('Ctrl Pts',(-52.575,4.45699252464179,0.893649215236444));
#31874=CARTESIAN_POINT('Ctrl Pts',(-52.575,4.45884750535299,0.8759027682724));
#31875=CARTESIAN_POINT('Ctrl Pts',(-52.575,4.47288219592637,0.741634044929663));
#31876=CARTESIAN_POINT('Ctrl Pts',(-52.575,4.48091097969341,0.607056985697511));
#31877=CARTESIAN_POINT('Ctrl Pts',(-52.575,4.4828462748776,0.472553339734528));
#31878=CARTESIAN_POINT('Ctrl Pts',(-52.575,4.48415655129386,0.381488701819775));
#31879=CARTESIAN_POINT('Ctrl Pts',(-52.575,4.4826725944393,0.290457608534688));
#31880=CARTESIAN_POINT('Ctrl Pts',(-52.575,4.4783536900286,0.19957981697436));
#31881=CARTESIAN_POINT('Ctrl Pts',(-52.575,4.47194675885048,0.0647660538580273));
#31882=CARTESIAN_POINT('Ctrl Pts',(-52.575,4.45930309571538,-0.0697115117325435));
#31883=CARTESIAN_POINT('Ctrl Pts',(-52.575,4.44051793802534,-0.203434251933974));
#31884=CARTESIAN_POINT('Ctrl Pts',(-52.575,4.42188439250804,-0.336077736080069));
#31885=CARTESIAN_POINT('Ctrl Pts',(-52.575,4.39720771395406,-0.467979255925283));
#31886=CARTESIAN_POINT('Ctrl Pts',(-52.575,4.36653652929021,-0.598704962823127));
#31887=CARTESIAN_POINT('Ctrl Pts',(-52.575,4.35826910408269,-0.633942108578089));
#31888=CARTESIAN_POINT('Ctrl Pts',(-52.575,4.34956590074294,-0.66909364602887));
#31889=CARTESIAN_POINT('Ctrl Pts',(-52.575,4.34042736750284,-0.704150655988287));
#31890=CARTESIAN_POINT('Ctrl Pts',(-52.575,4.33455267477135,-0.726687003582102));
#31891=CARTESIAN_POINT('Ctrl Pts',(-52.575,4.32849807591017,-0.749184283359156));
#31892=CARTESIAN_POINT('Ctrl Pts',(-52.575,4.32226364568102,-0.77164008078128));
#31893=CARTESIAN_POINT('Ctrl Pts',(-52.575,4.31754011549755,-0.788653766558259));
#31894=CARTESIAN_POINT('Ctrl Pts',(-52.575,4.31271343970828,-0.805643132465032));
#31895=CARTESIAN_POINT('Ctrl Pts',(-52.575,4.3077875565571,-0.822594272316468));
#31896=CARTESIAN_POINT('Ctrl Pts',(-52.575,4.27100624199071,-0.949167556334511));
#31897=CARTESIAN_POINT('Ctrl Pts',(-52.575,4.22864619087658,-1.07379868233084));
#31898=CARTESIAN_POINT('Ctrl Pts',(-52.575,4.18082992080759,-1.19610839048349));
#31899=CARTESIAN_POINT('Ctrl Pts',(-52.575,4.1335416210436,-1.31706759819301));
#31900=CARTESIAN_POINT('Ctrl Pts',(-52.575,4.08091651537112,-1.43575703633188));
#31901=CARTESIAN_POINT('Ctrl Pts',(-52.575,4.02302930721789,-1.55178516490185));
#31902=CARTESIAN_POINT('Ctrl Pts',(-52.575,3.96819756105823,-1.66168897778376));
#31903=CARTESIAN_POINT('Ctrl Pts',(-52.575,3.90864399407258,-1.76920531054976));
#31904=CARTESIAN_POINT('Ctrl Pts',(-52.575,3.84439996309285,-1.87397258856179));
#31905=CARTESIAN_POINT('Ctrl Pts',(-52.575,3.79893585979599,-1.9481141123272));
#31906=CARTESIAN_POINT('Ctrl Pts',(-52.575,3.75112194501686,-2.02087824453719));
#31907=CARTESIAN_POINT('Ctrl Pts',(-52.575,3.70103299493048,-2.09216319996224));
#31908=CARTESIAN_POINT('Ctrl Pts',(-52.575,3.67453230440468,-2.1298781159189));
#31909=CARTESIAN_POINT('Ctrl Pts',(-52.575,3.6473947043283,-2.16717883751779));
#31910=CARTESIAN_POINT('Ctrl Pts',(-52.575,3.61963075641688,-2.20404924569613));
#31911=CARTESIAN_POINT('Ctrl Pts',(-52.575,3.60474852672729,-2.22381278526946));
#31912=CARTESIAN_POINT('Ctrl Pts',(-52.575,3.58968632609275,-2.2434526722059));
#31913=CARTESIAN_POINT('Ctrl Pts',(-52.575,3.57444574627334,-2.26296633271248));
#31914=CARTESIAN_POINT('Ctrl Pts',(-52.575,3.56382195463694,-2.27656877210399));
#31915=CARTESIAN_POINT('Ctrl Pts',(-52.575,3.55311463654801,-2.29010579189593));
#31916=CARTESIAN_POINT('Ctrl Pts',(-52.575,3.54232924135416,-2.30357081513136));
#31917=CARTESIAN_POINT('Ctrl Pts',(-52.575,3.46063398202519,-2.4055632359298));
#31918=CARTESIAN_POINT('Ctrl Pts',(-52.575,3.3743805109152,-2.50353323130147));
#31919=CARTESIAN_POINT('Ctrl Pts',(-52.575,3.28388534939653,-2.59720213470236));
#31920=CARTESIAN_POINT('Ctrl Pts',(-52.575,3.19548588962452,-2.68870183832316));
#31921=CARTESIAN_POINT('Ctrl Pts',(-52.575,3.10303810752968,-2.77609769489524));
#31922=CARTESIAN_POINT('Ctrl Pts',(-52.575,3.00680571587098,-2.85908844917917));
#31923=CARTESIAN_POINT('Ctrl Pts',(-52.575,2.90715122652406,-2.94503041836574));
#31924=CARTESIAN_POINT('Ctrl Pts',(-52.575,2.80343757806056,-3.02624927085457));
#31925=CARTESIAN_POINT('Ctrl Pts',(-52.575,2.6959339822994,-3.10235576984184));
#31926=CARTESIAN_POINT('Ctrl Pts',(-52.575,2.59557664254627,-3.17340312153467));
#31927=CARTESIAN_POINT('Ctrl Pts',(-52.575,2.49191576181343,-3.2399950596289));
#31928=CARTESIAN_POINT('Ctrl Pts',(-52.575,2.38516016083428,-3.30176468148191));
#31929=CARTESIAN_POINT('Ctrl Pts',(-52.575,2.37755829676769,-3.30616317921379));
#31930=CARTESIAN_POINT('Ctrl Pts',(-52.575,2.36994073858172,-3.31053720298181));
#31931=CARTESIAN_POINT('Ctrl Pts',(-52.575,2.36230756092339,-3.31488661006741));
#31932=CARTESIAN_POINT('Origin',(-52.575,0.,0.));
#31933=CARTESIAN_POINT('Origin',(-55.3478126690739,0.,0.));
#31934=CARTESIAN_POINT('Ctrl Pts',(-52.575,2.36230756092333,-3.31488661006745));
#31935=CARTESIAN_POINT('Ctrl Pts',(-52.5353636670017,2.91267249451488,-2.92267674082431));
#31936=CARTESIAN_POINT('Ctrl Pts',(-52.456091001005,3.81372197207604,-1.85922435845946));
#31937=CARTESIAN_POINT('Ctrl Pts',(-52.3371820020101,4.2384739899776,0.188973964574656));
#31938=CARTESIAN_POINT('Ctrl Pts',(-52.2182730030151,3.63326518569111,2.1907646706185));
#31939=CARTESIAN_POINT('Ctrl Pts',(-52.0993640040202,2.14517071451495,3.66043213853357));
#31940=CARTESIAN_POINT('Ctrl Pts',(-51.9804550050252,0.135793741969793,
4.240490317549));
#31941=CARTESIAN_POINT('Ctrl Pts',(-51.8615460060302,-1.90658020276247,
3.79016093772832));
#31942=CARTESIAN_POINT('Ctrl Pts',(-51.7426370070353,-3.48565239142985,
2.41878623204276));
#31943=CARTESIAN_POINT('Ctrl Pts',(-51.6547258947165,-4.02686902757588,
0.970374196809295));
#31944=CARTESIAN_POINT('Ctrl Pts',(-51.606451115396,-4.07067915096537,0.147388340486156));
#31945=CARTESIAN_POINT('Ctrl Pts',(-51.5978126690739,-4.07052776695671,
0.00010449757507032));
#31946=CARTESIAN_POINT('Ctrl Pts',(-53.0683458050225,2.85821514250023,-4.01076441581681));
#31947=CARTESIAN_POINT('Ctrl Pts',(-53.0287094720242,3.52411547364834,-3.53621986207098));
#31948=CARTESIAN_POINT('Ctrl Pts',(-52.9494368060276,4.6143178264278,-2.24952216322641));
#31949=CARTESIAN_POINT('Ctrl Pts',(-52.8305278070326,5.12823594168768,0.228644337435172));
#31950=CARTESIAN_POINT('Ctrl Pts',(-52.7116188080377,4.3959786364154,2.65066109883206));
#31951=CARTESIAN_POINT('Ctrl Pts',(-52.5927098090426,2.59549582827328,4.42884861375204));
#31952=CARTESIAN_POINT('Ctrl Pts',(-52.4738008100477,0.16430025284401,5.13067554696692));
#31953=CARTESIAN_POINT('Ctrl Pts',(-52.3548918110528,-2.30681918648935,
4.58581074028058));
#31954=CARTESIAN_POINT('Ctrl Pts',(-52.2359828120578,-4.21737821589285,
2.92655010264362));
#31955=CARTESIAN_POINT('Ctrl Pts',(-52.1170738130628,-5.1031065981609,0.556150593197082));
#31956=CARTESIAN_POINT('Ctrl Pts',(-51.9981648140679,-4.74877130744063,
-1.94940347214282));
#31957=CARTESIAN_POINT('Ctrl Pts',(-51.8792558150729,-3.24047617807803,
-3.9812445731161));
#31958=CARTESIAN_POINT('Ctrl Pts',(-51.760346816078,-0.944739701634101,
-5.04563852186393));
#31959=CARTESIAN_POINT('Ctrl Pts',(-51.641437817083,1.58057020018507,-4.88393233495926));
#31960=CARTESIAN_POINT('Ctrl Pts',(-51.522528818088,3.72179876201096,-3.53542259729576));
#31961=CARTESIAN_POINT('Ctrl Pts',(-51.4036198190931,4.95862370685834,-1.32779868772642));
#31962=CARTESIAN_POINT('Ctrl Pts',(-51.2847108200981,4.99049439700665,1.20248248786643));
#31963=CARTESIAN_POINT('Ctrl Pts',(-51.1658018211031,3.80966620304533,3.44055838262431));
#31964=CARTESIAN_POINT('Ctrl Pts',(-51.0468928221082,1.70308244370534,4.8425725242518));
#31965=CARTESIAN_POINT('Ctrl Pts',(-50.9279838231132,-0.817353334162299,
5.06783307265007));
#31966=CARTESIAN_POINT('Ctrl Pts',(-50.8090748241183,-3.13917081939765,
4.06160129283451));
#31967=CARTESIAN_POINT('Ctrl Pts',(-50.6901658251233,-4.69816429329073,
2.06839328444175));
#31968=CARTESIAN_POINT('Ctrl Pts',(-50.5712568261283,-5.11549560931122,
-0.427437919675575));
#31969=CARTESIAN_POINT('Ctrl Pts',(-50.4523478271334,-4.28975252612823,
-2.81940095899504));
#31970=CARTESIAN_POINT('Ctrl Pts',(-50.3334388281384,-2.42159206029875,
-4.52624462417659));
#31971=CARTESIAN_POINT('Ctrl Pts',(-50.2145298291435,0.0350195206030677,
-5.1332029120825));
#31972=CARTESIAN_POINT('Ctrl Pts',(-50.0956208301484,2.48312129661556,-4.49278389533952));
#31973=CARTESIAN_POINT('Ctrl Pts',(-49.9767118311536,4.32782024529306,-2.76061051728878));
#31974=CARTESIAN_POINT('Ctrl Pts',(-49.8578028321585,5.12085128883261,-0.357603944948157));
#31975=CARTESIAN_POINT('Ctrl Pts',(-49.7388938331636,4.6695064936802,2.13230101281847));
#31976=CARTESIAN_POINT('Ctrl Pts',(-49.6199848341686,3.08346343614612,4.10405308709817));
#31977=CARTESIAN_POINT('Ctrl Pts',(-49.5010758351737,0.748133359127894,
5.07851306789146));
#31978=CARTESIAN_POINT('Ctrl Pts',(-49.3821668361787,-1.76899443543955,
4.81888547188666));
#31979=CARTESIAN_POINT('Ctrl Pts',(-49.2632578371838,-3.85625348161299,
3.38826025997524));
#31980=CARTESIAN_POINT('Ctrl Pts',(-49.1443488381888,-5.00643617275599,
1.13428186615986));
#31981=CARTESIAN_POINT('Ctrl Pts',(-49.0254398391939,-4.94004609895293,
-1.39532900922998));
#31982=CARTESIAN_POINT('Ctrl Pts',(-48.9065308401988,-3.6732161645023,-3.58587248973217));
#31983=CARTESIAN_POINT('Ctrl Pts',(-48.787621841204,-1.51378826389541,-4.90504267013768));
#31984=CARTESIAN_POINT('Ctrl Pts',(-48.6687128422089,1.01349283811091,-5.03227888444955));
#31985=CARTESIAN_POINT('Ctrl Pts',(-48.549803843214,3.29449340406979,-3.93666250957833));
#31986=CARTESIAN_POINT('Ctrl Pts',(-48.430894844219,4.77492629845893,-1.88443024494519));
#31987=CARTESIAN_POINT('Ctrl Pts',(-48.3119858452241,5.09504373313213,0.625721872120406));
#31988=CARTESIAN_POINT('Ctrl Pts',(-48.1930768462291,4.17705661038212,2.98382247753481));
#31989=CARTESIAN_POINT('Ctrl Pts',(-48.0741678472341,2.24403741002721,4.61684899105194));
#31990=CARTESIAN_POINT('Ctrl Pts',(-47.9552588482392,-0.234286814171907,
5.12797310762099));
#31991=CARTESIAN_POINT('Ctrl Pts',(-47.8363498492442,-2.65567893188406,
4.39299077104949));
#31992=CARTESIAN_POINT('Ctrl Pts',(-47.7174408502493,-4.43173641444143,
2.59050397735512));
#31993=CARTESIAN_POINT('Ctrl Pts',(-47.5985318512543,-5.13087418062076,
0.158520176691056));
#31994=CARTESIAN_POINT('Ctrl Pts',(-47.4796228522593,-4.58320052783577,
-2.31198430475313));
#31995=CARTESIAN_POINT('Ctrl Pts',(-47.3607138532644,-2.92180111364115,
-4.22067254784166));
#31996=CARTESIAN_POINT('Ctrl Pts',(-47.2418048542695,-0.55039890768255,
-5.10372996407537));
#31997=CARTESIAN_POINT('Ctrl Pts',(-47.1228958552744,1.95475119754748,-4.74657205354196));
#31998=CARTESIAN_POINT('Ctrl Pts',(-47.0039868562796,3.98489333560856,-3.23598881450499));
#31999=CARTESIAN_POINT('Ctrl Pts',(-46.8850778572845,5.04669940864642,-0.93905462170567));
#32000=CARTESIAN_POINT('Ctrl Pts',(-46.7661688582896,4.88214867984596,1.58607149008397));
#32001=CARTESIAN_POINT('Ctrl Pts',(-46.6472598592946,3.53122726471987,3.72577944981691));
#32002=CARTESIAN_POINT('Ctrl Pts',(-46.5283508602996,1.3222114349539,4.96011647293244));
#32003=CARTESIAN_POINT('Ctrl Pts',(-46.4094418613047,-1.20810409099495,
4.98913649934544));
#32004=CARTESIAN_POINT('Ctrl Pts',(-46.2905328623097,-3.44484820534307,
3.80578761177265));
#32005=CARTESIAN_POINT('Ctrl Pts',(-46.1716238633147,-4.84448816787985,
1.69762566399454));
#32006=CARTESIAN_POINT('Ctrl Pts',(-46.0527148643198,-5.06690901450728,
-0.823062295626789));
#32007=CARTESIAN_POINT('Ctrl Pts',(-45.9338058653248,-4.05806208965098,
-3.14374467479683));
#32008=CARTESIAN_POINT('Ctrl Pts',(-45.8148968663299,-2.0630989642918,-4.70049158783766));
#32009=CARTESIAN_POINT('Ctrl Pts',(-45.6959878673349,0.43320082545685,-5.11501080629941));
#32010=CARTESIAN_POINT('Ctrl Pts',(-45.57707886834,2.82423205533933,-4.2865734335784));
#32011=CARTESIAN_POINT('Ctrl Pts',(-45.458169869345,4.52896994562411,-2.41649120322742));
#32012=CARTESIAN_POINT('Ctrl Pts',(-45.33926087035,5.13316020105655,0.0408026249133683));
#32013=CARTESIAN_POINT('Ctrl Pts',(-45.2203518713551,4.48998353049627,2.48818134382005));
#32014=CARTESIAN_POINT('Ctrl Pts',(-45.1014428723601,2.75573299237594,4.33092763477912));
#32015=CARTESIAN_POINT('Ctrl Pts',(-44.9825338733652,0.351834506810982,
5.12125092005135));
#32016=CARTESIAN_POINT('Ctrl Pts',(-44.8636248743701,-2.13756038013976,
4.66710125446325));
#32017=CARTESIAN_POINT('Ctrl Pts',(-44.7447158753753,-4.10752434901852,
3.07883780599703));
#32018=CARTESIAN_POINT('Ctrl Pts',(-44.6258068763802,-5.07935269991291,
0.742411369974384));
#32019=CARTESIAN_POINT('Ctrl Pts',(-44.5068978773853,-4.81688944547566,
-1.77442232161193));
#32020=CARTESIAN_POINT('Ctrl Pts',(-44.3879888783903,-3.38391360602914,
-3.86006829609525));
#32021=CARTESIAN_POINT('Ctrl Pts',(-44.2690798793954,-1.12864084321015,
-5.00771087473245));
#32022=CARTESIAN_POINT('Ctrl Pts',(-44.1501708804004,1.40089365066207,-4.93847100187184));
#32023=CARTESIAN_POINT('Ctrl Pts',(-44.0312618814055,3.59000847626879,-3.66917388350381));
#32024=CARTESIAN_POINT('Ctrl Pts',(-43.9123528824105,4.90674506105724,-1.50826135214278));
#32025=CARTESIAN_POINT('Ctrl Pts',(-43.7934438834155,5.03113377377479,1.0191618737146));
#32026=CARTESIAN_POINT('Ctrl Pts',(-43.6745348844206,3.93294860418829,3.29892589575286));
#32027=CARTESIAN_POINT('Ctrl Pts',(-43.5556258854256,1.87904914644228,4.77704730235934));
#32028=CARTESIAN_POINT('Ctrl Pts',(-43.4367168864307,-0.631460783603362,
5.09433353275251));
#32029=CARTESIAN_POINT('Ctrl Pts',(-43.3178078874357,-2.98852815585981,
4.1736963834896));
#32030=CARTESIAN_POINT('Ctrl Pts',(-43.1988988884407,-4.61937092551605,
2.23882654156266));
#32031=CARTESIAN_POINT('Ctrl Pts',(-43.0799898894457,-5.12771247664765,
-0.240047840842145));
#32032=CARTESIAN_POINT('Ctrl Pts',(-42.9610808904508,-4.3899829470878,-2.66065848599509));
#32033=CARTESIAN_POINT('Ctrl Pts',(-42.8421718914558,-2.58553566085927,
-4.43458815242399));
#32034=CARTESIAN_POINT('Ctrl Pts',(-42.7232628924609,-0.152687346186725,
-5.13117710407935));
#32035=CARTESIAN_POINT('Ctrl Pts',(-42.6043538934659,2.31704211155937,-4.58033832038339));
#32036=CARTESIAN_POINT('Ctrl Pts',(-42.485444894471,4.22416955122785,-2.91755220346545));
#32037=CARTESIAN_POINT('Ctrl Pts',(-42.366535895476,5.10393188151341,-0.543635036753471));
#32038=CARTESIAN_POINT('Ctrl Pts',(-42.247626896481,4.74519466135189,1.95807585226838));
#32039=CARTESIAN_POINT('Ctrl Pts',(-42.1287178974861,3.22984652054977,3.99255890873504));
#32040=CARTESIAN_POINT('Ctrl Pts',(-42.0098088984911,0.936649650830306,
5.03987138354553));
#32041=CARTESIAN_POINT('Ctrl Pts',(-41.8512635664979,-2.44270025858044,
4.84518225905994));
#32042=CARTESIAN_POINT('Ctrl Pts',(-41.6530819015062,-5.62465355290164,
1.50292499192576));
#32043=CARTESIAN_POINT('Ctrl Pts',(-41.4152639035164,-4.30521954672645,
-3.91925959538388));
#32044=CARTESIAN_POINT('Ctrl Pts',(-41.2170822385247,0.0566412091691752,
-5.42580569594987));
#32045=CARTESIAN_POINT('Ctrl Pts',(-41.0585369065314,3.1476070435387,-4.04600865428477));
#32046=CARTESIAN_POINT('Ctrl Pts',(-40.9396279075364,4.70319485935917,-2.06213319184877));
#32047=CARTESIAN_POINT('Ctrl Pts',(-40.8207189085415,5.11432592288447,0.441139175171419));
#32048=CARTESIAN_POINT('Ctrl Pts',(-40.7018099095466,4.28348608439691,2.82796864711987));
#32049=CARTESIAN_POINT('Ctrl Pts',(-40.5829009105515,2.41133856199462,4.53223626887482));
#32050=CARTESIAN_POINT('Ctrl Pts',(-40.4639919115566,-0.0465612617872453,
5.13283696651402));
#32051=CARTESIAN_POINT('Ctrl Pts',(-40.3450829125616,-2.49325046885601,
4.48731478711524));
#32052=CARTESIAN_POINT('Ctrl Pts',(-40.2261739135667,-4.3340233953047,2.75078315105821));
#32053=CARTESIAN_POINT('Ctrl Pts',(-40.1072649145717,-5.1216471237482,0.346099110980013));
#32054=CARTESIAN_POINT('Ctrl Pts',(-39.9883559155767,-4.66468855239917,
-2.14283431888165));
#32055=CARTESIAN_POINT('Ctrl Pts',(-39.8694469165818,-3.07420903783289,
-4.11098173462434));
#32056=CARTESIAN_POINT('Ctrl Pts',(-39.7505379175868,-0.736688055742687,
-5.08019022758471));
#32057=CARTESIAN_POINT('Ctrl Pts',(-39.6316289185919,1.77984776980155,-4.81488512640624));
#32058=CARTESIAN_POINT('Ctrl Pts',(-39.5127199195969,3.86387829223252,-3.37956375387986));
#32059=CARTESIAN_POINT('Ctrl Pts',(-39.393810920602,5.00897920406026,-1.12299782820232));
#32060=CARTESIAN_POINT('Ctrl Pts',(-39.274901921607,4.93688959696835,1.40645621396351));
#32061=CARTESIAN_POINT('Ctrl Pts',(-39.155992922612,3.66512706095948,3.59414009571131));
#32062=CARTESIAN_POINT('Ctrl Pts',(-39.0370839236171,1.50273227714512,4.90844105091367));
#32063=CARTESIAN_POINT('Ctrl Pts',(-38.9181749246221,-1.024829109976,5.02998252006308));
#32064=CARTESIAN_POINT('Ctrl Pts',(-38.7992659256272,-3.30335521405396,
3.92922927399997));
#32065=CARTESIAN_POINT('Ctrl Pts',(-38.6803569266322,-4.77916021775016,
1.8736665009182));
#32066=CARTESIAN_POINT('Ctrl Pts',(-38.5614479276373,-5.09362090864089,
-0.637200552750805));
#32067=CARTESIAN_POINT('Ctrl Pts',(-38.4425389286422,-4.17032279259777,
-2.99322673680418));
#32068=CARTESIAN_POINT('Ctrl Pts',(-38.3236299296473,-2.23362892764998,
-4.62189358672198));
#32069=CARTESIAN_POINT('Ctrl Pts',(-38.2047209306523,0.24584068126806,-5.12743218946767));
#32070=CARTESIAN_POINT('Ctrl Pts',(-38.0858119316574,2.66557057395082,-4.38699578545469));
#32071=CARTESIAN_POINT('Ctrl Pts',(-37.9669029326624,4.43756214501543,-2.58051171516208));
#32072=CARTESIAN_POINT('Ctrl Pts',(-37.8479939336674,5.13121833701352,-0.146958775709808));
#32073=CARTESIAN_POINT('Ctrl Pts',(-37.7290849346725,4.57797947941461,2.32230540411237));
#32074=CARTESIAN_POINT('Ctrl Pts',(-37.6101759356775,2.91228358433659,4.22724530019794));
#32075=CARTESIAN_POINT('Ctrl Pts',(-37.4912669366826,0.538897673790773,
5.10495717915922));
#32076=CARTESIAN_POINT('Ctrl Pts',(-37.3723579376876,-1.96544131602887,
4.74215551590023));
#32077=CARTESIAN_POINT('Ctrl Pts',(-37.2534489386926,-3.99217462115323,
3.22700175054406));
#32078=CARTESIAN_POINT('Ctrl Pts',(-37.1345399396977,-5.04880249610402,
0.927680903710816));
#32079=CARTESIAN_POINT('Ctrl Pts',(-37.0156309407027,-4.87856251527856,
-1.59706802870025));
#32080=CARTESIAN_POINT('Ctrl Pts',(-36.8967219417078,-3.52282329240276,
-3.73372663089914));
#32081=CARTESIAN_POINT('Ctrl Pts',(-36.7778129427128,-1.31103183489013,
-4.96308311754722));
#32082=CARTESIAN_POINT('Ctrl Pts',(-36.6589039437178,1.21934265639497,-4.98640170765204));
#32083=CARTESIAN_POINT('Ctrl Pts',(-36.5399949447229,3.45341474498895,-3.79801594294593));
#32084=CARTESIAN_POINT('Ctrl Pts',(-36.4210859457279,4.84830099762253,-1.68670564718072));
#32085=CARTESIAN_POINT('Ctrl Pts',(-36.302176946733,5.06504161003687,0.834477077201056));
#32086=CARTESIAN_POINT('Ctrl Pts',(-36.183267947738,4.05096823352596,3.15288040920401));
#32087=CARTESIAN_POINT('Ctrl Pts',(-36.064358948743,2.05250247598596,4.70512827559997));
#32088=CARTESIAN_POINT('Ctrl Pts',(-35.9454499497481,-0.444724980715808,
5.1140217241723));
#32089=CARTESIAN_POINT('Ctrl Pts',(-35.8265409507531,-2.83388348761767,
4.28019893023523));
#32090=CARTESIAN_POINT('Ctrl Pts',(-35.7076319517582,-4.53440333997578,
2.40628029418757));
#32091=CARTESIAN_POINT('Ctrl Pts',(-35.5887229527631,-5.13305523310285,
-0.0523686709243773));
#32092=CARTESIAN_POINT('Ctrl Pts',(-35.4698139537683,-4.48436570768963,
-2.4982919572132));
#32093=CARTESIAN_POINT('Ctrl Pts',(-35.3509049547733,-2.74596745539376,
-4.33712591905021));
#32094=CARTESIAN_POINT('Ctrl Pts',(-35.2319959557783,-0.340294298478209,
-5.12203068071659));
#32095=CARTESIAN_POINT('Ctrl Pts',(-35.1130869567833,2.14807096941398,-4.66227300939571));
#32096=CARTESIAN_POINT('Ctrl Pts',(-34.9941779577884,4.11445122673493,-3.06957482505287));
#32097=CARTESIAN_POINT('Ctrl Pts',(-34.8752689587934,5.08101262440804,-0.730964578064523));
#32098=CARTESIAN_POINT('Ctrl Pts',(-34.7563599597985,4.81287904867072,1.78527134258224));
#32099=CARTESIAN_POINT('Ctrl Pts',(-34.6374509608035,3.37520742839479,3.86768319787021));
#32100=CARTESIAN_POINT('Ctrl Pts',(-34.5185419618086,1.11735448716771,5.01024125704392));
#32101=CARTESIAN_POINT('Ctrl Pts',(-34.3996329628135,-1.41201755286977,
4.93530190912031));
#32102=CARTESIAN_POINT('Ctrl Pts',(-34.2807239638187,-3.59826685266438,
3.66107554699376));
#32103=CARTESIAN_POINT('Ctrl Pts',(-34.1618149648236,-4.91013100044579,
1.49720141004484));
#32104=CARTESIAN_POINT('Ctrl Pts',(-34.0429059658287,-5.02882470895011,
-1.03049529374547));
#32105=CARTESIAN_POINT('Ctrl Pts',(-33.9239969668337,-3.92550519897206,
-3.30777983496817));
#32106=CARTESIAN_POINT('Ctrl Pts',(-33.8050879678388,-1.86828104526512,
-4.78126807862545));
#32107=CARTESIAN_POINT('Ctrl Pts',(-33.6861789688438,0.642938677046443,
-5.0928997988704));
#32108=CARTESIAN_POINT('Ctrl Pts',(-33.5672699698489,2.9979231739338,-4.16694794147646));
#32109=CARTESIAN_POINT('Ctrl Pts',(-33.4483609708539,4.62440708498306,-2.22842043073757));
#32110=CARTESIAN_POINT('Ctrl Pts',(-33.3294519718589,5.12715196901376,0.251617150501759));
#32111=CARTESIAN_POINT('Ctrl Pts',(-33.210542972864,4.38398993802041,2.67051132315832));
#32112=CARTESIAN_POINT('Ctrl Pts',(-33.091633973869,2.57551066811489,4.44046656356744));
#32113=CARTESIAN_POINT('Ctrl Pts',(-32.972724974874,0.141177791647324,5.13138064609063));
#32114=CARTESIAN_POINT('Ctrl Pts',(-32.8538159758791,-2.32746153560409,
4.57536023758993));
#32115=CARTESIAN_POINT('Ctrl Pts',(-32.7349069768842,-4.23052363034337,
2.90751927207641));
#32116=CARTESIAN_POINT('Ctrl Pts',(-32.6159979778891,-5.1055610677782,0.533146027081844));
#32117=CARTESIAN_POINT('Ctrl Pts',(-32.4970889788942,-4.73993821730678,
-1.97078263646032));
#32118=CARTESIAN_POINT('Ctrl Pts',(-32.3781799798992,-3.22250207162541,
-3.99580766607272));
#32119=CARTESIAN_POINT('Ctrl Pts',(-32.2592709809043,-0.921992275415497,
-5.04984442724594));
#32120=CARTESIAN_POINT('Ctrl Pts',(-32.1403619819093,1.60256326187619,-4.87676014550612));
#32121=CARTESIAN_POINT('Ctrl Pts',(-32.0214529829143,3.73769311337828,-3.51861459283342));
#32122=CARTESIAN_POINT('Ctrl Pts',(-31.9025439839194,4.96455699567959,-1.30543954265259));
#32123=CARTESIAN_POINT('Ctrl Pts',(-31.7836349849244,4.98502480941995,1.22495963592593));
#32124=CARTESIAN_POINT('Ctrl Pts',(-31.6647259859295,3.79412289105023,3.45769141320538));
#32125=CARTESIAN_POINT('Ctrl Pts',(-31.5458169869345,1.68124239217829,4.85019824183698));
#32126=CARTESIAN_POINT('Ctrl Pts',(-31.4269079879396,-0.840182819327128,
5.06409814678598));
#32127=CARTESIAN_POINT('Ctrl Pts',(-31.3079989889446,-3.15744240337648,
4.04741382447126));
#32128=CARTESIAN_POINT('Ctrl Pts',(-31.1890899899496,-4.70743740996291,
2.04719985417626));
#32129=CARTESIAN_POINT('Ctrl Pts',(-31.0701809909546,-5.11351795109797,
-0.450485284301895));
#32130=CARTESIAN_POINT('Ctrl Pts',(-30.9512719919597,-4.27700252027738,
-2.83870566914707));
#32131=CARTESIAN_POINT('Ctrl Pts',(-30.8323629929647,-2.40117226505815,
-4.53710769903983));
#32132=CARTESIAN_POINT('Ctrl Pts',(-30.7134539939698,0.0581556084619265,
-5.13300037307933));
#32133=CARTESIAN_POINT('Ctrl Pts',(-30.5945449949748,2.5033345078755,-4.48153349680761));
#32134=CARTESIAN_POINT('Ctrl Pts',(-30.4756359959799,4.34023277605901,-2.7411089157019));
#32135=CARTESIAN_POINT('Ctrl Pts',(-30.3567269969849,5.12237892249915,-0.334464657353477));
#32136=CARTESIAN_POINT('Ctrl Pts',(-30.2378179979899,4.65991389359687,2.15320333710529));
#32137=CARTESIAN_POINT('Ctrl Pts',(-30.118908998995,3.06480657161386,4.11815974006944));
#32138=CARTESIAN_POINT('Ctrl Pts',(-30.0396363329983,1.50529535683796,4.76007633060596));
#32139=CARTESIAN_POINT('Ctrl Pts',(-30.,0.695807839646249,4.87560011181053));
#32140=CARTESIAN_POINT('Ctrl Pts',(-52.9038972033484,2.69291261530793,-3.77880514723369));
#32141=CARTESIAN_POINT('Ctrl Pts',(-52.86426087035,3.32030114727052,-3.33170548832209));
#32142=CARTESIAN_POINT('Ctrl Pts',(-52.7849882043534,4.34745254164389,-2.11942289497076));
#32143=CARTESIAN_POINT('Ctrl Pts',(-52.6660792053584,4.83164862445098,0.215420879815001));
#32144=CARTESIAN_POINT('Ctrl Pts',(-52.5471702063635,4.14174081950731,2.49736228942754));
#32145=CARTESIAN_POINT('Ctrl Pts',(-52.4282612073685,2.4453874570205,4.17270978867922));
#32146=CARTESIAN_POINT('Ctrl Pts',(-52.3093522083736,0.154798082552608,
4.83394713716095));
#32147=CARTESIAN_POINT('Ctrl Pts',(-52.1904432093786,-2.17340619191372,
4.32059413942983));
#32148=CARTESIAN_POINT('Ctrl Pts',(-52.0715342103836,-3.97346960773852,
2.75729547911));
#32149=CARTESIAN_POINT('Ctrl Pts',(-51.9526252113887,-4.80797261588486,
0.523986080040587));
#32150=CARTESIAN_POINT('Ctrl Pts',(-51.8337162123937,-4.47413001592062,
-1.83666132209573));
#32151=CARTESIAN_POINT('Ctrl Pts',(-51.7148072133987,-3.05306589759289,
-3.75099256041035));
#32152=CARTESIAN_POINT('Ctrl Pts',(-51.5958982144038,-0.890101456284074,
-4.75382815861975));
#32153=CARTESIAN_POINT('Ctrl Pts',(-51.4769892154088,1.48915921974122,-4.60147411633167));
#32154=CARTESIAN_POINT('Ctrl Pts',(-51.3580802164139,3.50655158487809,-3.33095433270087));
#32155=CARTESIAN_POINT('Ctrl Pts',(-51.2391712174189,4.67184577403192,-1.25100654027042));
#32156=CARTESIAN_POINT('Ctrl Pts',(-51.1202622184239,4.70187324896995,1.1329378999895));
#32157=CARTESIAN_POINT('Ctrl Pts',(-51.001353219429,3.58933728456801,3.24157651203533));
#32158=CARTESIAN_POINT('Ctrl Pts',(-50.882444220434,1.60458606819627,4.56250631633484));
#32159=CARTESIAN_POINT('Ctrl Pts',(-50.763535221439,-0.770082374836318,
4.77473910577498));
#32160=CARTESIAN_POINT('Ctrl Pts',(-50.6446262224441,-2.95761945119629,
3.826701915188));
#32161=CARTESIAN_POINT('Ctrl Pts',(-50.5257172234491,-4.4264498169038,1.94876945624846));
#32162=CARTESIAN_POINT('Ctrl Pts',(-50.4068082244542,-4.81964511874225,
-0.402717398365085));
#32163=CARTESIAN_POINT('Ctrl Pts',(-50.2878992254592,-4.04165820913488,
-2.65634321825318));
#32164=CARTESIAN_POINT('Ctrl Pts',(-50.1689902264643,-2.28154127075387,
-4.26447298076822));
#32165=CARTESIAN_POINT('Ctrl Pts',(-50.0500812274693,0.0329941953675342,
-4.83632833418913));
#32166=CARTESIAN_POINT('Ctrl Pts',(-49.9311722284743,2.33951201418187,-4.23294742572411));
#32167=CARTESIAN_POINT('Ctrl Pts',(-49.8122632294794,4.07752431300185,-2.600952873497));
#32168=CARTESIAN_POINT('Ctrl Pts',(-49.6933542304844,4.82469105693362,-0.336922214257224));
#32169=CARTESIAN_POINT('Ctrl Pts',(-49.5744452314894,4.39944941761592,2.00898113359999));
#32170=CARTESIAN_POINT('Ctrl Pts',(-49.4555362324945,2.90513385873921,3.86669854476821));
#32171=CARTESIAN_POINT('Ctrl Pts',(-49.3366272334995,0.7048656802531,4.78480143225605));
#32172=CARTESIAN_POINT('Ctrl Pts',(-49.2177182345045,-1.66668609397878,
4.54018918520461));
#32173=CARTESIAN_POINT('Ctrl Pts',(-49.0988092355096,-3.63323022611126,
3.19230300839155));
#32174=CARTESIAN_POINT('Ctrl Pts',(-48.9799002365146,-4.71689304520134,
1.06868160527093));
#32175=CARTESIAN_POINT('Ctrl Pts',(-48.8609912375197,-4.65434258683413,
-1.31463130104814));
#32176=CARTESIAN_POINT('Ctrl Pts',(-48.7420822385247,-3.46077872202735,
-3.3784864970096));
#32177=CARTESIAN_POINT('Ctrl Pts',(-48.6231732395298,-1.4262395619327,-4.6213635525991));
#32178=CARTESIAN_POINT('Ctrl Pts',(-48.5042642405347,0.954878311534569,
-4.74124116487174));
#32179=CARTESIAN_POINT('Ctrl Pts',(-48.3853552415398,3.10395908164831,-3.7089888639313));
#32180=CARTESIAN_POINT('Ctrl Pts',(-48.2664462425448,4.4987723544973,-1.77544576817321));
#32181=CARTESIAN_POINT('Ctrl Pts',(-48.1475372435499,4.80037606003829,0.589533761140604));
#32182=CARTESIAN_POINT('Ctrl Pts',(-48.0286282445549,3.93547996919283,2.81125555319956));
#32183=CARTESIAN_POINT('Ctrl Pts',(-47.90971924556,2.11425534797181,4.34983731843916));
#32184=CARTESIAN_POINT('Ctrl Pts',(-47.790810246565,-0.220737028540126,
4.83140099117685));
#32185=CARTESIAN_POINT('Ctrl Pts',(-47.6719012475701,-2.50208992022283,
4.13892575488286));
#32186=CARTESIAN_POINT('Ctrl Pts',(-47.5529922485751,-4.17543057578559,
2.44068430570367));
#32187=CARTESIAN_POINT('Ctrl Pts',(-47.4340832495801,-4.83413428300043,
0.149352292360577));
#32188=CARTESIAN_POINT('Ctrl Pts',(-47.3151742505852,-4.31813488647971,
-2.17827258980143));
#32189=CARTESIAN_POINT('Ctrl Pts',(-47.1962652515901,-2.75282114398926,
-3.97657341470254));
#32190=CARTESIAN_POINT('Ctrl Pts',(-47.0773562525953,-0.51856703853771,
-4.80855992994323));
#32191=CARTESIAN_POINT('Ctrl Pts',(-46.9584472536002,1.84169976619019,-4.47205795406638));
#32192=CARTESIAN_POINT('Ctrl Pts',(-46.8395382546054,3.75443029971838,-3.04883805700957));
#32193=CARTESIAN_POINT('Ctrl Pts',(-46.7206292556103,4.75482768988579,-0.884745168287887));
#32194=CARTESIAN_POINT('Ctrl Pts',(-46.6017202566154,4.5997936174481,1.49434234705342));
#32195=CARTESIAN_POINT('Ctrl Pts',(-46.4828112576204,3.32700163374164,3.5103020528715));
#32196=CARTESIAN_POINT('Ctrl Pts',(-46.3639022586255,1.24574242167685,4.67325220720515));
#32197=CARTESIAN_POINT('Ctrl Pts',(-46.2449932596305,-1.13823438231442,
4.70059388420562));
#32198=CARTESIAN_POINT('Ctrl Pts',(-46.1260842606356,-3.24561823637756,
3.58568300843865));
#32199=CARTESIAN_POINT('Ctrl Pts',(-46.0071752616406,-4.56431117028574,
1.59944487686198));
#32200=CARTESIAN_POINT('Ctrl Pts',(-45.8882662626456,-4.77386848977654,
-0.775461163199525));
#32201=CARTESIAN_POINT('Ctrl Pts',(-45.7693572636507,-3.82336739891617,
-2.96192878142196));
#32202=CARTESIAN_POINT('Ctrl Pts',(-45.6504482646557,-1.94378132875964,
-4.42864251428049));
#32203=CARTESIAN_POINT('Ctrl Pts',(-45.5315392656608,0.408147011219782,
-4.81918835391478));
#32204=CARTESIAN_POINT('Ctrl Pts',(-45.4126302666657,2.66089491210501,-4.03866297679377));
#32205=CARTESIAN_POINT('Ctrl Pts',(-45.2937212676709,4.26704068548633,-2.27673541756528));
#32206=CARTESIAN_POINT('Ctrl Pts',(-45.1748122686758,4.83628809332033,0.0384428385859125));
#32207=CARTESIAN_POINT('Ctrl Pts',(-45.0559032696809,4.23030901768346,2.34427941770878));
#32208=CARTESIAN_POINT('Ctrl Pts',(-44.936994270686,2.59635743623479,4.08045198916703));
#32209=CARTESIAN_POINT('Ctrl Pts',(-44.818085271691,0.331486446840065,4.82506757580879));
#32210=CARTESIAN_POINT('Ctrl Pts',(-44.699176272696,-2.01393632972831,4.39718328343523));
#32211=CARTESIAN_POINT('Ctrl Pts',(-44.5802672737011,-3.86996904910406,
2.9007757481138));
#32212=CARTESIAN_POINT('Ctrl Pts',(-44.4613582747061,-4.78559250484858,
0.699474617646573));
#32213=CARTESIAN_POINT('Ctrl Pts',(-44.3424492757111,-4.53830859734306,
-1.67180006280874));
#32214=CARTESIAN_POINT('Ctrl Pts',(-44.2235402767162,-3.18820773960938,
-3.63682441392853));
#32215=CARTESIAN_POINT('Ctrl Pts',(-44.1046312777212,-1.06336682625425,
-4.71809402583507));
#32216=CARTESIAN_POINT('Ctrl Pts',(-43.9857222787263,1.31987411600958,-4.65285858420012));
#32217=CARTESIAN_POINT('Ctrl Pts',(-43.8668132797312,3.38238328215905,-3.45697022303314));
#32218=CARTESIAN_POINT('Ctrl Pts',(-43.7479042807364,4.62296748713688,-1.42103229458567));
#32219=CARTESIAN_POINT('Ctrl Pts',(-43.6289952817413,4.74016228073313,0.960219483116374));
#32220=CARTESIAN_POINT('Ctrl Pts',(-43.5100862827464,3.7054897492117,3.10813522381238));
#32221=CARTESIAN_POINT('Ctrl Pts',(-43.3911772837514,1.77037588108625,4.50077069187773));
#32222=CARTESIAN_POINT('Ctrl Pts',(-43.2722682847565,-0.594940767387539,
4.79970693351479));
#32223=CARTESIAN_POINT('Ctrl Pts',(-43.1533592857615,-2.81568908248032,
3.9323140782651));
#32224=CARTESIAN_POINT('Ctrl Pts',(-43.0344502867666,-4.35221339889315,
2.10934584580864));
#32225=CARTESIAN_POINT('Ctrl Pts',(-42.9155412877716,-4.83115543358196,
-0.226164870960634));
#32226=CARTESIAN_POINT('Ctrl Pts',(-42.7966322887766,-4.13609188595165,
-2.50678148590829));
#32227=CARTESIAN_POINT('Ctrl Pts',(-42.6777232897817,-2.43600332771514,
-4.17811738584219));
#32228=CARTESIAN_POINT('Ctrl Pts',(-42.5588142907867,-0.143856798821795,
-4.83441968712938));
#32229=CARTESIAN_POINT('Ctrl Pts',(-42.4399052917917,2.18303788250169,-4.31543821244649));
#32230=CARTESIAN_POINT('Ctrl Pts',(-42.3209962927968,3.97986817176768,-2.74881796604673));
#32231=CARTESIAN_POINT('Ctrl Pts',(-42.2020872938018,4.80875016965195,-0.512194350533092));
#32232=CARTESIAN_POINT('Ctrl Pts',(-42.0831782948068,4.47076022222327,1.84483214223366));
#32233=CARTESIAN_POINT('Ctrl Pts',(-41.9642692958119,3.04305099758463,3.7616525407138));
#32234=CARTESIAN_POINT('Ctrl Pts',(-41.8453602968169,0.882479286929472,
4.74839455801324));
#32235=CARTESIAN_POINT('Ctrl Pts',(-41.6868149648237,-2.30142869371028,
4.564965119272));
#32236=CARTESIAN_POINT('Ctrl Pts',(-41.488633299832,-5.29935633050202,1.41600455838255));
#32237=CARTESIAN_POINT('Ctrl Pts',(-41.2508153018422,-4.0562307072897,-3.69259243299773));
#32238=CARTESIAN_POINT('Ctrl Pts',(-41.0526336368505,0.0533654113191093,
-5.11200867617396));
#32239=CARTESIAN_POINT('Ctrl Pts',(-40.8940883048573,2.96556777323727,-3.81201106409278));
#32240=CARTESIAN_POINT('Ctrl Pts',(-40.7751793058623,4.43118944431198,-1.9428714109733));
#32241=CARTESIAN_POINT('Ctrl Pts',(-40.6562703068673,4.8185430801701,0.415626252993168));
#32242=CARTESIAN_POINT('Ctrl Pts',(-40.5373613078723,4.03575418191859,2.66441540116632));
#32243=CARTESIAN_POINT('Ctrl Pts',(-40.4184523088774,2.27188077510969,4.27011810361233));
#32244=CARTESIAN_POINT('Ctrl Pts',(-40.2995433098825,-0.0438684294219718,
4.83598355278229));
#32245=CARTESIAN_POINT('Ctrl Pts',(-40.1806343108874,-2.34905537405823,
4.22779461888579));
#32246=CARTESIAN_POINT('Ctrl Pts',(-40.0617253118925,-4.08336870892313,
2.59169386492762));
#32247=CARTESIAN_POINT('Ctrl Pts',(-39.9428163128975,-4.82544086538998,
0.326082752920268));
#32248=CARTESIAN_POINT('Ctrl Pts',(-39.8239073139026,-4.39491011801506,
-2.01890525455108));
#32249=CARTESIAN_POINT('Ctrl Pts',(-39.7049983149076,-2.89641468095787,
-3.87322647965064));
#32250=CARTESIAN_POINT('Ctrl Pts',(-39.5860893159127,-0.694082306596669,
-4.78638159479478));
#32251=CARTESIAN_POINT('Ctrl Pts',(-39.4671803169177,1.67691173465467,-4.5364201964222));
#32252=CARTESIAN_POINT('Ctrl Pts',(-39.3482713179228,3.64041406206585,-3.18410945758946));
#32253=CARTESIAN_POINT('Ctrl Pts',(-39.2293623189277,4.71928900237705,-1.05805017038851));
#32254=CARTESIAN_POINT('Ctrl Pts',(-39.1104533199328,4.65136863855145,1.32511497302736));
#32255=CARTESIAN_POINT('Ctrl Pts',(-38.9915443209378,3.45315744514966,3.38627595278169));
#32256=CARTESIAN_POINT('Ctrl Pts',(-38.8726353219429,1.41582298910311,4.62456539081176));
#32257=CARTESIAN_POINT('Ctrl Pts',(-38.7537263229479,-0.965558959419366,
4.73907760883507));
#32258=CARTESIAN_POINT('Ctrl Pts',(-38.634817323953,-3.11230837612443,3.70198552343258));
#32259=CARTESIAN_POINT('Ctrl Pts',(-38.5159083249579,-4.50276140854086,
1.76530453644884));
#32260=CARTESIAN_POINT('Ctrl Pts',(-38.3969993259631,-4.79903552343387,
-0.600348581696643));
#32261=CARTESIAN_POINT('Ctrl Pts',(-38.278090326968,-3.92913559623399,-2.82011592485163));
#32262=CARTESIAN_POINT('Ctrl Pts',(-38.1591813279731,-2.10444883163121,
-4.35459016405844));
#32263=CARTESIAN_POINT('Ctrl Pts',(-38.0402723289782,0.231622687214369,
-4.83089135658103));
#32264=CARTESIAN_POINT('Ctrl Pts',(-37.9213633299832,2.51140948728817,-4.1332774843602));
#32265=CARTESIAN_POINT('Ctrl Pts',(-37.8024543309883,4.18091938001268,-2.43126993779448));
#32266=CARTESIAN_POINT('Ctrl Pts',(-37.6835453319933,4.83445853539064,-0.138459535517298));
#32267=CARTESIAN_POINT('Ctrl Pts',(-37.5646363329983,4.31321579310937,2.18799677684917));
#32268=CARTESIAN_POINT('Ctrl Pts',(-37.4457273340034,2.74385405318153,3.98276603732017));
#32269=CARTESIAN_POINT('Ctrl Pts',(-37.3268183350084,0.507730969069655,
4.80971617004981));
#32270=CARTESIAN_POINT('Ctrl Pts',(-37.2079093360135,-1.85177163044197,
4.46789684325476));
#32271=CARTESIAN_POINT('Ctrl Pts',(-37.0890003370184,-3.76129047808892,
3.04037075251765));
#32272=CARTESIAN_POINT('Ctrl Pts',(-36.9700913380235,-4.75680914700616,
0.874029239939502));
#32273=CARTESIAN_POINT('Ctrl Pts',(-36.8511823390286,-4.59641485576549,
-1.50470290988306));
#32274=CARTESIAN_POINT('Ctrl Pts',(-36.7322733400336,-3.31908369826683,
-3.51778961525764));
#32275=CARTESIAN_POINT('Ctrl Pts',(-36.6133643410386,-1.2352093846083,-4.67604727836319));
#32276=CARTESIAN_POINT('Ctrl Pts',(-36.4944553420437,1.14882297450738,-4.69801725694553));
#32277=CARTESIAN_POINT('Ctrl Pts',(-36.3755463430487,3.25368933723309,-3.57836080770076));
#32278=CARTESIAN_POINT('Ctrl Pts',(-36.2566373440537,4.56790348814921,-1.58915641025914));
#32279=CARTESIAN_POINT('Ctrl Pts',(-36.1377283450588,4.77210908511122,0.786215780248905));
#32280=CARTESIAN_POINT('Ctrl Pts',(-36.0188193460638,3.81668381013861,2.97053615812688));
#32281=CARTESIAN_POINT('Ctrl Pts',(-35.8999103470689,1.93379767965904,4.43301104301114));
#32282=CARTESIAN_POINT('Ctrl Pts',(-35.7810013480739,-0.419004676416563,
4.8182564745408));
#32283=CARTESIAN_POINT('Ctrl Pts',(-35.6620923490789,-2.66998816171791,
4.03265713762026));
#32284=CARTESIAN_POINT('Ctrl Pts',(-35.543183350084,-4.27215984393455,2.26711504807025));
#32285=CARTESIAN_POINT('Ctrl Pts',(-35.424274351089,-4.83618919610208,-0.049339971817471));
#32286=CARTESIAN_POINT('Ctrl Pts',(-35.3053653520941,-4.22501609704862,
-2.35380529207354));
#32287=CARTESIAN_POINT('Ctrl Pts',(-35.1864563530991,-2.58715668106996,
-4.08629180075389));
#32288=CARTESIAN_POINT('Ctrl Pts',(-35.0675473541041,-0.32061365698583,
-4.82580223965586));
#32289=CARTESIAN_POINT('Ctrl Pts',(-34.9486383551092,2.0238390476973,-4.39263427595891));
#32290=CARTESIAN_POINT('Ctrl Pts',(-34.8297293561142,3.87649531653223,-2.89204848407095));
#32291=CARTESIAN_POINT('Ctrl Pts',(-34.7108203571192,4.78715642897274,-0.688689841553088));
#32292=CARTESIAN_POINT('Ctrl Pts',(-34.5919113581243,4.53453013854623,1.6820216395544));
#32293=CARTESIAN_POINT('Ctrl Pts',(-34.4730023591293,3.18000507661384,3.64399891410845));
#32294=CARTESIAN_POINT('Ctrl Pts',(-34.3540933601343,1.05273320735146,4.7204780655621));
#32295=CARTESIAN_POINT('Ctrl Pts',(-34.2351843611394,-1.33035467646186,
4.64987277332718));
#32296=CARTESIAN_POINT('Ctrl Pts',(-34.1162753621445,-3.39016404213297,
3.4493402471693));
#32297=CARTESIAN_POINT('Ctrl Pts',(-33.9973663631495,-4.62615760349954,
1.4106119951627));
#32298=CARTESIAN_POINT('Ctrl Pts',(-33.8784573641545,-4.73798675877766,
-0.970897444100449));
#32299=CARTESIAN_POINT('Ctrl Pts',(-33.7595483651595,-3.69847682722778,
-3.11647710271909));
#32300=CARTESIAN_POINT('Ctrl Pts',(-33.6406393661646,-1.76023054420391,
-4.50474736301224));
#32301=CARTESIAN_POINT('Ctrl Pts',(-33.5217303671696,0.605754846282592,
-4.79835611845518));
#32302=CARTESIAN_POINT('Ctrl Pts',(-33.4028213681747,2.82454074739396,-3.92595592685773));
#32303=CARTESIAN_POINT('Ctrl Pts',(-33.2839123691797,4.35695829621027,-2.09954156386342));
#32304=CARTESIAN_POINT('Ctrl Pts',(-33.1650033701848,4.83062734244711,0.237065079090355));
#32305=CARTESIAN_POINT('Ctrl Pts',(-33.0460943711897,4.13044547764555,2.51606449231984));
#32306=CARTESIAN_POINT('Ctrl Pts',(-32.9271853721949,2.42655812219919,4.18365582390123));
#32307=CARTESIAN_POINT('Ctrl Pts',(-32.8082763731998,0.133012889923945,
4.83461145745548));
#32308=CARTESIAN_POINT('Ctrl Pts',(-32.6893673742049,-2.19285470770741,
4.31074803298615));
#32309=CARTESIAN_POINT('Ctrl Pts',(-32.5704583752099,-3.98585476793198,
2.73936528101113));
#32310=CARTESIAN_POINT('Ctrl Pts',(-32.451549376215,-4.81028513326609,0.502311964128084));
#32311=CARTESIAN_POINT('Ctrl Pts',(-32.33264037722,-4.46580778030585,-1.85680403998959));
#32312=CARTESIAN_POINT('Ctrl Pts',(-32.2137313782251,-3.03613130883664,
-3.76471340883693));
#32313=CARTESIAN_POINT('Ctrl Pts',(-32.0948223792301,-0.868669608793307,
-4.75779081891554));
#32314=CARTESIAN_POINT('Ctrl Pts',(-31.9759133802352,1.50988033075788,-4.59471672456974));
#32315=CARTESIAN_POINT('Ctrl Pts',(-31.8570043812401,3.52152669947767,-3.31511840538324));
#32316=CARTESIAN_POINT('Ctrl Pts',(-31.7380953822452,4.6774359159633,-1.22994051800305));
#32317=CARTESIAN_POINT('Ctrl Pts',(-31.6191863832502,4.69671999049274,1.1541151006367));
#32318=CARTESIAN_POINT('Ctrl Pts',(-31.5002773842553,3.57469290726663,3.25771866785284));
#32319=CARTESIAN_POINT('Ctrl Pts',(-31.3813683852603,1.5840091181264,4.56969100680148));
#32320=CARTESIAN_POINT('Ctrl Pts',(-31.2624593862654,-0.791591535461496,
4.77122018628319));
#32321=CARTESIAN_POINT('Ctrl Pts',(-31.1435503872704,-2.97483431311015,
3.81333496741468));
#32322=CARTESIAN_POINT('Ctrl Pts',(-31.0246413882754,-4.43518663048317,
1.92880173063014));
#32323=CARTESIAN_POINT('Ctrl Pts',(-30.9057323892805,-4.81778183676882,
-0.424431837571901));
#32324=CARTESIAN_POINT('Ctrl Pts',(-30.7868233902855,-4.02964558940921,
-2.67453145633584));
#32325=CARTESIAN_POINT('Ctrl Pts',(-30.6679143912906,-2.26230243761365,
-4.27470779861144));
#32326=CARTESIAN_POINT('Ctrl Pts',(-30.5490053922956,0.0547922265715433,
-4.836137508863));
#32327=CARTESIAN_POINT('Ctrl Pts',(-30.4300963933006,2.35855621095642,-4.22234768475872));
#32328=CARTESIAN_POINT('Ctrl Pts',(-30.3111873943057,4.0892189752372,-2.58257913103404));
#32329=CARTESIAN_POINT('Ctrl Pts',(-30.1922783953107,4.8261303411607,-0.31512116837149));
#32330=CARTESIAN_POINT('Ctrl Pts',(-30.0733693963157,4.39041159768631,2.02867458911503));
#32331=CARTESIAN_POINT('Ctrl Pts',(-29.9544603973208,2.88755599865654,3.8799893510414));
#32332=CARTESIAN_POINT('Ctrl Pts',(-29.8751877313241,1.41823783518528,4.48478122234858));
#32333=CARTESIAN_POINT('Ctrl Pts',(-29.8355513983258,0.655566364250106,
4.59362378047096));
#32334=CARTESIAN_POINT('Ctrl Pts',(-52.7394486016742,2.52761008811563,-3.54684587865057));
#32335=CARTESIAN_POINT('Ctrl Pts',(-52.6998122686759,3.1164868208927,-3.1271911145732));
#32336=CARTESIAN_POINT('Ctrl Pts',(-52.6205396026793,4.08058725685996,-1.98932362671511));
#32337=CARTESIAN_POINT('Ctrl Pts',(-52.5016306036842,4.53506130721429,0.202197422194829));
#32338=CARTESIAN_POINT('Ctrl Pts',(-52.3827216046893,3.88750300259921,2.34406348002302));
#32339=CARTESIAN_POINT('Ctrl Pts',(-52.2638126056943,2.29527908576773,3.9165709636064));
#32340=CARTESIAN_POINT('Ctrl Pts',(-52.1449036066994,0.145295912261199,
4.53721872735497));
#32341=CARTESIAN_POINT('Ctrl Pts',(-52.0259946077044,-2.03999319733809,
4.05537753857908));
#32342=CARTESIAN_POINT('Ctrl Pts',(-51.9070856087095,-3.72956099958419,
2.58804085557638));
#32343=CARTESIAN_POINT('Ctrl Pts',(-51.7881766097145,-4.51283863360882,
0.491821566884094));
#32344=CARTESIAN_POINT('Ctrl Pts',(-51.6692676107196,-4.19948872440061,
-1.72391917204864));
#32345=CARTESIAN_POINT('Ctrl Pts',(-51.5503586117245,-2.86565561710775,
-3.52074054770459));
#32346=CARTESIAN_POINT('Ctrl Pts',(-51.4314496127296,-0.835463210934045,
-4.46201779537558));
#32347=CARTESIAN_POINT('Ctrl Pts',(-51.3125406137346,1.39774823929737,-4.31901589770407));
#32348=CARTESIAN_POINT('Ctrl Pts',(-51.1936316147397,3.29130440774522,-3.12648606810599));
#32349=CARTESIAN_POINT('Ctrl Pts',(-51.0747226157447,4.38506784120549,-1.17421439281441));
#32350=CARTESIAN_POINT('Ctrl Pts',(-50.9558136167497,4.41325210093325,1.06339331211258));
#32351=CARTESIAN_POINT('Ctrl Pts',(-50.8369046177548,3.36900836609068,3.04259464144634));
#32352=CARTESIAN_POINT('Ctrl Pts',(-50.7179956187598,1.50608969268721,4.28244010841788));
#32353=CARTESIAN_POINT('Ctrl Pts',(-50.5990866197649,-0.722811415510337,
4.48164513889988));
#32354=CARTESIAN_POINT('Ctrl Pts',(-50.4801776207699,-2.77606808299493,
3.59180253754148));
#32355=CARTESIAN_POINT('Ctrl Pts',(-50.361268621775,-4.15473534051688,1.82914562805518));
#32356=CARTESIAN_POINT('Ctrl Pts',(-50.24235962278,-4.52379462817329,-0.377996877054597));
#32357=CARTESIAN_POINT('Ctrl Pts',(-50.123450623785,-3.79356389214153,-2.49328547751131));
#32358=CARTESIAN_POINT('Ctrl Pts',(-50.0045416247901,-2.14149048120899,
-4.00270133735984));
#32359=CARTESIAN_POINT('Ctrl Pts',(-49.8856326257951,0.0309688701320005,
-4.53945375629576));
#32360=CARTESIAN_POINT('Ctrl Pts',(-49.7667236268001,2.19590273174818,-3.97311095610869));
#32361=CARTESIAN_POINT('Ctrl Pts',(-49.6478146278052,3.82722838071063,-2.44129522970522));
#32362=CARTESIAN_POINT('Ctrl Pts',(-49.5289056288102,4.52853082503464,-0.316240483566295));
#32363=CARTESIAN_POINT('Ctrl Pts',(-49.4099966298152,4.12939234155163,1.88566125438151));
#32364=CARTESIAN_POINT('Ctrl Pts',(-49.2910876308203,2.7268042813323,3.62934400243824));
#32365=CARTESIAN_POINT('Ctrl Pts',(-49.1721786318253,0.661598001378305,
4.49108979662063));
#32366=CARTESIAN_POINT('Ctrl Pts',(-49.0532696328304,-1.56437775251801,
4.26149289852256));
#32367=CARTESIAN_POINT('Ctrl Pts',(-48.9343606338354,-3.41020697060952,
2.99634575680785));
#32368=CARTESIAN_POINT('Ctrl Pts',(-48.8154516348404,-4.42734991764669,
1.00308134438201));
#32369=CARTESIAN_POINT('Ctrl Pts',(-48.6965426358456,-4.36863907471532,
-1.23393359286629));
#32370=CARTESIAN_POINT('Ctrl Pts',(-48.5776336368505,-3.24834127955239,
-3.17110050428704));
#32371=CARTESIAN_POINT('Ctrl Pts',(-48.4587246378556,-1.33869085997,-4.33768443506052));
#32372=CARTESIAN_POINT('Ctrl Pts',(-48.3398156388605,0.896263784958227,
-4.45020344529392));
#32373=CARTESIAN_POINT('Ctrl Pts',(-48.2209066398657,2.91342475922682,-3.48131521828427));
#32374=CARTESIAN_POINT('Ctrl Pts',(-48.1019976408706,4.22261841053568,-1.66646129140123));
#32375=CARTESIAN_POINT('Ctrl Pts',(-47.9830886418758,4.50570838694445,0.5533456501608));
#32376=CARTESIAN_POINT('Ctrl Pts',(-47.8641796428807,3.69390332800355,2.63868862886432));
#32377=CARTESIAN_POINT('Ctrl Pts',(-47.7452706438858,1.98447328591641,4.08282564582639));
#32378=CARTESIAN_POINT('Ctrl Pts',(-47.6263616448909,-0.207187242908341,
4.53482887473271));
#32379=CARTESIAN_POINT('Ctrl Pts',(-47.5074526458958,-2.3485009085616,3.88486073871624));
#32380=CARTESIAN_POINT('Ctrl Pts',(-47.3885436469009,-3.91912473712975,
2.29086463405221));
#32381=CARTESIAN_POINT('Ctrl Pts',(-47.269634647906,-4.53739438538009,0.140184408030102));
#32382=CARTESIAN_POINT('Ctrl Pts',(-47.150725648911,-4.05306924512365,-2.04456087484974));
#32383=CARTESIAN_POINT('Ctrl Pts',(-47.031816649916,-2.58384117433738,-3.73247428156342));
#32384=CARTESIAN_POINT('Ctrl Pts',(-46.9129076509211,-0.486735169392868,
-4.51338989581109));
#32385=CARTESIAN_POINT('Ctrl Pts',(-46.7939986519261,1.72864833483289,-4.19754385459079));
#32386=CARTESIAN_POINT('Ctrl Pts',(-46.6750896529311,3.52396726382821,-2.86168729951416));
#32387=CARTESIAN_POINT('Ctrl Pts',(-46.5561806539362,4.46295597112516,-0.830435714870097));
#32388=CARTESIAN_POINT('Ctrl Pts',(-46.4372716549412,4.31743855505023,1.40261320402286));
#32389=CARTESIAN_POINT('Ctrl Pts',(-46.3183626559463,3.12277600276341,3.2948246559261));
#32390=CARTESIAN_POINT('Ctrl Pts',(-46.1994536569513,1.1692734083998,4.38638794147786));
#32391=CARTESIAN_POINT('Ctrl Pts',(-46.0805446579563,-1.06836467363388,
4.41205126906581));
#32392=CARTESIAN_POINT('Ctrl Pts',(-45.9616356589614,-3.04638826741205,
3.36557840510464));
#32393=CARTESIAN_POINT('Ctrl Pts',(-45.8427266599664,-4.2841341726916,1.50126408972942));
#32394=CARTESIAN_POINT('Ctrl Pts',(-45.7238176609715,-4.48082796504582,
-0.727860030772266));
#32395=CARTESIAN_POINT('Ctrl Pts',(-45.6049086619765,-3.58867270818134,
-2.78011288804709));
#32396=CARTESIAN_POINT('Ctrl Pts',(-45.4859996629815,-1.82446369322749,
-4.15679344072332));
#32397=CARTESIAN_POINT('Ctrl Pts',(-45.3670906639866,0.383093196982726,
-4.52336590153015));
#32398=CARTESIAN_POINT('Ctrl Pts',(-45.2481816649916,2.49755776887068,-3.79075252000914));
#32399=CARTESIAN_POINT('Ctrl Pts',(-45.1292726659966,4.00511142534855,-2.13697963190314));
#32400=CARTESIAN_POINT('Ctrl Pts',(-45.0103636670017,4.53941598558409,0.0360830522584563));
#32401=CARTESIAN_POINT('Ctrl Pts',(-44.8914546680067,3.97063450487066,2.20037749159751));
#32402=CARTESIAN_POINT('Ctrl Pts',(-44.7725456690117,2.43698188009364,3.82997634355494));
#32403=CARTESIAN_POINT('Ctrl Pts',(-44.6536366700168,0.311138386869151,
4.52888423156623));
#32404=CARTESIAN_POINT('Ctrl Pts',(-44.5347276710218,-1.89031227931686,
4.12726531240721));
#32405=CARTESIAN_POINT('Ctrl Pts',(-44.4158186720269,-3.6324137491896,2.72271369023057));
#32406=CARTESIAN_POINT('Ctrl Pts',(-44.2969096730319,-4.49183230978425,
0.656537865318763));
#32407=CARTESIAN_POINT('Ctrl Pts',(-44.178000674037,-4.25972774921047,-1.56917780400555));
#32408=CARTESIAN_POINT('Ctrl Pts',(-44.059091675042,-2.9925018731896,-3.41358053176182));
#32409=CARTESIAN_POINT('Ctrl Pts',(-43.940182676047,-0.998092809298354,
-4.42847717693769));
#32410=CARTESIAN_POINT('Ctrl Pts',(-43.821273677052,1.2388545813571,-4.36724616652841));
#32411=CARTESIAN_POINT('Ctrl Pts',(-43.7023646780571,3.17475808804931,-3.24476656256246));
#32412=CARTESIAN_POINT('Ctrl Pts',(-43.5834556790621,4.33918991321652,-1.33380323702856));
#32413=CARTESIAN_POINT('Ctrl Pts',(-43.4645466800672,4.44919078769146,0.901277092518143));
#32414=CARTESIAN_POINT('Ctrl Pts',(-43.3456376810722,3.47803089423511,2.9173445518719));
#32415=CARTESIAN_POINT('Ctrl Pts',(-43.2267286820773,1.66170261573023,4.2244940813961));
#32416=CARTESIAN_POINT('Ctrl Pts',(-43.1078196830822,-0.558420751171717,
4.5050803342771));
#32417=CARTESIAN_POINT('Ctrl Pts',(-42.9889106840873,-2.64285000910083,
3.6909317730406));
#32418=CARTESIAN_POINT('Ctrl Pts',(-42.8700016850924,-4.08505587227025,
1.97986515005463));
#32419=CARTESIAN_POINT('Ctrl Pts',(-42.7510926860974,-4.53459839051628,
-0.212281901079125));
#32420=CARTESIAN_POINT('Ctrl Pts',(-42.6321836871025,-3.8822008248155,-2.35290448582148));
#32421=CARTESIAN_POINT('Ctrl Pts',(-42.5132746881075,-2.28647099457101,
-3.92164661926039));
#32422=CARTESIAN_POINT('Ctrl Pts',(-42.3943656891125,-0.135026251456862,
-4.53766227017941));
#32423=CARTESIAN_POINT('Ctrl Pts',(-42.2754566901175,2.04903365344401,-4.05053810450959));
#32424=CARTESIAN_POINT('Ctrl Pts',(-42.1565476911226,3.73556679230751,-2.58008372862802));
#32425=CARTESIAN_POINT('Ctrl Pts',(-42.0376386921276,4.51356845779047,-0.480753664312707));
#32426=CARTESIAN_POINT('Ctrl Pts',(-41.9187296931327,4.19632578309466,1.73158843219894));
#32427=CARTESIAN_POINT('Ctrl Pts',(-41.7998206941377,2.85625547461948,3.53074617269255));
#32428=CARTESIAN_POINT('Ctrl Pts',(-41.6809116951428,0.828308923028642,
4.45691773248095));
#32429=CARTESIAN_POINT('Ctrl Pts',(-41.5223663631495,-2.16015712884012,
4.28474797948406));
#32430=CARTESIAN_POINT('Ctrl Pts',(-41.3241846981579,-4.9740591081024,1.32908412483934));
#32431=CARTESIAN_POINT('Ctrl Pts',(-41.0863667001679,-3.80724186785295,
-3.46592527061159));
#32432=CARTESIAN_POINT('Ctrl Pts',(-40.8881850351764,0.0500896134690414,
-4.79821165639804));
#32433=CARTESIAN_POINT('Ctrl Pts',(-40.7296397031831,2.78352850293585,-3.5780134739008));
#32434=CARTESIAN_POINT('Ctrl Pts',(-40.6107307041881,4.15918402926478,-1.82360963009783));
#32435=CARTESIAN_POINT('Ctrl Pts',(-40.4918217051932,4.52276023745573,0.390113330814915));
#32436=CARTESIAN_POINT('Ctrl Pts',(-40.3729127061981,3.78802227944025,2.50086215521277));
#32437=CARTESIAN_POINT('Ctrl Pts',(-40.2540037072033,2.13242298822478,4.00799993834983));
#32438=CARTESIAN_POINT('Ctrl Pts',(-40.1350947082082,-0.0411755970567031,
4.53913013905057));
#32439=CARTESIAN_POINT('Ctrl Pts',(-40.0161857092133,-2.20486027926045,
3.96827445065634));
#32440=CARTESIAN_POINT('Ctrl Pts',(-39.8972767102183,-3.83271402254156,
2.43260457879703));
#32441=CARTESIAN_POINT('Ctrl Pts',(-39.7783677112234,-4.52923460703175,
0.306066394860525));
#32442=CARTESIAN_POINT('Ctrl Pts',(-39.6594587122284,-4.12513168363095,
-1.89497619022052));
#32443=CARTESIAN_POINT('Ctrl Pts',(-39.5405497132335,-2.71862032408285,
-3.63547122467695));
#32444=CARTESIAN_POINT('Ctrl Pts',(-39.4216407142385,-0.651476557450647,
-4.49257296200486));
#32445=CARTESIAN_POINT('Ctrl Pts',(-39.3027317152435,1.57397569950779,-4.25795526643815));
#32446=CARTESIAN_POINT('Ctrl Pts',(-39.1838227162486,3.41694983189919,-2.98865516129907));
#32447=CARTESIAN_POINT('Ctrl Pts',(-39.0649137172536,4.42959880069384,-0.993102512574686));
#32448=CARTESIAN_POINT('Ctrl Pts',(-38.9460047182586,4.36584768013456,1.24377373209122));
#32449=CARTESIAN_POINT('Ctrl Pts',(-38.8270957192637,3.24118782933984,3.17841180985207));
#32450=CARTESIAN_POINT('Ctrl Pts',(-38.7081867202687,1.32891370106109,4.34068973070986));
#32451=CARTESIAN_POINT('Ctrl Pts',(-38.5892777212737,-0.906288808862736,
4.44817269760705));
#32452=CARTESIAN_POINT('Ctrl Pts',(-38.4703687222788,-2.92126153819489,
3.47474177286519));
#32453=CARTESIAN_POINT('Ctrl Pts',(-38.3514597232838,-4.22636259933156,
1.65694257197947));
#32454=CARTESIAN_POINT('Ctrl Pts',(-38.2325507242889,-4.50445013822686,
-0.56349661064248));
#32455=CARTESIAN_POINT('Ctrl Pts',(-38.1136417252939,-3.68794839987019,
-2.64700511289908));
#32456=CARTESIAN_POINT('Ctrl Pts',(-37.9947327262989,-1.97526873561246,
-4.0872867413949));
#32457=CARTESIAN_POINT('Ctrl Pts',(-37.875823727304,0.217404693160681,-4.53435052369439));
#32458=CARTESIAN_POINT('Ctrl Pts',(-37.756914728309,2.35724840062552,-3.8795591832657));
#32459=CARTESIAN_POINT('Ctrl Pts',(-37.638005729314,3.92427661500994,-2.28202816042688));
#32460=CARTESIAN_POINT('Ctrl Pts',(-37.5190967303191,4.53769873376776,-0.12996029532479));
#32461=CARTESIAN_POINT('Ctrl Pts',(-37.4001877313241,4.04845210680413,2.05368814958598));
#32462=CARTESIAN_POINT('Ctrl Pts',(-37.2812787323292,2.57542452202649,3.7382867744424));
#32463=CARTESIAN_POINT('Ctrl Pts',(-37.1623697333342,0.476564264348535,
4.51447516094041));
#32464=CARTESIAN_POINT('Ctrl Pts',(-37.0434607343392,-1.73810194485508,
4.19363817060929));
#32465=CARTESIAN_POINT('Ctrl Pts',(-36.9245517353443,-3.53040633502461,
2.85373975449125));
#32466=CARTESIAN_POINT('Ctrl Pts',(-36.8056427363493,-4.4648157979083,0.820377576168181));
#32467=CARTESIAN_POINT('Ctrl Pts',(-36.6867337373543,-4.31426719625242,
-1.41233779106585));
#32468=CARTESIAN_POINT('Ctrl Pts',(-36.5678247383594,-3.11534410413089,
-3.30185259961615));
#32469=CARTESIAN_POINT('Ctrl Pts',(-36.4489157393644,-1.15938693432648,
-4.38901143917916));
#32470=CARTESIAN_POINT('Ctrl Pts',(-36.3300067403695,1.07830329261979,-4.40963280623902));
#32471=CARTESIAN_POINT('Ctrl Pts',(-36.2110977413745,3.05396392947723,-3.35870567245557));
#32472=CARTESIAN_POINT('Ctrl Pts',(-36.0921887423796,4.28750597867589,-1.49160717333758));
#32473=CARTESIAN_POINT('Ctrl Pts',(-35.9732797433846,4.47917656018556,0.73795448329676));
#32474=CARTESIAN_POINT('Ctrl Pts',(-35.8543707443897,3.58239938675126,2.78819190704975));
#32475=CARTESIAN_POINT('Ctrl Pts',(-35.7354617453947,1.81509288333212,4.1608938104223));
#32476=CARTESIAN_POINT('Ctrl Pts',(-35.6165527463997,-0.393284372117317,
4.52249122490932));
#32477=CARTESIAN_POINT('Ctrl Pts',(-35.4976437474047,-2.50609283581814,
3.78511534500529));
#32478=CARTESIAN_POINT('Ctrl Pts',(-35.3787347484098,-4.00991634789332,
2.12794980195292));
#32479=CARTESIAN_POINT('Ctrl Pts',(-35.2598257494148,-4.53932315910131,
-0.0463112727105621));
#32480=CARTESIAN_POINT('Ctrl Pts',(-35.1409167504199,-3.96566648640761,
-2.20931862693388));
#32481=CARTESIAN_POINT('Ctrl Pts',(-35.0220077514249,-2.42834590674615,
-3.83545768245756));
#32482=CARTESIAN_POINT('Ctrl Pts',(-34.9030987524299,-0.300933015493449,
-4.52957379859513));
#32483=CARTESIAN_POINT('Ctrl Pts',(-34.784189753435,1.89960712598062,-4.12299554252211));
#32484=CARTESIAN_POINT('Ctrl Pts',(-34.66528075444,3.63853940632953,-2.71452214308902));
#32485=CARTESIAN_POINT('Ctrl Pts',(-34.5463717554451,4.49330023353743,-0.646415105041655));
#32486=CARTESIAN_POINT('Ctrl Pts',(-34.4274627564501,4.25618122842175,1.57877193652657));
#32487=CARTESIAN_POINT('Ctrl Pts',(-34.3085537574552,2.98480272483288,3.4203146303467));
#32488=CARTESIAN_POINT('Ctrl Pts',(-34.1896447584602,0.988111927535212,
4.43071487408027));
#32489=CARTESIAN_POINT('Ctrl Pts',(-34.0707357594652,-1.24869180005395,
4.36444363753406));
#32490=CARTESIAN_POINT('Ctrl Pts',(-33.9518267604703,-3.18206123160157,
3.23760494734484));
#32491=CARTESIAN_POINT('Ctrl Pts',(-33.8329177614753,-4.3421842065533,1.32402258028056));
#32492=CARTESIAN_POINT('Ctrl Pts',(-33.7140087624803,-4.44714880860522,
-0.911299594455427));
#32493=CARTESIAN_POINT('Ctrl Pts',(-33.5950997634854,-3.47144845548349,
-2.92517437047002));
#32494=CARTESIAN_POINT('Ctrl Pts',(-33.4761907644904,-1.65218004314271,
-4.22822664739902));
#32495=CARTESIAN_POINT('Ctrl Pts',(-33.3572817654955,0.568571015518742,
-4.50381243803997));
#32496=CARTESIAN_POINT('Ctrl Pts',(-33.2383727665005,2.65115832085412,-3.68496391223899));
#32497=CARTESIAN_POINT('Ctrl Pts',(-33.1194637675055,4.08950950743749,-1.97066269698927));
#32498=CARTESIAN_POINT('Ctrl Pts',(-33.0005547685106,4.53410271588046,0.222513007678954));
#32499=CARTESIAN_POINT('Ctrl Pts',(-32.8816457695156,3.87690101727068,2.36161766148137));
#32500=CARTESIAN_POINT('Ctrl Pts',(-32.7627367705207,2.27760557628349,3.92684508423502));
#32501=CARTESIAN_POINT('Ctrl Pts',(-32.6438277715256,0.124847988200563,
4.53784226882032));
#32502=CARTESIAN_POINT('Ctrl Pts',(-32.5249187725308,-2.05824787981073,
4.04613582838238));
#32503=CARTESIAN_POINT('Ctrl Pts',(-32.4060097735357,-3.7411859055206,2.57121128994584));
#32504=CARTESIAN_POINT('Ctrl Pts',(-32.2871007745408,-4.51500919875398,
0.471477901174332));
#32505=CARTESIAN_POINT('Ctrl Pts',(-32.1681917755458,-4.19167734330492,
-1.74282544351886));
#32506=CARTESIAN_POINT('Ctrl Pts',(-32.0492827765509,-2.84976054604786,
-3.53361915160113));
#32507=CARTESIAN_POINT('Ctrl Pts',(-31.9303737775559,-0.815346942171119,
-4.46573721058515));
#32508=CARTESIAN_POINT('Ctrl Pts',(-31.8114647785609,1.41719739963958,-4.31267330363336));
#32509=CARTESIAN_POINT('Ctrl Pts',(-31.692555779566,3.30536028557706,-3.11162221793306));
#32510=CARTESIAN_POINT('Ctrl Pts',(-31.573646780571,4.39031483624702,-1.15444149335352));
#32511=CARTESIAN_POINT('Ctrl Pts',(-31.4547377815761,4.40841517156554,1.08327056534746));
#32512=CARTESIAN_POINT('Ctrl Pts',(-31.3358287825811,3.35526292348304,3.0577459225003));
#32513=CARTESIAN_POINT('Ctrl Pts',(-31.2169197835862,1.48677584407451,4.28918377176597));
#32514=CARTESIAN_POINT('Ctrl Pts',(-31.0980107845911,-0.743000251595862,
4.4783422257804));
#32515=CARTESIAN_POINT('Ctrl Pts',(-30.9791017855963,-2.79222622284383,
3.57925611035811));
#32516=CARTESIAN_POINT('Ctrl Pts',(-30.8601927866012,-4.16293585100342,
1.81040360708402));
#32517=CARTESIAN_POINT('Ctrl Pts',(-30.7412837876063,-4.52204572243967,
-0.398378390841908));
#32518=CARTESIAN_POINT('Ctrl Pts',(-30.6223747886113,-3.78228865854103,
-2.51035724352461));
#32519=CARTESIAN_POINT('Ctrl Pts',(-30.5034657896164,-2.12343261016916,
-4.01230789818306));
#32520=CARTESIAN_POINT('Ctrl Pts',(-30.3845567906214,0.0514288446811627,
-4.53927464464667));
#32521=CARTESIAN_POINT('Ctrl Pts',(-30.2656477916264,2.21377791403734,-3.96316187270984));
#32522=CARTESIAN_POINT('Ctrl Pts',(-30.1467387926315,3.83820517441539,-2.42404934636619));
#32523=CARTESIAN_POINT('Ctrl Pts',(-30.0278297936365,4.52988175982226,-0.295777679389505));
#32524=CARTESIAN_POINT('Ctrl Pts',(-29.9089207946416,4.12090930177574,1.90414584112476));
#32525=CARTESIAN_POINT('Ctrl Pts',(-29.7900117956466,2.71030542569923,3.64181896201337));
#32526=CARTESIAN_POINT('Ctrl Pts',(-29.71073912965,1.3311803135326,4.20948611409121));
#32527=CARTESIAN_POINT('Ctrl Pts',(-29.6711027966516,0.615324888853963,
4.3116474491314));
#32528=CARTESIAN_POINT('Ctrl Pts',(-52.575,2.36230756092333,-3.31488661006745));
#32529=CARTESIAN_POINT('Ctrl Pts',(-52.5353636670017,2.91267249451488,-2.92267674082431));
#32530=CARTESIAN_POINT('Ctrl Pts',(-52.456091001005,3.81372197207604,-1.85922435845946));
#32531=CARTESIAN_POINT('Ctrl Pts',(-52.3371820020101,4.2384739899776,0.188973964574656));
#32532=CARTESIAN_POINT('Ctrl Pts',(-52.2182730030151,3.63326518569111,2.1907646706185));
#32533=CARTESIAN_POINT('Ctrl Pts',(-52.0993640040202,2.14517071451495,3.66043213853357));
#32534=CARTESIAN_POINT('Ctrl Pts',(-51.9804550050252,0.135793741969793,
4.240490317549));
#32535=CARTESIAN_POINT('Ctrl Pts',(-51.8615460060302,-1.90658020276247,
3.79016093772832));
#32536=CARTESIAN_POINT('Ctrl Pts',(-51.7426370070353,-3.48565239142985,
2.41878623204276));
#32537=CARTESIAN_POINT('Ctrl Pts',(-51.6237280080403,-4.21770465133279,
0.459657053727601));
#32538=CARTESIAN_POINT('Ctrl Pts',(-51.5048190090453,-3.9248474328806,-1.61117702200155));
#32539=CARTESIAN_POINT('Ctrl Pts',(-51.3859100100504,-2.67824533662262,
-3.29048853499884));
#32540=CARTESIAN_POINT('Ctrl Pts',(-51.2670010110555,-0.78082496558402,
-4.17020743213141));
#32541=CARTESIAN_POINT('Ctrl Pts',(-51.1480920120604,1.30633725885353,-4.03655767907646));
#32542=CARTESIAN_POINT('Ctrl Pts',(-51.0291830130655,3.07605723061235,-2.9220178035111));
#32543=CARTESIAN_POINT('Ctrl Pts',(-50.9102740140706,4.09828990837908,-1.0974222453584));
#32544=CARTESIAN_POINT('Ctrl Pts',(-50.7913650150755,4.12463095289654,0.993848724235651));
#32545=CARTESIAN_POINT('Ctrl Pts',(-50.6724560160807,3.14867944761336,2.84361277085736));
#32546=CARTESIAN_POINT('Ctrl Pts',(-50.5535470170857,1.40759331717813,4.00237390050092));
#32547=CARTESIAN_POINT('Ctrl Pts',(-50.4346380180907,-0.675540456184353,
4.18855117202478));
#32548=CARTESIAN_POINT('Ctrl Pts',(-50.3157290190957,-2.59451671479358,
3.35690315989496));
#32549=CARTESIAN_POINT('Ctrl Pts',(-50.1968200201008,-3.88302086412996,
1.7095217998619));
#32550=CARTESIAN_POINT('Ctrl Pts',(-50.0779110211058,-4.22794413760432,
-0.353276355744105));
#32551=CARTESIAN_POINT('Ctrl Pts',(-49.9590020221109,-3.54546957514818,
-2.33022773676946));
#32552=CARTESIAN_POINT('Ctrl Pts',(-49.8400930231158,-2.00143969166412,
-3.74092969395146));
#32553=CARTESIAN_POINT('Ctrl Pts',(-49.721184024121,0.0289435448964663,
-4.2425791784024));
#32554=CARTESIAN_POINT('Ctrl Pts',(-49.6022750251259,2.05229344931449,-3.71327448649327));
#32555=CARTESIAN_POINT('Ctrl Pts',(-49.4833660261311,3.57693244841941,-2.28163758591345));
#32556=CARTESIAN_POINT('Ctrl Pts',(-49.364457027136,4.23237059313566,-0.295558752875362));
#32557=CARTESIAN_POINT('Ctrl Pts',(-49.2455480281411,3.85933526548734,1.76234137516302));
#32558=CARTESIAN_POINT('Ctrl Pts',(-49.1266390291461,2.54847470392539,3.39198946010828));
#32559=CARTESIAN_POINT('Ctrl Pts',(-49.0077300301511,0.618330322503512,
4.19737816098522));
#32560=CARTESIAN_POINT('Ctrl Pts',(-48.8888210311563,-1.46206941105725,
3.98279661184051));
#32561=CARTESIAN_POINT('Ctrl Pts',(-48.7699120321612,-3.18718371510779,
2.80038850522416));
#32562=CARTESIAN_POINT('Ctrl Pts',(-48.6510030331662,-4.13780679009204,
0.937481083493075));
#32563=CARTESIAN_POINT('Ctrl Pts',(-48.5320940341714,-4.08293556259652,
-1.15323588468445));
#32564=CARTESIAN_POINT('Ctrl Pts',(-48.4131850351763,-3.03590383707744,
-2.96371451156447));
#32565=CARTESIAN_POINT('Ctrl Pts',(-48.2942760361814,-1.2511421580073,-4.05400531752194));
#32566=CARTESIAN_POINT('Ctrl Pts',(-48.1753670371864,0.837649258381883,
-4.15916572571611));
#32567=CARTESIAN_POINT('Ctrl Pts',(-48.0564580381915,2.72289043680534,-3.25364157263724));
#32568=CARTESIAN_POINT('Ctrl Pts',(-47.9375490391965,3.94646446657405,-1.55747681462926));
#32569=CARTESIAN_POINT('Ctrl Pts',(-47.8186400402015,4.21104071385062,0.517157539180999));
#32570=CARTESIAN_POINT('Ctrl Pts',(-47.6997310412066,3.45232668681426,2.46612170452907));
#32571=CARTESIAN_POINT('Ctrl Pts',(-47.5808220422116,1.85469122386101,3.81581397321361));
#32572=CARTESIAN_POINT('Ctrl Pts',(-47.4619130432167,-0.193637457276558,
4.23825675828857));
#32573=CARTESIAN_POINT('Ctrl Pts',(-47.3430040442216,-2.19491189690037,
3.6307957225496));
#32574=CARTESIAN_POINT('Ctrl Pts',(-47.2240950452268,-3.66281889847391,
2.14104496240076));
#32575=CARTESIAN_POINT('Ctrl Pts',(-47.1051860462317,-4.24065448775976,
0.131016523699623));
#32576=CARTESIAN_POINT('Ctrl Pts',(-46.9862770472369,-3.78800360376758,
-1.91084915989804));
#32577=CARTESIAN_POINT('Ctrl Pts',(-46.8673680482418,-2.41486120468549,
-3.4883751484243));
#32578=CARTESIAN_POINT('Ctrl Pts',(-46.748459049247,-0.454903300248022,
-4.21821986167895));
#32579=CARTESIAN_POINT('Ctrl Pts',(-46.6295500502518,1.61559690347559,-3.92302975511522));
#32580=CARTESIAN_POINT('Ctrl Pts',(-46.510641051257,3.29350422793804,-2.67453654201874));
#32581=CARTESIAN_POINT('Ctrl Pts',(-46.391732052262,4.17108425236453,-0.776126261452312));
#32582=CARTESIAN_POINT('Ctrl Pts',(-46.2728230532671,4.03508349265237,1.3108840609923));
#32583=CARTESIAN_POINT('Ctrl Pts',(-46.153914054272,2.91855037178518,3.0793472589807));
#32584=CARTESIAN_POINT('Ctrl Pts',(-46.0350050552771,1.09280439512275,4.09952367575057));
#32585=CARTESIAN_POINT('Ctrl Pts',(-45.9160960562821,-0.998494964953347,
4.123508653926));
#32586=CARTESIAN_POINT('Ctrl Pts',(-45.7971870572872,-2.84715829844654,
3.14547380177063));
#32587=CARTESIAN_POINT('Ctrl Pts',(-45.6782780582922,-4.00395717509747,
1.40308330259685));
#32588=CARTESIAN_POINT('Ctrl Pts',(-45.5593690592973,-4.18778744031509,
-0.680258898345004));
#32589=CARTESIAN_POINT('Ctrl Pts',(-45.4404600603022,-3.35397801744653,
-2.59829699467222));
#32590=CARTESIAN_POINT('Ctrl Pts',(-45.3215510613074,-1.70514605769533,
-3.88494436716616));
#32591=CARTESIAN_POINT('Ctrl Pts',(-45.2026420623123,0.358039382745663,
-4.22754344914553));
#32592=CARTESIAN_POINT('Ctrl Pts',(-45.0837330633174,2.33422062563635,-3.54284206322451));
#32593=CARTESIAN_POINT('Ctrl Pts',(-44.9648240643225,3.74318216521078,-1.997223846241));
#32594=CARTESIAN_POINT('Ctrl Pts',(-44.8459150653275,4.24254387784786,0.0337232659310005));
#32595=CARTESIAN_POINT('Ctrl Pts',(-44.7270060663325,3.71095999205786,2.05647556548625));
#32596=CARTESIAN_POINT('Ctrl Pts',(-44.6080970673375,2.27760632395248,3.57950069794286));
#32597=CARTESIAN_POINT('Ctrl Pts',(-44.4891880683426,0.290790326898236,
4.23270088732366));
#32598=CARTESIAN_POINT('Ctrl Pts',(-44.3702790693477,-1.76668822890541,
3.85734734137919));
#32599=CARTESIAN_POINT('Ctrl Pts',(-44.2513700703527,-3.39485844927514,
2.54465163234734));
#32600=CARTESIAN_POINT('Ctrl Pts',(-44.1324610713577,-4.19807211471991,
0.61360111299095));
#32601=CARTESIAN_POINT('Ctrl Pts',(-44.0135520723628,-3.98114690107788,
-1.46655554520236));
#32602=CARTESIAN_POINT('Ctrl Pts',(-43.8946430733678,-2.79679600676983,
-3.19033664959511));
#32603=CARTESIAN_POINT('Ctrl Pts',(-43.7757340743728,-0.932818792342456,
-4.1388603280403));
#32604=CARTESIAN_POINT('Ctrl Pts',(-43.6568250753779,1.15783504670461,-4.0816337488567));
#32605=CARTESIAN_POINT('Ctrl Pts',(-43.5379160763829,2.96713289393957,-3.03256290209179));
#32606=CARTESIAN_POINT('Ctrl Pts',(-43.4190070773879,4.05541233929616,-1.24657417947145));
#32607=CARTESIAN_POINT('Ctrl Pts',(-43.300098078393,4.15821929464979,0.842334701919917));
#32608=CARTESIAN_POINT('Ctrl Pts',(-43.181189079398,3.25057203925852,2.72655387993142));
#32609=CARTESIAN_POINT('Ctrl Pts',(-43.0622800804031,1.55302935037421,3.94821747091449));
#32610=CARTESIAN_POINT('Ctrl Pts',(-42.9433710814082,-0.521900734955894,
4.21045373503939));
#32611=CARTESIAN_POINT('Ctrl Pts',(-42.824462082413,-2.47001093572135,3.44954946781609));
#32612=CARTESIAN_POINT('Ctrl Pts',(-42.7055530834183,-3.81789834564735,
1.85038445430061));
#32613=CARTESIAN_POINT('Ctrl Pts',(-42.5866440844232,-4.23804134745061,
-0.198398931197613));
#32614=CARTESIAN_POINT('Ctrl Pts',(-42.4677350854283,-3.62830976367934,
-2.19902748573468));
#32615=CARTESIAN_POINT('Ctrl Pts',(-42.3488260864333,-2.13693866142688,
-3.66517585267858));
#32616=CARTESIAN_POINT('Ctrl Pts',(-42.2299170874383,-0.126195704091931,
-4.24090485322945));
#32617=CARTESIAN_POINT('Ctrl Pts',(-42.1110080884434,1.91502942438633,-3.78563799657268));
#32618=CARTESIAN_POINT('Ctrl Pts',(-41.9920990894484,3.49126541284734,-2.41134949120931));
#32619=CARTESIAN_POINT('Ctrl Pts',(-41.8731900904535,4.21838674592901,-0.449312978092323));
#32620=CARTESIAN_POINT('Ctrl Pts',(-41.7542810914585,3.92189134396604,1.61834472216421));
#32621=CARTESIAN_POINT('Ctrl Pts',(-41.6353720924635,2.66945995165433,3.29983980467131));
#32622=CARTESIAN_POINT('Ctrl Pts',(-41.5164630934686,0.77413855912781,4.16544090694865));
#32623=CARTESIAN_POINT('Ctrl Pts',(-41.3579177614753,-2.01888556396995,
4.00453083969612));
#32624=CARTESIAN_POINT('Ctrl Pts',(-41.1597360964837,-4.64876188570278,
1.24216369129613));
#32625=CARTESIAN_POINT('Ctrl Pts',(-40.9219180984938,-3.5582530284162,-3.23925810822545));
#32626=CARTESIAN_POINT('Ctrl Pts',(-40.7237364335021,0.0468138156189731,
-4.48441463662212));
#32627=CARTESIAN_POINT('Ctrl Pts',(-40.5651911015089,2.60148923263442,-3.34401588370882));
#32628=CARTESIAN_POINT('Ctrl Pts',(-40.4462821025139,3.88717861421759,-1.70434784922236));
#32629=CARTESIAN_POINT('Ctrl Pts',(-40.327373103519,4.22697739474136,0.364600408636661));
#32630=CARTESIAN_POINT('Ctrl Pts',(-40.208464104524,3.54029037696192,2.33730890925922));
#32631=CARTESIAN_POINT('Ctrl Pts',(-40.0895551055291,1.99296520133986,3.74588177308733));
#32632=CARTESIAN_POINT('Ctrl Pts',(-39.9706461065341,-0.0384827646914282,
4.24227672531885));
#32633=CARTESIAN_POINT('Ctrl Pts',(-39.8517371075391,-2.06066518446267,
3.70875428242689));
#32634=CARTESIAN_POINT('Ctrl Pts',(-39.7328281085442,-3.58205933615999,
2.27351529266644));
#32635=CARTESIAN_POINT('Ctrl Pts',(-39.6139191095492,-4.23302834867352,
0.28605003680078));
#32636=CARTESIAN_POINT('Ctrl Pts',(-39.4950101105542,-3.85535324924685,
-1.77104712588996));
#32637=CARTESIAN_POINT('Ctrl Pts',(-39.3761011115593,-2.54082596720782,
-3.39771596970325));
#32638=CARTESIAN_POINT('Ctrl Pts',(-39.2571921125643,-0.608870808304631,
-4.19876432921494));
#32639=CARTESIAN_POINT('Ctrl Pts',(-39.1382831135694,1.47103966436091,-3.97949033645411));
#32640=CARTESIAN_POINT('Ctrl Pts',(-39.0193741145744,3.19348560173252,-2.79320086500867));
#32641=CARTESIAN_POINT('Ctrl Pts',(-38.9004651155794,4.13990859901063,-0.928154854760866));
#32642=CARTESIAN_POINT('Ctrl Pts',(-38.7815561165844,4.08032672171768,1.16243249115508));
#32643=CARTESIAN_POINT('Ctrl Pts',(-38.6626471175895,3.02921821353002,2.97054766692245));
#32644=CARTESIAN_POINT('Ctrl Pts',(-38.5437381185945,1.24200441301907,4.05681407060795));
#32645=CARTESIAN_POINT('Ctrl Pts',(-38.4248291195996,-0.84701865830611,
4.15726778637903));
#32646=CARTESIAN_POINT('Ctrl Pts',(-38.3059201206046,-2.73021470026535,
3.2474980222978));
#32647=CARTESIAN_POINT('Ctrl Pts',(-38.1870111216096,-3.94996379012226,
1.5485806075101));
#32648=CARTESIAN_POINT('Ctrl Pts',(-38.0681021226147,-4.20986475301984,
-0.526644639588315));
#32649=CARTESIAN_POINT('Ctrl Pts',(-37.9491931236197,-3.44676120350641,
-2.47389430094654));
#32650=CARTESIAN_POINT('Ctrl Pts',(-37.8302841246248,-1.8460886395937,-3.81998331873136));
#32651=CARTESIAN_POINT('Ctrl Pts',(-37.7113751256298,0.203186699106992,
-4.23780969080775));
#32652=CARTESIAN_POINT('Ctrl Pts',(-37.5924661266349,2.20308731396286,-3.6258408821712));
#32653=CARTESIAN_POINT('Ctrl Pts',(-37.4735571276399,3.6676338500072,-2.13278638305928));
#32654=CARTESIAN_POINT('Ctrl Pts',(-37.3546481286449,4.24093893214488,-0.121461055132279));
#32655=CARTESIAN_POINT('Ctrl Pts',(-37.23573912965,3.78368842049889,1.91937952232278));
#32656=CARTESIAN_POINT('Ctrl Pts',(-37.116830130655,2.40699499087144,3.49380751156464));
#32657=CARTESIAN_POINT('Ctrl Pts',(-36.9979211316601,0.445397559627416,
4.219234151831));
#32658=CARTESIAN_POINT('Ctrl Pts',(-36.8790121326651,-1.62443225926818,
3.91937949796381));
#32659=CARTESIAN_POINT('Ctrl Pts',(-36.7601031336701,-3.2995221919603,2.66710875646485));
#32660=CARTESIAN_POINT('Ctrl Pts',(-36.6411941346751,-4.17282244881044,
0.766725912396867));
#32661=CARTESIAN_POINT('Ctrl Pts',(-36.5222851356802,-4.03211953673935,
-1.31997267224866));
#32662=CARTESIAN_POINT('Ctrl Pts',(-36.4033761366853,-2.91160450999496,
-3.08591558397465));
#32663=CARTESIAN_POINT('Ctrl Pts',(-36.2844671376902,-1.08356448404466,
-4.10197559999513));
#32664=CARTESIAN_POINT('Ctrl Pts',(-36.1655581386953,1.00778361073219,-4.1212483555325));
#32665=CARTESIAN_POINT('Ctrl Pts',(-36.0466491397003,2.85423852172137,-3.1390505372104));
#32666=CARTESIAN_POINT('Ctrl Pts',(-35.9277401407054,4.00710846920256,-1.394057936416));
#32667=CARTESIAN_POINT('Ctrl Pts',(-35.8088311417104,4.18624403525991,0.689693186344611));
#32668=CARTESIAN_POINT('Ctrl Pts',(-35.6899221427155,3.34811496336391,2.60584765597262));
#32669=CARTESIAN_POINT('Ctrl Pts',(-35.5710131437205,1.69638808700519,3.88877657783347));
#32670=CARTESIAN_POINT('Ctrl Pts',(-35.4521041447256,-0.36756406781807,
4.22672597527783));
#32671=CARTESIAN_POINT('Ctrl Pts',(-35.3331951457305,-2.34219750991838,
3.53757355239032));
#32672=CARTESIAN_POINT('Ctrl Pts',(-35.2142861467357,-3.74767285185209,
1.98878455583559));
#32673=CARTESIAN_POINT('Ctrl Pts',(-35.0953771477406,-4.24245712210054,
-0.0432825736036531));
#32674=CARTESIAN_POINT('Ctrl Pts',(-34.9764681487457,-3.70631687576659,
-2.06483196179423));
#32675=CARTESIAN_POINT('Ctrl Pts',(-34.8575591497507,-2.26953513242235,
-3.58462356416123));
#32676=CARTESIAN_POINT('Ctrl Pts',(-34.7386501507558,-0.281252374001066,
-4.2333453575344));
#32677=CARTESIAN_POINT('Ctrl Pts',(-34.6197411517608,1.77537520426393,-3.8533568090853));
#32678=CARTESIAN_POINT('Ctrl Pts',(-34.5008321527659,3.40058349612684,-2.5369958021071));
#32679=CARTESIAN_POINT('Ctrl Pts',(-34.3819231537709,4.19944403810212,-0.604140368530221));
#32680=CARTESIAN_POINT('Ctrl Pts',(-34.2630141547759,3.97783231829727,1.47552223349874));
#32681=CARTESIAN_POINT('Ctrl Pts',(-34.144105155781,2.78960037305193,3.19663034658495));
#32682=CARTESIAN_POINT('Ctrl Pts',(-34.025196156786,0.92349064771896,4.14095168259845));
#32683=CARTESIAN_POINT('Ctrl Pts',(-33.9062871577911,-1.16702892364603,
4.07901450174094));
#32684=CARTESIAN_POINT('Ctrl Pts',(-33.7873781587961,-2.97395842107017,
3.02586964752038));
#32685=CARTESIAN_POINT('Ctrl Pts',(-33.6684691598011,-4.05821080960704,
1.23743316539842));
#32686=CARTESIAN_POINT('Ctrl Pts',(-33.5495601608062,-4.15631085843277,
-0.851701744810404));
#32687=CARTESIAN_POINT('Ctrl Pts',(-33.4306511618112,-3.24442008373921,
-2.73387163822095));
#32688=CARTESIAN_POINT('Ctrl Pts',(-33.3117421628162,-1.5441295420815,-3.95170593178579));
#32689=CARTESIAN_POINT('Ctrl Pts',(-33.1928331638213,0.531387184754894,
-4.20926875762475));
#32690=CARTESIAN_POINT('Ctrl Pts',(-33.0739241648263,2.47777589431427,-3.44397189762026));
#32691=CARTESIAN_POINT('Ctrl Pts',(-32.9550151658313,3.82206071866471,-1.84178383011512));
#32692=CARTESIAN_POINT('Ctrl Pts',(-32.8361061668364,4.23757808931381,0.207960936267553));
#32693=CARTESIAN_POINT('Ctrl Pts',(-32.7171971678414,3.62335655689582,2.20717083064289));
#32694=CARTESIAN_POINT('Ctrl Pts',(-32.5982881688465,2.12865303036779,3.67003434456881));
#32695=CARTESIAN_POINT('Ctrl Pts',(-32.4793791698515,0.116683086477182,
4.24107308018517));
#32696=CARTESIAN_POINT('Ctrl Pts',(-32.3604701708566,-1.92364105191405,
3.78152362377861));
#32697=CARTESIAN_POINT('Ctrl Pts',(-32.2415611718616,-3.49651704310921,
2.40305729888056));
#32698=CARTESIAN_POINT('Ctrl Pts',(-32.1226521728666,-4.21973326424187,
0.440643838220576));
#32699=CARTESIAN_POINT('Ctrl Pts',(-32.0037431738717,-3.91754690630399,
-1.62884684704813));
#32700=CARTESIAN_POINT('Ctrl Pts',(-31.8848341748767,-2.66338978325909,
-3.30252489436533));
#32701=CARTESIAN_POINT('Ctrl Pts',(-31.7659251758817,-0.762024275548931,
-4.17368360225475));
#32702=CARTESIAN_POINT('Ctrl Pts',(-31.6470161768868,1.32451446852128,-4.03062988269698));
#32703=CARTESIAN_POINT('Ctrl Pts',(-31.5281071778918,3.08919387167645,-2.90812603048288));
#32704=CARTESIAN_POINT('Ctrl Pts',(-31.4091981788968,4.10319375653073,-1.07894246870398));
#32705=CARTESIAN_POINT('Ctrl Pts',(-31.2902891799019,4.12011035263834,1.01242603005823));
#32706=CARTESIAN_POINT('Ctrl Pts',(-31.1713801809069,3.13583293969945,2.85777317714776));
#32707=CARTESIAN_POINT('Ctrl Pts',(-31.0524711819119,1.38954257002262,4.00867653673046));
#32708=CARTESIAN_POINT('Ctrl Pts',(-30.933562182917,-0.694408967730227,
4.18546426527762));
#32709=CARTESIAN_POINT('Ctrl Pts',(-30.8146531839221,-2.6096181325775,3.34517725330154));
#32710=CARTESIAN_POINT('Ctrl Pts',(-30.6957441849271,-3.89068507152368,
1.6920054835379));
#32711=CARTESIAN_POINT('Ctrl Pts',(-30.5768351859321,-4.22630960811051,
-0.37232494411191));
#32712=CARTESIAN_POINT('Ctrl Pts',(-30.4579261869372,-3.53493172767287,
-2.34618303071339));
#32713=CARTESIAN_POINT('Ctrl Pts',(-30.3390171879422,-1.98456278272466,
-3.74990799775467));
#32714=CARTESIAN_POINT('Ctrl Pts',(-30.2201081889473,0.0480654627907762,
-4.24241178043034));
#32715=CARTESIAN_POINT('Ctrl Pts',(-30.1011991899523,2.06899961711827,-3.70397606066096));
#32716=CARTESIAN_POINT('Ctrl Pts',(-29.9822901909573,3.58719137359357,-2.26551956169834));
#32717=CARTESIAN_POINT('Ctrl Pts',(-29.8633811919623,4.23363317848382,-0.276434190407516));
#32718=CARTESIAN_POINT('Ctrl Pts',(-29.7444721929674,3.85140700586516,1.77961709313449));
#32719=CARTESIAN_POINT('Ctrl Pts',(-29.6255631939724,2.53305485274192,3.40364857298535));
#32720=CARTESIAN_POINT('Ctrl Pts',(-29.5462905279758,1.24412279187993,3.93419100583383));
#32721=CARTESIAN_POINT('Ctrl Pts',(-29.5066541949775,0.575083413457821,
4.02967111779183));
#32722=CARTESIAN_POINT('',(-30.,0.695807839646249,4.87560011181053));
#32723=CARTESIAN_POINT('Ctrl Pts',(-30.,3.27123863458584,-2.42269058837956));
#32724=CARTESIAN_POINT('Ctrl Pts',(-30.,3.33974878250541,-2.34761006208624));
#32725=CARTESIAN_POINT('Ctrl Pts',(-30.,3.40533192358328,-2.27003566591244));
#32726=CARTESIAN_POINT('Ctrl Pts',(-30.,3.46783702656801,-2.19012891506847));
#32727=CARTESIAN_POINT('Ctrl Pts',(-30.,3.54519073167044,-2.09123965730679));
#32728=CARTESIAN_POINT('Ctrl Pts',(-30.,3.61783178849963,-1.98877939676093));
#32729=CARTESIAN_POINT('Ctrl Pts',(-30.,3.68567008600155,-1.88315345760476));
#32730=CARTESIAN_POINT('Ctrl Pts',(-30.,3.72452568859522,-1.82265430496434));
#32731=CARTESIAN_POINT('Ctrl Pts',(-30.,3.76180511742509,-1.76111580012076));
#32732=CARTESIAN_POINT('Ctrl Pts',(-30.,3.79748638403424,-1.69860841143877));
#32733=CARTESIAN_POINT('Ctrl Pts',(-30.,3.81574456349527,-1.66662324867262));
#32734=CARTESIAN_POINT('Ctrl Pts',(-30.,3.8335842187764,-1.63438433328503));
#32735=CARTESIAN_POINT('Ctrl Pts',(-30.,3.85100199058494,-1.60190075176667));
#32736=CARTESIAN_POINT('Ctrl Pts',(-30.,3.86219018238585,-1.58103513563606));
#32737=CARTESIAN_POINT('Ctrl Pts',(-30.,3.87320429714474,-1.56006856433113));
#32738=CARTESIAN_POINT('Ctrl Pts',(-30.,3.8840433802687,-1.5390033991797));
#32739=CARTESIAN_POINT('Ctrl Pts',(-30.,3.8935038434821,-1.52061750641368));
#32740=CARTESIAN_POINT('Ctrl Pts',(-30.,3.90282656389723,-1.5021650534667));
#32741=CARTESIAN_POINT('Ctrl Pts',(-30.,3.91201089233721,-1.48364853923209));
#32742=CARTESIAN_POINT('Ctrl Pts',(-30.,3.96947385833632,-1.36779751813259));
#32743=CARTESIAN_POINT('Ctrl Pts',(-30.,4.02152672316031,-1.24943342811707));
#32744=CARTESIAN_POINT('Ctrl Pts',(-30.,4.06807409839169,-1.12898161068632));
#32745=CARTESIAN_POINT('Ctrl Pts',(-30.,4.11491088273489,-1.00778088199419));
#32746=CARTESIAN_POINT('Ctrl Pts',(-30.,4.1561739627056,-0.88446569930994));
#32747=CARTESIAN_POINT('Ctrl Pts',(-30.,4.19172616679095,-0.759434914895517));
#32748=CARTESIAN_POINT('Ctrl Pts',(-30.,4.2041994658364,-0.715568538562162));
#32749=CARTESIAN_POINT('Ctrl Pts',(-30.,4.21596941142744,-0.671490725785992));
#32750=CARTESIAN_POINT('Ctrl Pts',(-30.,4.22702875952034,-0.627217950078772));
#32751=CARTESIAN_POINT('Ctrl Pts',(-30.,4.23745336325369,-0.58548618261418));
#32752=CARTESIAN_POINT('Ctrl Pts',(-30.,4.24724659311391,-0.543581183826834));
#32753=CARTESIAN_POINT('Ctrl Pts',(-30.,4.25640178065254,-0.501516507038128));
#32754=CARTESIAN_POINT('Ctrl Pts',(-30.,4.26067116719361,-0.481900266062384));
#32755=CARTESIAN_POINT('Ctrl Pts',(-30.,4.26479982210057,-0.462258272543662));
#32756=CARTESIAN_POINT('Ctrl Pts',(-30.,4.26878682150122,-0.442595092139843));
#32757=CARTESIAN_POINT('Ctrl Pts',(-30.,4.27969785634821,-0.38878378568377));
#32758=CARTESIAN_POINT('Ctrl Pts',(-30.,4.28954967875665,-0.334806539222378));
#32759=CARTESIAN_POINT('Ctrl Pts',(-30.,4.29833606013692,-0.280694354437186));
#32760=CARTESIAN_POINT('Ctrl Pts',(-30.,4.31910350792121,-0.152795060816309));
#32761=CARTESIAN_POINT('Ctrl Pts',(-30.,4.33392210423418,-0.0241436844331786));
#32762=CARTESIAN_POINT('Ctrl Pts',(-30.,4.34293706986683,0.104855255691433));
#32763=CARTESIAN_POINT('Ctrl Pts',(-30.,4.35209692663439,0.235927504090205));
#32764=CARTESIAN_POINT('Ctrl Pts',(-30.,4.35526525016914,0.367359263948117));
#32765=CARTESIAN_POINT('Ctrl Pts',(-30.,4.3525451613485,0.498747926672244));
#32766=CARTESIAN_POINT('Ctrl Pts',(-30.,4.35009455980085,0.617119524603827));
#32767=CARTESIAN_POINT('Ctrl Pts',(-30.,4.342863896526,0.735456818994498));
#32768=CARTESIAN_POINT('Ctrl Pts',(-30.,4.33089384577612,0.85347290367371));
#32769=CARTESIAN_POINT('Ctrl Pts',(-30.,4.32191630771371,0.941984967183119));
#32770=CARTESIAN_POINT('Ctrl Pts',(-30.,4.3102721913265,1.03031653659682));
#32771=CARTESIAN_POINT('Ctrl Pts',(-30.,4.29596640419823,1.11834673365244));
#32772=CARTESIAN_POINT('Ctrl Pts',(-30.,4.29282291216298,1.1376901099256));
#32773=CARTESIAN_POINT('Ctrl Pts',(-30.,4.28955086420591,1.15701893097116));
#32774=CARTESIAN_POINT('Ctrl Pts',(-30.,4.28615024400599,1.17633190572179));
#32775=CARTESIAN_POINT('Ctrl Pts',(-30.,4.28275399423854,1.1956200596906));
#32776=CARTESIAN_POINT('Ctrl Pts',(-30.,4.27923068225399,1.21488549492892));
#32777=CARTESIAN_POINT('Ctrl Pts',(-30.,4.27558221590421,1.2341187299655));
#32778=CARTESIAN_POINT('Ctrl Pts',(-30.,4.25019481772672,1.36795079782698));
#32779=CARTESIAN_POINT('Ctrl Pts',(-30.,4.2187302622092,1.50034532596835));
#32780=CARTESIAN_POINT('Ctrl Pts',(-30.,4.18131898274086,1.63087582632965));
#32781=CARTESIAN_POINT('Ctrl Pts',(-30.,4.15599233816626,1.7192422130391));
#32782=CARTESIAN_POINT('Ctrl Pts',(-30.,4.1279392470965,1.80675472203661));
#32783=CARTESIAN_POINT('Ctrl Pts',(-30.,4.09718685463689,1.89328334475779));
#32784=CARTESIAN_POINT('Ctrl Pts',(-30.,4.05202657818314,2.02035171930402));
#32785=CARTESIAN_POINT('Ctrl Pts',(-30.,4.00104764212238,2.1452989823121));
#32786=CARTESIAN_POINT('Ctrl Pts',(-30.,3.9445356482452,2.26782052204027));
#32787=CARTESIAN_POINT('Ctrl Pts',(-30.,3.88754811032845,2.39137307100984));
#32788=CARTESIAN_POINT('Ctrl Pts',(-30.,3.82493372767001,2.51245961368684));
#32789=CARTESIAN_POINT('Ctrl Pts',(-30.,3.75693418422412,2.63075452573071));
#32790=CARTESIAN_POINT('Ctrl Pts',(-30.,3.737983670491,2.66372164935602));
#32791=CARTESIAN_POINT('Ctrl Pts',(-30.,3.71861462433676,2.6964718440802));
#32792=CARTESIAN_POINT('Ctrl Pts',(-30.,3.69883162247989,2.72899776234456));
#32793=CARTESIAN_POINT('Ctrl Pts',(-30.,3.68688439772594,2.74864060818989));
#32794=CARTESIAN_POINT('Ctrl Pts',(-30.,3.67478619315373,2.76820165491218));
#32795=CARTESIAN_POINT('Ctrl Pts',(-30.,3.66253796903456,2.78767925573459));
#32796=CARTESIAN_POINT('Ctrl Pts',(-30.,3.65179479048755,2.80476347474192));
#32797=CARTESIAN_POINT('Ctrl Pts',(-30.,3.64093530565375,2.82178475520501));
#32798=CARTESIAN_POINT('Ctrl Pts',(-30.,3.62997054880261,2.83872623143875));
#32799=CARTESIAN_POINT('Ctrl Pts',(-30.,3.55452366838117,2.95529803954384));
#32800=CARTESIAN_POINT('Ctrl Pts',(-30.,3.47399244884128,3.06826045209769));
#32801=CARTESIAN_POINT('Ctrl Pts',(-30.,3.38870779675817,3.17730699510021));
#32802=CARTESIAN_POINT('Ctrl Pts',(-30.,3.30236442727477,3.28770723386977));
#32803=CARTESIAN_POINT('Ctrl Pts',(-30.,3.2111485886733,3.39409451140229));
#32804=CARTESIAN_POINT('Ctrl Pts',(-30.,3.11535169160701,3.49613785110227));
#32805=CARTESIAN_POINT('Ctrl Pts',(-30.,3.02057348092696,3.59709608090682));
#32806=CARTESIAN_POINT('Ctrl Pts',(-30.,2.92131065748878,3.6938029330822));
#32807=CARTESIAN_POINT('Ctrl Pts',(-30.,2.81780079208004,3.78591489553778));
#32808=CARTESIAN_POINT('Ctrl Pts',(-30.,2.74290681629881,3.85256198331119));
#32809=CARTESIAN_POINT('Ctrl Pts',(-30.,2.66578849251642,3.91680311881087));
#32810=CARTESIAN_POINT('Ctrl Pts',(-30.,2.58658176109254,3.97857999207842));
#32811=CARTESIAN_POINT('Ctrl Pts',(-30.,2.55153627131115,4.00591353737064));
#32812=CARTESIAN_POINT('Ctrl Pts',(-30.,2.51608180945682,4.03276453049069));
#32813=CARTESIAN_POINT('Ctrl Pts',(-30.,2.48022957230527,4.05912727077957));
#32814=CARTESIAN_POINT('Ctrl Pts',(-30.,2.45986378047589,4.07410257283691));
#32815=CARTESIAN_POINT('Ctrl Pts',(-30.,2.4393696290117,4.08892031865678));
#32816=CARTESIAN_POINT('Ctrl Pts',(-30.,2.41874912476045,4.10357940212803));
#32817=CARTESIAN_POINT('Ctrl Pts',(-30.,2.40331171174522,4.11455383433459));
#32818=CARTESIAN_POINT('Ctrl Pts',(-30.,2.38780322466491,4.12543944891267));
#32819=CARTESIAN_POINT('Ctrl Pts',(-30.,2.37223705386536,4.13622726943165));
#32820=CARTESIAN_POINT('Ctrl Pts',(-30.,2.25664934302075,4.21633299966218));
#32821=CARTESIAN_POINT('Ctrl Pts',(-30.,2.13771882511829,4.291167679162));
#32822=CARTESIAN_POINT('Ctrl Pts',(-30.,2.01587786606652,4.36063638947179));
#32823=CARTESIAN_POINT('Ctrl Pts',(-30.,1.89144311327298,4.43158397443468));
#32824=CARTESIAN_POINT('Ctrl Pts',(-30.,1.76397219298052,4.49693520894599));
#32825=CARTESIAN_POINT('Ctrl Pts',(-30.,1.63388274786013,4.55655607176829));
#32826=CARTESIAN_POINT('Ctrl Pts',(-30.,1.50331560745686,4.61639586553387));
#32827=CARTESIAN_POINT('Ctrl Pts',(-30.,1.37011002491396,4.6704635809884));
#32828=CARTESIAN_POINT('Ctrl Pts',(-30.,1.23465431498687,4.71858368863437));
#32829=CARTESIAN_POINT('Ctrl Pts',(-30.,1.10035269443314,4.76629381057425));
#32830=CARTESIAN_POINT('Ctrl Pts',(-30.,0.96383842616513,4.80815761322486));
#32831=CARTESIAN_POINT('Ctrl Pts',(-30.,0.825466850475934,4.8439586961056));
#32832=CARTESIAN_POINT('Ctrl Pts',(-30.,0.782423564497787,4.85509534928808));
#32833=CARTESIAN_POINT('Ctrl Pts',(-30.,0.739200428308711,4.86564499042763));
#32834=CARTESIAN_POINT('Ctrl Pts',(-30.,0.695807839646249,4.87560011181053));
#32835=CARTESIAN_POINT('Ctrl Pts',(-30.,0.695807839646318,4.87560011181052));
#32836=CARTESIAN_POINT('Ctrl Pts',(-30.0396363329983,1.505295356838,4.76007633060594));
#32837=CARTESIAN_POINT('Ctrl Pts',(-30.0792726659966,2.28505096422592,4.43911803533769));
#32838=CARTESIAN_POINT('Ctrl Pts',(-30.118908998995,2.94077998825037,3.95114615387622));
#32839=CARTESIAN_POINT('Ctrl Pts',(-30.1585453319933,3.59650901227486,3.46317427241473));
#32840=CARTESIAN_POINT('Ctrl Pts',(-30.1981816649916,4.12821145293587,2.80818880476));
#32841=CARTESIAN_POINT('Ctrl Pts',(-30.2378179979899,4.47114017808342,2.06608473852283));
#32842=CARTESIAN_POINT('Ctrl Pts',(-30.2774543309882,4.81406890323096,1.32398067228571));
#32843=CARTESIAN_POINT('Ctrl Pts',(-30.3170906639866,4.96822391286505,0.494758007466152));
#32844=CARTESIAN_POINT('Ctrl Pts',(-30.3567269969849,4.91494372660875,-0.320960701335019));
#32845=CARTESIAN_POINT('Ctrl Pts',(-30.3963633299832,4.86166354035245,-1.13667941013621));
#32846=CARTESIAN_POINT('Ctrl Pts',(-30.4359996629815,4.60094815820575,-1.93889416291902));
#32847=CARTESIAN_POINT('Ctrl Pts',(-30.4756359959798,4.16444075576848,-2.63007230282805));
#32848=CARTESIAN_POINT('Ctrl Pts',(-30.5152723289782,3.72793335333121,-3.3212504427371));
#32849=CARTESIAN_POINT('Ctrl Pts',(-30.5549086619765,3.11563393060335,-3.90139196977236));
#32850=CARTESIAN_POINT('Ctrl Pts',(-30.5945449949748,2.40195440267049,-4.30004054600194));
#32851=CARTESIAN_POINT('Ctrl Pts',(-30.6341813279731,1.68827487473765,-4.69868912223151));
#32852=CARTESIAN_POINT('Ctrl Pts',(-30.6738176609715,0.873215241599798,
-4.91584474765542));
#32853=CARTESIAN_POINT('Ctrl Pts',(-30.7134539939698,0.0557974461108648,
-4.92510711469413));
#32854=CARTESIAN_POINT('Ctrl Pts',(-30.7530903269681,-0.761620349378092,
-4.93436948173283));
#32855=CARTESIAN_POINT('Ctrl Pts',(-30.7927266599664,-1.58139630721813,
-4.73573859038633));
#32856=CARTESIAN_POINT('Ctrl Pts',(-30.8323629929647,-2.30392266200803,
-4.35335613973094));
#32857=CARTESIAN_POINT('Ctrl Pts',(-30.8719993259631,-3.02644901679793,
-3.97097368907555));
#32858=CARTESIAN_POINT('Ctrl Pts',(-30.9116356589614,-3.65172576853768,
-3.40483967911129));
#32859=CARTESIAN_POINT('Ctrl Pts',(-30.9512719919597,-4.10378338287765,
-2.72373594332161));
#32860=CARTESIAN_POINT('Ctrl Pts',(-30.990908324958,-4.55584099721759,-2.04263220753197));
#32861=CARTESIAN_POINT('Ctrl Pts',(-31.0305446579563,-4.83467947415777,
-1.24655874591693));
#32862=CARTESIAN_POINT('Ctrl Pts',(-31.0701809909546,-4.90641862243869,
-0.432241158696399));
#32863=CARTESIAN_POINT('Ctrl Pts',(-31.0771734853352,-4.91907457603671,
-0.288582280038523));
#32864=CARTESIAN_POINT('Ctrl Pts',(-31.0841659797158,-4.92528503863494,
-0.144355594868911));
#32865=CARTESIAN_POINT('Ctrl Pts',(-31.0911584740964,-4.92514031288301,
-0.000116505347877993));
#32866=CARTESIAN_POINT('Origin',(-53.,4.5,0.));
#32867=CARTESIAN_POINT('',(-53.,-4.5,-5.51091059616309E-16));
#32868=CARTESIAN_POINT('Origin',(-53.,0.,0.));
#32869=CARTESIAN_POINT('Origin',(-52.75,0.,0.));
#32870=CARTESIAN_POINT('',(-52.75,-4.75,-5.81707229594993E-16));
#32871=CARTESIAN_POINT('Origin',(-41.25,0.,0.));
#32872=CARTESIAN_POINT('Origin',(-30.,0.,0.));
#32873=CARTESIAN_POINT('Origin',(-30.,8.,0.));
#32874=CARTESIAN_POINT('',(-30.,-8.,-9.79717439317883E-16));
#32875=CARTESIAN_POINT('Origin',(-30.,0.,0.));
#32876=CARTESIAN_POINT('Origin',(0.,0.,0.));
#32877=CARTESIAN_POINT('',(30.,-8.,-9.79717439317883E-16));
#32878=CARTESIAN_POINT('Origin',(30.,0.,0.));
#32879=CARTESIAN_POINT('',(0.,-8.,-9.79717439317883E-16));
#32880=CARTESIAN_POINT('Origin',(30.,5.,0.));
#32881=CARTESIAN_POINT('Origin',(52.75,0.,0.));
#32882=CARTESIAN_POINT('',(53.,-4.5,-5.51091059616309E-16));
#32883=CARTESIAN_POINT('Origin',(53.,0.,0.));
#32884=CARTESIAN_POINT('',(52.75,-4.75,-5.81707229594993E-16));
#32885=CARTESIAN_POINT('Origin',(53.,0.,0.));
#56604=UNCERTAINTY_MEASURE_WITH_UNIT(LENGTH_MEASURE(0.01),#56640,
'DISTANCE_ACCURACY_VALUE',
'Maximum model space distance between geometric entities at asserted c
onnectivities');
#56617=UNCERTAINTY_MEASURE_WITH_UNIT(LENGTH_MEASURE(0.01),#56640,
'DISTANCE_ACCURACY_VALUE',
'Maximum model space distance between geometric entities at asserted c
onnectivities');
#56626=(
GEOMETRIC_REPRESENTATION_CONTEXT(3)
GLOBAL_UNCERTAINTY_ASSIGNED_CONTEXT((#56604))
GLOBAL_UNIT_ASSIGNED_CONTEXT((#56640,#56642,#56643))
REPRESENTATION_CONTEXT('','3D')
);
#56639=(
GEOMETRIC_REPRESENTATION_CONTEXT(3)
GLOBAL_UNCERTAINTY_ASSIGNED_CONTEXT((#56617))
GLOBAL_UNIT_ASSIGNED_CONTEXT((#56640,#56642,#56643))
REPRESENTATION_CONTEXT('','3D')
);
#56640=(
LENGTH_UNIT()
NAMED_UNIT(*)
SI_UNIT(.MILLI.,.METRE.)
);
#56642=(
NAMED_UNIT(*)
PLANE_ANGLE_UNIT()
SI_UNIT($,.RADIAN.)
);
#56643=(
NAMED_UNIT(*)
SI_UNIT($,.STERADIAN.)
SOLID_ANGLE_UNIT()
);
#56652=SHAPE_DEFINITION_REPRESENTATION(#56673,#56752);
#56673=PRODUCT_DEFINITION_SHAPE('',$,#56774);
#56752=SHAPE_REPRESENTATION('',(#17684),#56626);
#56765=PRODUCT_DEFINITION_CONTEXT('part definition',#56830,'design');
#56774=PRODUCT_DEFINITION('2026-10-26-00-02-42-773',
'08_Center_Rod_D16_M10',#56795,#56765);
#56795=PRODUCT_DEFINITION_FORMATION('',$,#56840);
#56830=APPLICATION_CONTEXT(
'Core Data for Automotive Mechanical Design Process');
#56831=PRODUCT_CONTEXT('part definition',#56830,'mechanical');
#56840=PRODUCT('2026-10-26-00-02-42-773','08_Center_Rod_D16_M10',$,(#56831));
#56909=COLOUR_RGB('Grey',0.48,0.52,0.57);
#56910=FILL_AREA_STYLE_COLOUR('',#56909);
#56911=FILL_AREA_STYLE('',(#56910));
#56912=SURFACE_STYLE_FILL_AREA(#56911);
#56913=SURFACE_SIDE_STYLE('',(#56912));
#56914=SURFACE_STYLE_USAGE(.BOTH.,#56913);
#56915=PRESENTATION_STYLE_ASSIGNMENT((#56914));
ENDSEC;
END-ISO-10303-21;
